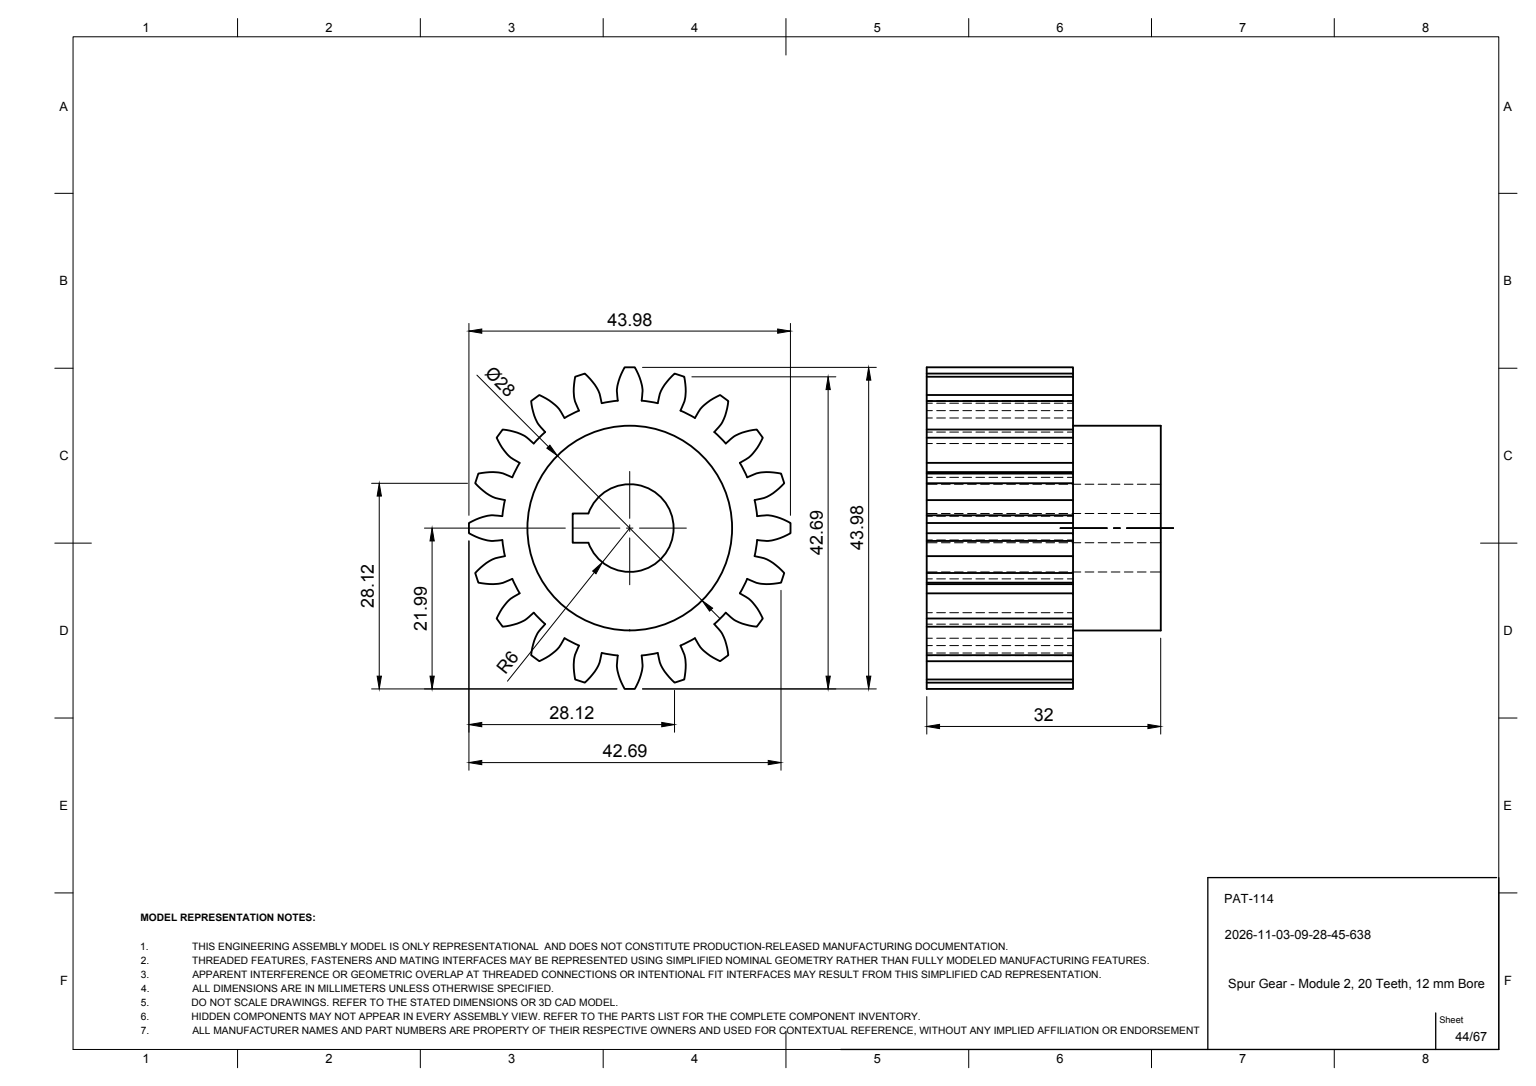
ISO-10303-21;
HEADER;
/* Generated by software containing ST-Developer
 * from STEP Tools, Inc. (www.steptools.com) 
 */

FILE_DESCRIPTION(
/* description */ ('Two-stage gear reducer in split housing'),
/* implementation_level */ '2;1');

FILE_NAME(
/* name */ 'Spur Gear - Module 2, 20 Teeth, 12 mm Bore.step',
/* time_stamp */ '2026-10-28T03:22:31-07:00',
/* author */ (''),
/* organization */ (''),
/* preprocessor_version */ 'ST-DEVELOPER v20.2',
/* originating_system */ 'Autodesk Translation Framework v15.17.0.0',
/* authorisation */ '');

FILE_SCHEMA (('AUTOMOTIVE_DESIGN { 1 0 10303 214 3 1 1 }'));
ENDSEC;

DATA;
#10=MECHANICAL_DESIGN_GEOMETRIC_PRESENTATION_REPRESENTATION('',(#1284),#73366);
#11=(
BOUNDED_SURFACE()
B_SPLINE_SURFACE(5,1,((#28644,#28645),(#28646,#28647),(#28648,#28649),(#28650,
#28651),(#28652,#28653),(#28654,#28655),(#28656,#28657),(#28658,#28659),
(#28660,#28661),(#28662,#28663),(#28664,#28665),(#28666,#28667),(#28668,
#28669),(#28670,#28671),(#28672,#28673),(#28674,#28675),(#28676,#28677),
(#28678,#28679),(#28680,#28681),(#28682,#28683),(#28684,#28685),(#28686,
#28687),(#28688,#28689),(#28690,#28691),(#28692,#28693),(#28694,#28695),
(#28696,#28697),(#28698,#28699),(#28700,#28701),(#28702,#28703),(#28704,
#28705),(#28706,#28707),(#28708,#28709),(#28710,#28711),(#28712,#28713),
(#28714,#28715),(#28716,#28717),(#28718,#28719),(#28720,#28721),(#28722,
#28723),(#28724,#28725),(#28726,#28727),(#28728,#28729),(#28730,#28731),
(#28732,#28733),(#28734,#28735),(#28736,#28737),(#28738,#28739),(#28740,
#28741),(#28742,#28743),(#28744,#28745),(#28746,#28747),(#28748,#28749),
(#28750,#28751),(#28752,#28753),(#28754,#28755),(#28756,#28757),(#28758,
#28759),(#28760,#28761),(#28762,#28763),(#28764,#28765),(#28766,#28767),
(#28768,#28769),(#28770,#28771),(#28772,#28773),(#28774,#28775),(#28776,
#28777),(#28778,#28779),(#28780,#28781),(#28782,#28783)),.UNSPECIFIED.,
 .F.,.F.,.F.)
B_SPLINE_SURFACE_WITH_KNOTS((6,1,1,1,1,1,1,1,1,1,1,1,1,1,1,1,1,1,1,1,1,
1,1,1,1,1,1,1,1,1,1,1,1,1,1,1,1,1,1,1,1,1,1,1,1,1,1,1,1,1,1,1,1,1,1,1,1,
1,1,1,1,1,1,1,1,6),(2,2),(-1.,-0.984615384615383,-0.969230769230768,-0.953846153846152,
-0.938461538461537,-0.923076923076922,-0.907692307692306,-0.892307692307691,
-0.876923076923076,-0.86153846153846,-0.846153846153845,-0.83076923076923,
-0.815384615384614,-0.799999999999999,-0.784615384615384,-0.769230769230768,
-0.753846153846153,-0.738461538461538,-0.723076923076922,-0.707692307692307,
-0.692307692307692,-0.676923076923076,-0.661538461538461,-0.646153846153846,
-0.63076923076923,-0.615384615384615,-0.6,-0.584615384615384,-0.569230769230769,
-0.553846153846154,-0.538461538461538,-0.523076923076923,-0.507692307692308,
-0.492307692307692,-0.476923076923077,-0.461538461538462,-0.446153846153846,
-0.430769230769231,-0.415384615384615,-0.4,-0.384615384615385,-0.369230769230769,
-0.353846153846154,-0.338461538461538,-0.323076923076923,-0.307692307692308,
-0.292307692307692,-0.276923076923077,-0.261538461538462,-0.246153846153846,
-0.230769230769231,-0.215384615384615,-0.2,-0.184615384615385,-0.169230769230769,
-0.153846153846154,-0.138461538461538,-0.123076923076923,-0.107692307692308,
-0.0923076923076923,-0.0769230769230769,-0.0615384615384615,-0.0461538461538462,
-0.0307692307692308,-0.0153846153846154,0.),(-1.,1.),.UNSPECIFIED.)
GEOMETRIC_REPRESENTATION_ITEM()
RATIONAL_B_SPLINE_SURFACE(((1.,1.),(1.,1.),(1.,1.),(1.,1.),(1.,1.),(1.,
1.),(1.,1.),(1.,1.),(1.,1.),(1.,1.),(1.,1.),(1.,1.),(1.,1.),(1.,1.),(1.,
1.),(1.,1.),(1.,1.),(1.,1.),(1.,1.),(1.,1.),(1.,1.),(1.,1.),(1.,1.),(1.,
1.),(1.,1.),(1.,1.),(1.,1.),(1.,1.),(1.,1.),(1.,1.),(1.,1.),(1.,1.),(1.,
1.),(1.,1.),(1.,1.),(1.,1.),(1.,1.),(1.,1.),(1.,1.),(1.,1.),(1.,1.),(1.,
1.),(1.,1.),(1.,1.),(1.,1.),(1.,1.),(1.,1.),(1.,1.),(1.,1.),(1.,1.),(1.,
1.),(1.,1.),(1.,1.),(1.,1.),(1.,1.),(1.,1.),(1.,1.),(1.,1.),(1.,1.),(1.,
1.),(1.,1.),(1.,1.),(1.,1.),(1.,1.),(1.,1.),(1.,1.),(1.,1.),(1.,1.),(1.,
1.),(1.,1.)))
REPRESENTATION_ITEM('')
SURFACE()
);
#12=(
BOUNDED_SURFACE()
B_SPLINE_SURFACE(5,1,((#28862,#28863),(#28864,#28865),(#28866,#28867),(#28868,
#28869),(#28870,#28871),(#28872,#28873),(#28874,#28875),(#28876,#28877),
(#28878,#28879),(#28880,#28881),(#28882,#28883),(#28884,#28885),(#28886,
#28887),(#28888,#28889),(#28890,#28891),(#28892,#28893),(#28894,#28895),
(#28896,#28897),(#28898,#28899),(#28900,#28901),(#28902,#28903),(#28904,
#28905),(#28906,#28907),(#28908,#28909),(#28910,#28911),(#28912,#28913),
(#28914,#28915),(#28916,#28917),(#28918,#28919),(#28920,#28921),(#28922,
#28923),(#28924,#28925),(#28926,#28927),(#28928,#28929),(#28930,#28931),
(#28932,#28933),(#28934,#28935),(#28936,#28937),(#28938,#28939),(#28940,
#28941),(#28942,#28943),(#28944,#28945),(#28946,#28947),(#28948,#28949),
(#28950,#28951),(#28952,#28953),(#28954,#28955),(#28956,#28957),(#28958,
#28959),(#28960,#28961),(#28962,#28963),(#28964,#28965),(#28966,#28967),
(#28968,#28969),(#28970,#28971),(#28972,#28973),(#28974,#28975),(#28976,
#28977),(#28978,#28979),(#28980,#28981),(#28982,#28983),(#28984,#28985),
(#28986,#28987),(#28988,#28989),(#28990,#28991),(#28992,#28993),(#28994,
#28995),(#28996,#28997),(#28998,#28999),(#29000,#29001)),.UNSPECIFIED.,
 .F.,.F.,.F.)
B_SPLINE_SURFACE_WITH_KNOTS((6,1,1,1,1,1,1,1,1,1,1,1,1,1,1,1,1,1,1,1,1,
1,1,1,1,1,1,1,1,1,1,1,1,1,1,1,1,1,1,1,1,1,1,1,1,1,1,1,1,1,1,1,1,1,1,1,1,
1,1,1,1,1,1,1,1,6),(2,2),(-1.,-0.984615384615383,-0.969230769230768,-0.953846153846152,
-0.938461538461537,-0.923076923076922,-0.907692307692306,-0.892307692307691,
-0.876923076923076,-0.86153846153846,-0.846153846153845,-0.83076923076923,
-0.815384615384614,-0.799999999999999,-0.784615384615384,-0.769230769230768,
-0.753846153846153,-0.738461538461538,-0.723076923076922,-0.707692307692307,
-0.692307692307692,-0.676923076923076,-0.661538461538461,-0.646153846153846,
-0.63076923076923,-0.615384615384615,-0.6,-0.584615384615384,-0.569230769230769,
-0.553846153846154,-0.538461538461538,-0.523076923076923,-0.507692307692308,
-0.492307692307692,-0.476923076923077,-0.461538461538462,-0.446153846153846,
-0.430769230769231,-0.415384615384615,-0.4,-0.384615384615385,-0.369230769230769,
-0.353846153846154,-0.338461538461538,-0.323076923076923,-0.307692307692308,
-0.292307692307692,-0.276923076923077,-0.261538461538462,-0.246153846153846,
-0.230769230769231,-0.215384615384615,-0.2,-0.184615384615385,-0.169230769230769,
-0.153846153846154,-0.138461538461538,-0.123076923076923,-0.107692307692308,
-0.0923076923076923,-0.0769230769230769,-0.0615384615384615,-0.0461538461538462,
-0.0307692307692308,-0.0153846153846154,0.),(-1.,1.),.UNSPECIFIED.)
GEOMETRIC_REPRESENTATION_ITEM()
RATIONAL_B_SPLINE_SURFACE(((1.,1.),(1.,1.),(1.,1.),(1.,1.),(1.,1.),(1.,
1.),(1.,1.),(1.,1.),(1.,1.),(1.,1.),(1.,1.),(1.,1.),(1.,1.),(1.,1.),(1.,
1.),(1.,1.),(1.,1.),(1.,1.),(1.,1.),(1.,1.),(1.,1.),(1.,1.),(1.,1.),(1.,
1.),(1.,1.),(1.,1.),(1.,1.),(1.,1.),(1.,1.),(1.,1.),(1.,1.),(1.,1.),(1.,
1.),(1.,1.),(1.,1.),(1.,1.),(1.,1.),(1.,1.),(1.,1.),(1.,1.),(1.,1.),(1.,
1.),(1.,1.),(1.,1.),(1.,1.),(1.,1.),(1.,1.),(1.,1.),(1.,1.),(1.,1.),(1.,
1.),(1.,1.),(1.,1.),(1.,1.),(1.,1.),(1.,1.),(1.,1.),(1.,1.),(1.,1.),(1.,
1.),(1.,1.),(1.,1.),(1.,1.),(1.,1.),(1.,1.),(1.,1.),(1.,1.),(1.,1.),(1.,
1.),(1.,1.)))
REPRESENTATION_ITEM('')
SURFACE()
);
#13=(
BOUNDED_SURFACE()
B_SPLINE_SURFACE(5,1,((#29078,#29079),(#29080,#29081),(#29082,#29083),(#29084,
#29085),(#29086,#29087),(#29088,#29089),(#29090,#29091),(#29092,#29093),
(#29094,#29095),(#29096,#29097),(#29098,#29099),(#29100,#29101),(#29102,
#29103),(#29104,#29105),(#29106,#29107),(#29108,#29109),(#29110,#29111),
(#29112,#29113),(#29114,#29115),(#29116,#29117),(#29118,#29119),(#29120,
#29121),(#29122,#29123),(#29124,#29125),(#29126,#29127),(#29128,#29129),
(#29130,#29131),(#29132,#29133),(#29134,#29135),(#29136,#29137),(#29138,
#29139),(#29140,#29141),(#29142,#29143),(#29144,#29145),(#29146,#29147),
(#29148,#29149),(#29150,#29151),(#29152,#29153),(#29154,#29155),(#29156,
#29157),(#29158,#29159),(#29160,#29161),(#29162,#29163),(#29164,#29165),
(#29166,#29167),(#29168,#29169),(#29170,#29171),(#29172,#29173),(#29174,
#29175),(#29176,#29177),(#29178,#29179),(#29180,#29181),(#29182,#29183),
(#29184,#29185),(#29186,#29187),(#29188,#29189),(#29190,#29191),(#29192,
#29193),(#29194,#29195),(#29196,#29197),(#29198,#29199),(#29200,#29201),
(#29202,#29203),(#29204,#29205),(#29206,#29207),(#29208,#29209),(#29210,
#29211),(#29212,#29213),(#29214,#29215),(#29216,#29217)),.UNSPECIFIED.,
 .F.,.F.,.F.)
B_SPLINE_SURFACE_WITH_KNOTS((6,1,1,1,1,1,1,1,1,1,1,1,1,1,1,1,1,1,1,1,1,
1,1,1,1,1,1,1,1,1,1,1,1,1,1,1,1,1,1,1,1,1,1,1,1,1,1,1,1,1,1,1,1,1,1,1,1,
1,1,1,1,1,1,1,1,6),(2,2),(-1.,-0.984615384615383,-0.969230769230768,-0.953846153846152,
-0.938461538461537,-0.923076923076922,-0.907692307692306,-0.892307692307691,
-0.876923076923076,-0.86153846153846,-0.846153846153845,-0.83076923076923,
-0.815384615384614,-0.799999999999999,-0.784615384615384,-0.769230769230768,
-0.753846153846153,-0.738461538461538,-0.723076923076922,-0.707692307692307,
-0.692307692307692,-0.676923076923076,-0.661538461538461,-0.646153846153846,
-0.63076923076923,-0.615384615384615,-0.6,-0.584615384615384,-0.569230769230769,
-0.553846153846154,-0.538461538461538,-0.523076923076923,-0.507692307692308,
-0.492307692307692,-0.476923076923077,-0.461538461538462,-0.446153846153846,
-0.430769230769231,-0.415384615384615,-0.4,-0.384615384615385,-0.369230769230769,
-0.353846153846154,-0.338461538461538,-0.323076923076923,-0.307692307692308,
-0.292307692307692,-0.276923076923077,-0.261538461538462,-0.246153846153846,
-0.230769230769231,-0.215384615384615,-0.2,-0.184615384615385,-0.169230769230769,
-0.153846153846154,-0.138461538461538,-0.123076923076923,-0.107692307692308,
-0.0923076923076923,-0.0769230769230769,-0.0615384615384615,-0.0461538461538462,
-0.0307692307692308,-0.0153846153846154,0.),(-1.,1.),.UNSPECIFIED.)
GEOMETRIC_REPRESENTATION_ITEM()
RATIONAL_B_SPLINE_SURFACE(((1.,1.),(1.,1.),(1.,1.),(1.,1.),(1.,1.),(1.,
1.),(1.,1.),(1.,1.),(1.,1.),(1.,1.),(1.,1.),(1.,1.),(1.,1.),(1.,1.),(1.,
1.),(1.,1.),(1.,1.),(1.,1.),(1.,1.),(1.,1.),(1.,1.),(1.,1.),(1.,1.),(1.,
1.),(1.,1.),(1.,1.),(1.,1.),(1.,1.),(1.,1.),(1.,1.),(1.,1.),(1.,1.),(1.,
1.),(1.,1.),(1.,1.),(1.,1.),(1.,1.),(1.,1.),(1.,1.),(1.,1.),(1.,1.),(1.,
1.),(1.,1.),(1.,1.),(1.,1.),(1.,1.),(1.,1.),(1.,1.),(1.,1.),(1.,1.),(1.,
1.),(1.,1.),(1.,1.),(1.,1.),(1.,1.),(1.,1.),(1.,1.),(1.,1.),(1.,1.),(1.,
1.),(1.,1.),(1.,1.),(1.,1.),(1.,1.),(1.,1.),(1.,1.),(1.,1.),(1.,1.),(1.,
1.),(1.,1.)))
REPRESENTATION_ITEM('')
SURFACE()
);
#14=(
BOUNDED_SURFACE()
B_SPLINE_SURFACE(5,1,((#29294,#29295),(#29296,#29297),(#29298,#29299),(#29300,
#29301),(#29302,#29303),(#29304,#29305),(#29306,#29307),(#29308,#29309),
(#29310,#29311),(#29312,#29313),(#29314,#29315),(#29316,#29317),(#29318,
#29319),(#29320,#29321),(#29322,#29323),(#29324,#29325),(#29326,#29327),
(#29328,#29329),(#29330,#29331),(#29332,#29333),(#29334,#29335),(#29336,
#29337),(#29338,#29339),(#29340,#29341),(#29342,#29343),(#29344,#29345),
(#29346,#29347),(#29348,#29349),(#29350,#29351),(#29352,#29353),(#29354,
#29355),(#29356,#29357),(#29358,#29359),(#29360,#29361),(#29362,#29363),
(#29364,#29365),(#29366,#29367),(#29368,#29369),(#29370,#29371),(#29372,
#29373),(#29374,#29375),(#29376,#29377),(#29378,#29379),(#29380,#29381),
(#29382,#29383),(#29384,#29385),(#29386,#29387),(#29388,#29389),(#29390,
#29391),(#29392,#29393),(#29394,#29395),(#29396,#29397),(#29398,#29399),
(#29400,#29401),(#29402,#29403),(#29404,#29405),(#29406,#29407),(#29408,
#29409),(#29410,#29411),(#29412,#29413),(#29414,#29415),(#29416,#29417),
(#29418,#29419),(#29420,#29421),(#29422,#29423),(#29424,#29425),(#29426,
#29427),(#29428,#29429),(#29430,#29431),(#29432,#29433)),.UNSPECIFIED.,
 .F.,.F.,.F.)
B_SPLINE_SURFACE_WITH_KNOTS((6,1,1,1,1,1,1,1,1,1,1,1,1,1,1,1,1,1,1,1,1,
1,1,1,1,1,1,1,1,1,1,1,1,1,1,1,1,1,1,1,1,1,1,1,1,1,1,1,1,1,1,1,1,1,1,1,1,
1,1,1,1,1,1,1,1,6),(2,2),(-1.,-0.984615384615383,-0.969230769230768,-0.953846153846152,
-0.938461538461537,-0.923076923076922,-0.907692307692306,-0.892307692307691,
-0.876923076923076,-0.86153846153846,-0.846153846153845,-0.83076923076923,
-0.815384615384614,-0.799999999999999,-0.784615384615384,-0.769230769230768,
-0.753846153846153,-0.738461538461538,-0.723076923076922,-0.707692307692307,
-0.692307692307692,-0.676923076923076,-0.661538461538461,-0.646153846153846,
-0.63076923076923,-0.615384615384615,-0.6,-0.584615384615384,-0.569230769230769,
-0.553846153846154,-0.538461538461538,-0.523076923076923,-0.507692307692308,
-0.492307692307692,-0.476923076923077,-0.461538461538462,-0.446153846153846,
-0.430769230769231,-0.415384615384615,-0.4,-0.384615384615385,-0.369230769230769,
-0.353846153846154,-0.338461538461538,-0.323076923076923,-0.307692307692308,
-0.292307692307692,-0.276923076923077,-0.261538461538462,-0.246153846153846,
-0.230769230769231,-0.215384615384615,-0.2,-0.184615384615385,-0.169230769230769,
-0.153846153846154,-0.138461538461538,-0.123076923076923,-0.107692307692308,
-0.0923076923076923,-0.0769230769230769,-0.0615384615384615,-0.0461538461538462,
-0.0307692307692308,-0.0153846153846154,0.),(-1.,1.),.UNSPECIFIED.)
GEOMETRIC_REPRESENTATION_ITEM()
RATIONAL_B_SPLINE_SURFACE(((1.,1.),(1.,1.),(1.,1.),(1.,1.),(1.,1.),(1.,
1.),(1.,1.),(1.,1.),(1.,1.),(1.,1.),(1.,1.),(1.,1.),(1.,1.),(1.,1.),(1.,
1.),(1.,1.),(1.,1.),(1.,1.),(1.,1.),(1.,1.),(1.,1.),(1.,1.),(1.,1.),(1.,
1.),(1.,1.),(1.,1.),(1.,1.),(1.,1.),(1.,1.),(1.,1.),(1.,1.),(1.,1.),(1.,
1.),(1.,1.),(1.,1.),(1.,1.),(1.,1.),(1.,1.),(1.,1.),(1.,1.),(1.,1.),(1.,
1.),(1.,1.),(1.,1.),(1.,1.),(1.,1.),(1.,1.),(1.,1.),(1.,1.),(1.,1.),(1.,
1.),(1.,1.),(1.,1.),(1.,1.),(1.,1.),(1.,1.),(1.,1.),(1.,1.),(1.,1.),(1.,
1.),(1.,1.),(1.,1.),(1.,1.),(1.,1.),(1.,1.),(1.,1.),(1.,1.),(1.,1.),(1.,
1.),(1.,1.)))
REPRESENTATION_ITEM('')
SURFACE()
);
#15=(
BOUNDED_SURFACE()
B_SPLINE_SURFACE(5,1,((#29510,#29511),(#29512,#29513),(#29514,#29515),(#29516,
#29517),(#29518,#29519),(#29520,#29521),(#29522,#29523),(#29524,#29525),
(#29526,#29527),(#29528,#29529),(#29530,#29531),(#29532,#29533),(#29534,
#29535),(#29536,#29537),(#29538,#29539),(#29540,#29541),(#29542,#29543),
(#29544,#29545),(#29546,#29547),(#29548,#29549),(#29550,#29551),(#29552,
#29553),(#29554,#29555),(#29556,#29557),(#29558,#29559),(#29560,#29561),
(#29562,#29563),(#29564,#29565),(#29566,#29567),(#29568,#29569),(#29570,
#29571),(#29572,#29573),(#29574,#29575),(#29576,#29577),(#29578,#29579),
(#29580,#29581),(#29582,#29583),(#29584,#29585),(#29586,#29587),(#29588,
#29589),(#29590,#29591),(#29592,#29593),(#29594,#29595),(#29596,#29597),
(#29598,#29599),(#29600,#29601),(#29602,#29603),(#29604,#29605),(#29606,
#29607),(#29608,#29609),(#29610,#29611),(#29612,#29613),(#29614,#29615),
(#29616,#29617),(#29618,#29619),(#29620,#29621),(#29622,#29623),(#29624,
#29625),(#29626,#29627),(#29628,#29629),(#29630,#29631),(#29632,#29633),
(#29634,#29635),(#29636,#29637),(#29638,#29639),(#29640,#29641),(#29642,
#29643),(#29644,#29645),(#29646,#29647),(#29648,#29649)),.UNSPECIFIED.,
 .F.,.F.,.F.)
B_SPLINE_SURFACE_WITH_KNOTS((6,1,1,1,1,1,1,1,1,1,1,1,1,1,1,1,1,1,1,1,1,
1,1,1,1,1,1,1,1,1,1,1,1,1,1,1,1,1,1,1,1,1,1,1,1,1,1,1,1,1,1,1,1,1,1,1,1,
1,1,1,1,1,1,1,1,6),(2,2),(-1.,-0.984615384615383,-0.969230769230768,-0.953846153846152,
-0.938461538461537,-0.923076923076922,-0.907692307692306,-0.892307692307691,
-0.876923076923076,-0.86153846153846,-0.846153846153845,-0.83076923076923,
-0.815384615384614,-0.799999999999999,-0.784615384615384,-0.769230769230768,
-0.753846153846153,-0.738461538461538,-0.723076923076922,-0.707692307692307,
-0.692307692307692,-0.676923076923076,-0.661538461538461,-0.646153846153846,
-0.63076923076923,-0.615384615384615,-0.6,-0.584615384615384,-0.569230769230769,
-0.553846153846154,-0.538461538461538,-0.523076923076923,-0.507692307692308,
-0.492307692307692,-0.476923076923077,-0.461538461538462,-0.446153846153846,
-0.430769230769231,-0.415384615384615,-0.4,-0.384615384615385,-0.369230769230769,
-0.353846153846154,-0.338461538461538,-0.323076923076923,-0.307692307692308,
-0.292307692307692,-0.276923076923077,-0.261538461538462,-0.246153846153846,
-0.230769230769231,-0.215384615384615,-0.2,-0.184615384615385,-0.169230769230769,
-0.153846153846154,-0.138461538461538,-0.123076923076923,-0.107692307692308,
-0.0923076923076923,-0.0769230769230769,-0.0615384615384615,-0.0461538461538462,
-0.0307692307692308,-0.0153846153846154,0.),(-1.,1.),.UNSPECIFIED.)
GEOMETRIC_REPRESENTATION_ITEM()
RATIONAL_B_SPLINE_SURFACE(((1.,1.),(1.,1.),(1.,1.),(1.,1.),(1.,1.),(1.,
1.),(1.,1.),(1.,1.),(1.,1.),(1.,1.),(1.,1.),(1.,1.),(1.,1.),(1.,1.),(1.,
1.),(1.,1.),(1.,1.),(1.,1.),(1.,1.),(1.,1.),(1.,1.),(1.,1.),(1.,1.),(1.,
1.),(1.,1.),(1.,1.),(1.,1.),(1.,1.),(1.,1.),(1.,1.),(1.,1.),(1.,1.),(1.,
1.),(1.,1.),(1.,1.),(1.,1.),(1.,1.),(1.,1.),(1.,1.),(1.,1.),(1.,1.),(1.,
1.),(1.,1.),(1.,1.),(1.,1.),(1.,1.),(1.,1.),(1.,1.),(1.,1.),(1.,1.),(1.,
1.),(1.,1.),(1.,1.),(1.,1.),(1.,1.),(1.,1.),(1.,1.),(1.,1.),(1.,1.),(1.,
1.),(1.,1.),(1.,1.),(1.,1.),(1.,1.),(1.,1.),(1.,1.),(1.,1.),(1.,1.),(1.,
1.),(1.,1.)))
REPRESENTATION_ITEM('')
SURFACE()
);
#16=(
BOUNDED_SURFACE()
B_SPLINE_SURFACE(5,1,((#29726,#29727),(#29728,#29729),(#29730,#29731),(#29732,
#29733),(#29734,#29735),(#29736,#29737),(#29738,#29739),(#29740,#29741),
(#29742,#29743),(#29744,#29745),(#29746,#29747),(#29748,#29749),(#29750,
#29751),(#29752,#29753),(#29754,#29755),(#29756,#29757),(#29758,#29759),
(#29760,#29761),(#29762,#29763),(#29764,#29765),(#29766,#29767),(#29768,
#29769),(#29770,#29771),(#29772,#29773),(#29774,#29775),(#29776,#29777),
(#29778,#29779),(#29780,#29781),(#29782,#29783),(#29784,#29785),(#29786,
#29787),(#29788,#29789),(#29790,#29791),(#29792,#29793),(#29794,#29795),
(#29796,#29797),(#29798,#29799),(#29800,#29801),(#29802,#29803),(#29804,
#29805),(#29806,#29807),(#29808,#29809),(#29810,#29811),(#29812,#29813),
(#29814,#29815),(#29816,#29817),(#29818,#29819),(#29820,#29821),(#29822,
#29823),(#29824,#29825),(#29826,#29827),(#29828,#29829),(#29830,#29831),
(#29832,#29833),(#29834,#29835),(#29836,#29837),(#29838,#29839),(#29840,
#29841),(#29842,#29843),(#29844,#29845),(#29846,#29847),(#29848,#29849),
(#29850,#29851),(#29852,#29853),(#29854,#29855),(#29856,#29857),(#29858,
#29859),(#29860,#29861),(#29862,#29863),(#29864,#29865)),.UNSPECIFIED.,
 .F.,.F.,.F.)
B_SPLINE_SURFACE_WITH_KNOTS((6,1,1,1,1,1,1,1,1,1,1,1,1,1,1,1,1,1,1,1,1,
1,1,1,1,1,1,1,1,1,1,1,1,1,1,1,1,1,1,1,1,1,1,1,1,1,1,1,1,1,1,1,1,1,1,1,1,
1,1,1,1,1,1,1,1,6),(2,2),(-1.,-0.984615384615383,-0.969230769230768,-0.953846153846152,
-0.938461538461537,-0.923076923076922,-0.907692307692306,-0.892307692307691,
-0.876923076923076,-0.86153846153846,-0.846153846153845,-0.83076923076923,
-0.815384615384614,-0.799999999999999,-0.784615384615384,-0.769230769230768,
-0.753846153846153,-0.738461538461538,-0.723076923076922,-0.707692307692307,
-0.692307692307692,-0.676923076923076,-0.661538461538461,-0.646153846153846,
-0.63076923076923,-0.615384615384615,-0.6,-0.584615384615384,-0.569230769230769,
-0.553846153846154,-0.538461538461538,-0.523076923076923,-0.507692307692308,
-0.492307692307692,-0.476923076923077,-0.461538461538462,-0.446153846153846,
-0.430769230769231,-0.415384615384615,-0.4,-0.384615384615385,-0.369230769230769,
-0.353846153846154,-0.338461538461538,-0.323076923076923,-0.307692307692308,
-0.292307692307692,-0.276923076923077,-0.261538461538462,-0.246153846153846,
-0.230769230769231,-0.215384615384615,-0.2,-0.184615384615385,-0.169230769230769,
-0.153846153846154,-0.138461538461538,-0.123076923076923,-0.107692307692308,
-0.0923076923076923,-0.0769230769230769,-0.0615384615384615,-0.0461538461538462,
-0.0307692307692308,-0.0153846153846154,0.),(-1.,1.),.UNSPECIFIED.)
GEOMETRIC_REPRESENTATION_ITEM()
RATIONAL_B_SPLINE_SURFACE(((1.,1.),(1.,1.),(1.,1.),(1.,1.),(1.,1.),(1.,
1.),(1.,1.),(1.,1.),(1.,1.),(1.,1.),(1.,1.),(1.,1.),(1.,1.),(1.,1.),(1.,
1.),(1.,1.),(1.,1.),(1.,1.),(1.,1.),(1.,1.),(1.,1.),(1.,1.),(1.,1.),(1.,
1.),(1.,1.),(1.,1.),(1.,1.),(1.,1.),(1.,1.),(1.,1.),(1.,1.),(1.,1.),(1.,
1.),(1.,1.),(1.,1.),(1.,1.),(1.,1.),(1.,1.),(1.,1.),(1.,1.),(1.,1.),(1.,
1.),(1.,1.),(1.,1.),(1.,1.),(1.,1.),(1.,1.),(1.,1.),(1.,1.),(1.,1.),(1.,
1.),(1.,1.),(1.,1.),(1.,1.),(1.,1.),(1.,1.),(1.,1.),(1.,1.),(1.,1.),(1.,
1.),(1.,1.),(1.,1.),(1.,1.),(1.,1.),(1.,1.),(1.,1.),(1.,1.),(1.,1.),(1.,
1.),(1.,1.)))
REPRESENTATION_ITEM('')
SURFACE()
);
#17=(
BOUNDED_SURFACE()
B_SPLINE_SURFACE(5,1,((#29942,#29943),(#29944,#29945),(#29946,#29947),(#29948,
#29949),(#29950,#29951),(#29952,#29953),(#29954,#29955),(#29956,#29957),
(#29958,#29959),(#29960,#29961),(#29962,#29963),(#29964,#29965),(#29966,
#29967),(#29968,#29969),(#29970,#29971),(#29972,#29973),(#29974,#29975),
(#29976,#29977),(#29978,#29979),(#29980,#29981),(#29982,#29983),(#29984,
#29985),(#29986,#29987),(#29988,#29989),(#29990,#29991),(#29992,#29993),
(#29994,#29995),(#29996,#29997),(#29998,#29999),(#30000,#30001),(#30002,
#30003),(#30004,#30005),(#30006,#30007),(#30008,#30009),(#30010,#30011),
(#30012,#30013),(#30014,#30015),(#30016,#30017),(#30018,#30019),(#30020,
#30021),(#30022,#30023),(#30024,#30025),(#30026,#30027),(#30028,#30029),
(#30030,#30031),(#30032,#30033),(#30034,#30035),(#30036,#30037),(#30038,
#30039),(#30040,#30041),(#30042,#30043),(#30044,#30045),(#30046,#30047),
(#30048,#30049),(#30050,#30051),(#30052,#30053),(#30054,#30055),(#30056,
#30057),(#30058,#30059),(#30060,#30061),(#30062,#30063),(#30064,#30065),
(#30066,#30067),(#30068,#30069),(#30070,#30071),(#30072,#30073),(#30074,
#30075),(#30076,#30077),(#30078,#30079),(#30080,#30081)),.UNSPECIFIED.,
 .F.,.F.,.F.)
B_SPLINE_SURFACE_WITH_KNOTS((6,1,1,1,1,1,1,1,1,1,1,1,1,1,1,1,1,1,1,1,1,
1,1,1,1,1,1,1,1,1,1,1,1,1,1,1,1,1,1,1,1,1,1,1,1,1,1,1,1,1,1,1,1,1,1,1,1,
1,1,1,1,1,1,1,1,6),(2,2),(-1.,-0.984615384615383,-0.969230769230768,-0.953846153846152,
-0.938461538461537,-0.923076923076922,-0.907692307692306,-0.892307692307691,
-0.876923076923076,-0.86153846153846,-0.846153846153845,-0.83076923076923,
-0.815384615384614,-0.799999999999999,-0.784615384615384,-0.769230769230768,
-0.753846153846153,-0.738461538461538,-0.723076923076922,-0.707692307692307,
-0.692307692307692,-0.676923076923076,-0.661538461538461,-0.646153846153846,
-0.63076923076923,-0.615384615384615,-0.6,-0.584615384615384,-0.569230769230769,
-0.553846153846154,-0.538461538461538,-0.523076923076923,-0.507692307692308,
-0.492307692307692,-0.476923076923077,-0.461538461538462,-0.446153846153846,
-0.430769230769231,-0.415384615384615,-0.4,-0.384615384615385,-0.369230769230769,
-0.353846153846154,-0.338461538461538,-0.323076923076923,-0.307692307692308,
-0.292307692307692,-0.276923076923077,-0.261538461538462,-0.246153846153846,
-0.230769230769231,-0.215384615384615,-0.2,-0.184615384615385,-0.169230769230769,
-0.153846153846154,-0.138461538461538,-0.123076923076923,-0.107692307692308,
-0.0923076923076923,-0.0769230769230769,-0.0615384615384615,-0.0461538461538462,
-0.0307692307692308,-0.0153846153846154,0.),(-1.,1.),.UNSPECIFIED.)
GEOMETRIC_REPRESENTATION_ITEM()
RATIONAL_B_SPLINE_SURFACE(((1.,1.),(1.,1.),(1.,1.),(1.,1.),(1.,1.),(1.,
1.),(1.,1.),(1.,1.),(1.,1.),(1.,1.),(1.,1.),(1.,1.),(1.,1.),(1.,1.),(1.,
1.),(1.,1.),(1.,1.),(1.,1.),(1.,1.),(1.,1.),(1.,1.),(1.,1.),(1.,1.),(1.,
1.),(1.,1.),(1.,1.),(1.,1.),(1.,1.),(1.,1.),(1.,1.),(1.,1.),(1.,1.),(1.,
1.),(1.,1.),(1.,1.),(1.,1.),(1.,1.),(1.,1.),(1.,1.),(1.,1.),(1.,1.),(1.,
1.),(1.,1.),(1.,1.),(1.,1.),(1.,1.),(1.,1.),(1.,1.),(1.,1.),(1.,1.),(1.,
1.),(1.,1.),(1.,1.),(1.,1.),(1.,1.),(1.,1.),(1.,1.),(1.,1.),(1.,1.),(1.,
1.),(1.,1.),(1.,1.),(1.,1.),(1.,1.),(1.,1.),(1.,1.),(1.,1.),(1.,1.),(1.,
1.),(1.,1.)))
REPRESENTATION_ITEM('')
SURFACE()
);
#18=(
BOUNDED_SURFACE()
B_SPLINE_SURFACE(5,1,((#30158,#30159),(#30160,#30161),(#30162,#30163),(#30164,
#30165),(#30166,#30167),(#30168,#30169),(#30170,#30171),(#30172,#30173),
(#30174,#30175),(#30176,#30177),(#30178,#30179),(#30180,#30181),(#30182,
#30183),(#30184,#30185),(#30186,#30187),(#30188,#30189),(#30190,#30191),
(#30192,#30193),(#30194,#30195),(#30196,#30197),(#30198,#30199),(#30200,
#30201),(#30202,#30203),(#30204,#30205),(#30206,#30207),(#30208,#30209),
(#30210,#30211),(#30212,#30213),(#30214,#30215),(#30216,#30217),(#30218,
#30219),(#30220,#30221),(#30222,#30223),(#30224,#30225),(#30226,#30227),
(#30228,#30229),(#30230,#30231),(#30232,#30233),(#30234,#30235),(#30236,
#30237),(#30238,#30239),(#30240,#30241),(#30242,#30243),(#30244,#30245),
(#30246,#30247),(#30248,#30249),(#30250,#30251),(#30252,#30253),(#30254,
#30255),(#30256,#30257),(#30258,#30259),(#30260,#30261),(#30262,#30263),
(#30264,#30265),(#30266,#30267),(#30268,#30269),(#30270,#30271),(#30272,
#30273),(#30274,#30275),(#30276,#30277),(#30278,#30279),(#30280,#30281),
(#30282,#30283),(#30284,#30285),(#30286,#30287),(#30288,#30289),(#30290,
#30291),(#30292,#30293),(#30294,#30295),(#30296,#30297)),.UNSPECIFIED.,
 .F.,.F.,.F.)
B_SPLINE_SURFACE_WITH_KNOTS((6,1,1,1,1,1,1,1,1,1,1,1,1,1,1,1,1,1,1,1,1,
1,1,1,1,1,1,1,1,1,1,1,1,1,1,1,1,1,1,1,1,1,1,1,1,1,1,1,1,1,1,1,1,1,1,1,1,
1,1,1,1,1,1,1,1,6),(2,2),(-1.,-0.984615384615383,-0.969230769230768,-0.953846153846152,
-0.938461538461537,-0.923076923076922,-0.907692307692306,-0.892307692307691,
-0.876923076923076,-0.86153846153846,-0.846153846153845,-0.83076923076923,
-0.815384615384614,-0.799999999999999,-0.784615384615384,-0.769230769230768,
-0.753846153846153,-0.738461538461538,-0.723076923076922,-0.707692307692307,
-0.692307692307692,-0.676923076923076,-0.661538461538461,-0.646153846153846,
-0.63076923076923,-0.615384615384615,-0.6,-0.584615384615384,-0.569230769230769,
-0.553846153846154,-0.538461538461538,-0.523076923076923,-0.507692307692308,
-0.492307692307692,-0.476923076923077,-0.461538461538462,-0.446153846153846,
-0.430769230769231,-0.415384615384615,-0.4,-0.384615384615385,-0.369230769230769,
-0.353846153846154,-0.338461538461538,-0.323076923076923,-0.307692307692308,
-0.292307692307692,-0.276923076923077,-0.261538461538462,-0.246153846153846,
-0.230769230769231,-0.215384615384615,-0.2,-0.184615384615385,-0.169230769230769,
-0.153846153846154,-0.138461538461538,-0.123076923076923,-0.107692307692308,
-0.0923076923076923,-0.0769230769230769,-0.0615384615384615,-0.0461538461538462,
-0.0307692307692308,-0.0153846153846154,0.),(-1.,1.),.UNSPECIFIED.)
GEOMETRIC_REPRESENTATION_ITEM()
RATIONAL_B_SPLINE_SURFACE(((1.,1.),(1.,1.),(1.,1.),(1.,1.),(1.,1.),(1.,
1.),(1.,1.),(1.,1.),(1.,1.),(1.,1.),(1.,1.),(1.,1.),(1.,1.),(1.,1.),(1.,
1.),(1.,1.),(1.,1.),(1.,1.),(1.,1.),(1.,1.),(1.,1.),(1.,1.),(1.,1.),(1.,
1.),(1.,1.),(1.,1.),(1.,1.),(1.,1.),(1.,1.),(1.,1.),(1.,1.),(1.,1.),(1.,
1.),(1.,1.),(1.,1.),(1.,1.),(1.,1.),(1.,1.),(1.,1.),(1.,1.),(1.,1.),(1.,
1.),(1.,1.),(1.,1.),(1.,1.),(1.,1.),(1.,1.),(1.,1.),(1.,1.),(1.,1.),(1.,
1.),(1.,1.),(1.,1.),(1.,1.),(1.,1.),(1.,1.),(1.,1.),(1.,1.),(1.,1.),(1.,
1.),(1.,1.),(1.,1.),(1.,1.),(1.,1.),(1.,1.),(1.,1.),(1.,1.),(1.,1.),(1.,
1.),(1.,1.)))
REPRESENTATION_ITEM('')
SURFACE()
);
#19=(
BOUNDED_SURFACE()
B_SPLINE_SURFACE(5,1,((#30374,#30375),(#30376,#30377),(#30378,#30379),(#30380,
#30381),(#30382,#30383),(#30384,#30385),(#30386,#30387),(#30388,#30389),
(#30390,#30391),(#30392,#30393),(#30394,#30395),(#30396,#30397),(#30398,
#30399),(#30400,#30401),(#30402,#30403),(#30404,#30405),(#30406,#30407),
(#30408,#30409),(#30410,#30411),(#30412,#30413),(#30414,#30415),(#30416,
#30417),(#30418,#30419),(#30420,#30421),(#30422,#30423),(#30424,#30425),
(#30426,#30427),(#30428,#30429),(#30430,#30431),(#30432,#30433),(#30434,
#30435),(#30436,#30437),(#30438,#30439),(#30440,#30441),(#30442,#30443),
(#30444,#30445),(#30446,#30447),(#30448,#30449),(#30450,#30451),(#30452,
#30453),(#30454,#30455),(#30456,#30457),(#30458,#30459),(#30460,#30461),
(#30462,#30463),(#30464,#30465),(#30466,#30467),(#30468,#30469),(#30470,
#30471),(#30472,#30473),(#30474,#30475),(#30476,#30477),(#30478,#30479),
(#30480,#30481),(#30482,#30483),(#30484,#30485),(#30486,#30487),(#30488,
#30489),(#30490,#30491),(#30492,#30493),(#30494,#30495),(#30496,#30497),
(#30498,#30499),(#30500,#30501),(#30502,#30503),(#30504,#30505),(#30506,
#30507),(#30508,#30509),(#30510,#30511),(#30512,#30513)),.UNSPECIFIED.,
 .F.,.F.,.F.)
B_SPLINE_SURFACE_WITH_KNOTS((6,1,1,1,1,1,1,1,1,1,1,1,1,1,1,1,1,1,1,1,1,
1,1,1,1,1,1,1,1,1,1,1,1,1,1,1,1,1,1,1,1,1,1,1,1,1,1,1,1,1,1,1,1,1,1,1,1,
1,1,1,1,1,1,1,1,6),(2,2),(-1.,-0.984615384615383,-0.969230769230768,-0.953846153846152,
-0.938461538461537,-0.923076923076922,-0.907692307692306,-0.892307692307691,
-0.876923076923076,-0.86153846153846,-0.846153846153845,-0.83076923076923,
-0.815384615384614,-0.799999999999999,-0.784615384615384,-0.769230769230768,
-0.753846153846153,-0.738461538461538,-0.723076923076922,-0.707692307692307,
-0.692307692307692,-0.676923076923076,-0.661538461538461,-0.646153846153846,
-0.63076923076923,-0.615384615384615,-0.6,-0.584615384615384,-0.569230769230769,
-0.553846153846154,-0.538461538461538,-0.523076923076923,-0.507692307692308,
-0.492307692307692,-0.476923076923077,-0.461538461538462,-0.446153846153846,
-0.430769230769231,-0.415384615384615,-0.4,-0.384615384615385,-0.369230769230769,
-0.353846153846154,-0.338461538461538,-0.323076923076923,-0.307692307692308,
-0.292307692307692,-0.276923076923077,-0.261538461538462,-0.246153846153846,
-0.230769230769231,-0.215384615384615,-0.2,-0.184615384615385,-0.169230769230769,
-0.153846153846154,-0.138461538461538,-0.123076923076923,-0.107692307692308,
-0.0923076923076923,-0.0769230769230769,-0.0615384615384615,-0.0461538461538462,
-0.0307692307692308,-0.0153846153846154,0.),(-1.,1.),.UNSPECIFIED.)
GEOMETRIC_REPRESENTATION_ITEM()
RATIONAL_B_SPLINE_SURFACE(((1.,1.),(1.,1.),(1.,1.),(1.,1.),(1.,1.),(1.,
1.),(1.,1.),(1.,1.),(1.,1.),(1.,1.),(1.,1.),(1.,1.),(1.,1.),(1.,1.),(1.,
1.),(1.,1.),(1.,1.),(1.,1.),(1.,1.),(1.,1.),(1.,1.),(1.,1.),(1.,1.),(1.,
1.),(1.,1.),(1.,1.),(1.,1.),(1.,1.),(1.,1.),(1.,1.),(1.,1.),(1.,1.),(1.,
1.),(1.,1.),(1.,1.),(1.,1.),(1.,1.),(1.,1.),(1.,1.),(1.,1.),(1.,1.),(1.,
1.),(1.,1.),(1.,1.),(1.,1.),(1.,1.),(1.,1.),(1.,1.),(1.,1.),(1.,1.),(1.,
1.),(1.,1.),(1.,1.),(1.,1.),(1.,1.),(1.,1.),(1.,1.),(1.,1.),(1.,1.),(1.,
1.),(1.,1.),(1.,1.),(1.,1.),(1.,1.),(1.,1.),(1.,1.),(1.,1.),(1.,1.),(1.,
1.),(1.,1.)))
REPRESENTATION_ITEM('')
SURFACE()
);
#20=(
BOUNDED_SURFACE()
B_SPLINE_SURFACE(5,1,((#30590,#30591),(#30592,#30593),(#30594,#30595),(#30596,
#30597),(#30598,#30599),(#30600,#30601),(#30602,#30603),(#30604,#30605),
(#30606,#30607),(#30608,#30609),(#30610,#30611),(#30612,#30613),(#30614,
#30615),(#30616,#30617),(#30618,#30619),(#30620,#30621),(#30622,#30623),
(#30624,#30625),(#30626,#30627),(#30628,#30629),(#30630,#30631),(#30632,
#30633),(#30634,#30635),(#30636,#30637),(#30638,#30639),(#30640,#30641),
(#30642,#30643),(#30644,#30645),(#30646,#30647),(#30648,#30649),(#30650,
#30651),(#30652,#30653),(#30654,#30655),(#30656,#30657),(#30658,#30659),
(#30660,#30661),(#30662,#30663),(#30664,#30665),(#30666,#30667),(#30668,
#30669),(#30670,#30671),(#30672,#30673),(#30674,#30675),(#30676,#30677),
(#30678,#30679),(#30680,#30681),(#30682,#30683),(#30684,#30685),(#30686,
#30687),(#30688,#30689),(#30690,#30691),(#30692,#30693),(#30694,#30695),
(#30696,#30697),(#30698,#30699),(#30700,#30701),(#30702,#30703),(#30704,
#30705),(#30706,#30707),(#30708,#30709),(#30710,#30711),(#30712,#30713),
(#30714,#30715),(#30716,#30717),(#30718,#30719),(#30720,#30721),(#30722,
#30723),(#30724,#30725),(#30726,#30727),(#30728,#30729)),.UNSPECIFIED.,
 .F.,.F.,.F.)
B_SPLINE_SURFACE_WITH_KNOTS((6,1,1,1,1,1,1,1,1,1,1,1,1,1,1,1,1,1,1,1,1,
1,1,1,1,1,1,1,1,1,1,1,1,1,1,1,1,1,1,1,1,1,1,1,1,1,1,1,1,1,1,1,1,1,1,1,1,
1,1,1,1,1,1,1,1,6),(2,2),(-1.,-0.984615384615383,-0.969230769230768,-0.953846153846152,
-0.938461538461537,-0.923076923076922,-0.907692307692306,-0.892307692307691,
-0.876923076923076,-0.86153846153846,-0.846153846153845,-0.83076923076923,
-0.815384615384614,-0.799999999999999,-0.784615384615384,-0.769230769230768,
-0.753846153846153,-0.738461538461538,-0.723076923076922,-0.707692307692307,
-0.692307692307692,-0.676923076923076,-0.661538461538461,-0.646153846153846,
-0.63076923076923,-0.615384615384615,-0.6,-0.584615384615384,-0.569230769230769,
-0.553846153846154,-0.538461538461538,-0.523076923076923,-0.507692307692308,
-0.492307692307692,-0.476923076923077,-0.461538461538462,-0.446153846153846,
-0.430769230769231,-0.415384615384615,-0.4,-0.384615384615385,-0.369230769230769,
-0.353846153846154,-0.338461538461538,-0.323076923076923,-0.307692307692308,
-0.292307692307692,-0.276923076923077,-0.261538461538462,-0.246153846153846,
-0.230769230769231,-0.215384615384615,-0.2,-0.184615384615385,-0.169230769230769,
-0.153846153846154,-0.138461538461538,-0.123076923076923,-0.107692307692308,
-0.0923076923076923,-0.0769230769230769,-0.0615384615384615,-0.0461538461538462,
-0.0307692307692308,-0.0153846153846154,0.),(-1.,1.),.UNSPECIFIED.)
GEOMETRIC_REPRESENTATION_ITEM()
RATIONAL_B_SPLINE_SURFACE(((1.,1.),(1.,1.),(1.,1.),(1.,1.),(1.,1.),(1.,
1.),(1.,1.),(1.,1.),(1.,1.),(1.,1.),(1.,1.),(1.,1.),(1.,1.),(1.,1.),(1.,
1.),(1.,1.),(1.,1.),(1.,1.),(1.,1.),(1.,1.),(1.,1.),(1.,1.),(1.,1.),(1.,
1.),(1.,1.),(1.,1.),(1.,1.),(1.,1.),(1.,1.),(1.,1.),(1.,1.),(1.,1.),(1.,
1.),(1.,1.),(1.,1.),(1.,1.),(1.,1.),(1.,1.),(1.,1.),(1.,1.),(1.,1.),(1.,
1.),(1.,1.),(1.,1.),(1.,1.),(1.,1.),(1.,1.),(1.,1.),(1.,1.),(1.,1.),(1.,
1.),(1.,1.),(1.,1.),(1.,1.),(1.,1.),(1.,1.),(1.,1.),(1.,1.),(1.,1.),(1.,
1.),(1.,1.),(1.,1.),(1.,1.),(1.,1.),(1.,1.),(1.,1.),(1.,1.),(1.,1.),(1.,
1.),(1.,1.)))
REPRESENTATION_ITEM('')
SURFACE()
);
#21=(
BOUNDED_SURFACE()
B_SPLINE_SURFACE(5,1,((#30806,#30807),(#30808,#30809),(#30810,#30811),(#30812,
#30813),(#30814,#30815),(#30816,#30817),(#30818,#30819),(#30820,#30821),
(#30822,#30823),(#30824,#30825),(#30826,#30827),(#30828,#30829),(#30830,
#30831),(#30832,#30833),(#30834,#30835),(#30836,#30837),(#30838,#30839),
(#30840,#30841),(#30842,#30843),(#30844,#30845),(#30846,#30847),(#30848,
#30849),(#30850,#30851),(#30852,#30853),(#30854,#30855),(#30856,#30857),
(#30858,#30859),(#30860,#30861),(#30862,#30863),(#30864,#30865),(#30866,
#30867),(#30868,#30869),(#30870,#30871),(#30872,#30873),(#30874,#30875),
(#30876,#30877),(#30878,#30879),(#30880,#30881),(#30882,#30883),(#30884,
#30885),(#30886,#30887),(#30888,#30889),(#30890,#30891),(#30892,#30893),
(#30894,#30895),(#30896,#30897),(#30898,#30899),(#30900,#30901),(#30902,
#30903),(#30904,#30905),(#30906,#30907),(#30908,#30909),(#30910,#30911),
(#30912,#30913),(#30914,#30915),(#30916,#30917),(#30918,#30919),(#30920,
#30921),(#30922,#30923),(#30924,#30925),(#30926,#30927),(#30928,#30929),
(#30930,#30931),(#30932,#30933),(#30934,#30935),(#30936,#30937),(#30938,
#30939),(#30940,#30941),(#30942,#30943),(#30944,#30945)),.UNSPECIFIED.,
 .F.,.F.,.F.)
B_SPLINE_SURFACE_WITH_KNOTS((6,1,1,1,1,1,1,1,1,1,1,1,1,1,1,1,1,1,1,1,1,
1,1,1,1,1,1,1,1,1,1,1,1,1,1,1,1,1,1,1,1,1,1,1,1,1,1,1,1,1,1,1,1,1,1,1,1,
1,1,1,1,1,1,1,1,6),(2,2),(-1.,-0.984615384615383,-0.969230769230768,-0.953846153846152,
-0.938461538461537,-0.923076923076922,-0.907692307692306,-0.892307692307691,
-0.876923076923076,-0.86153846153846,-0.846153846153845,-0.83076923076923,
-0.815384615384614,-0.799999999999999,-0.784615384615384,-0.769230769230768,
-0.753846153846153,-0.738461538461538,-0.723076923076922,-0.707692307692307,
-0.692307692307692,-0.676923076923076,-0.661538461538461,-0.646153846153846,
-0.63076923076923,-0.615384615384615,-0.6,-0.584615384615384,-0.569230769230769,
-0.553846153846154,-0.538461538461538,-0.523076923076923,-0.507692307692308,
-0.492307692307692,-0.476923076923077,-0.461538461538462,-0.446153846153846,
-0.430769230769231,-0.415384615384615,-0.4,-0.384615384615385,-0.369230769230769,
-0.353846153846154,-0.338461538461538,-0.323076923076923,-0.307692307692308,
-0.292307692307692,-0.276923076923077,-0.261538461538462,-0.246153846153846,
-0.230769230769231,-0.215384615384615,-0.2,-0.184615384615385,-0.169230769230769,
-0.153846153846154,-0.138461538461538,-0.123076923076923,-0.107692307692308,
-0.0923076923076923,-0.0769230769230769,-0.0615384615384615,-0.0461538461538462,
-0.0307692307692308,-0.0153846153846154,0.),(-1.,1.),.UNSPECIFIED.)
GEOMETRIC_REPRESENTATION_ITEM()
RATIONAL_B_SPLINE_SURFACE(((1.,1.),(1.,1.),(1.,1.),(1.,1.),(1.,1.),(1.,
1.),(1.,1.),(1.,1.),(1.,1.),(1.,1.),(1.,1.),(1.,1.),(1.,1.),(1.,1.),(1.,
1.),(1.,1.),(1.,1.),(1.,1.),(1.,1.),(1.,1.),(1.,1.),(1.,1.),(1.,1.),(1.,
1.),(1.,1.),(1.,1.),(1.,1.),(1.,1.),(1.,1.),(1.,1.),(1.,1.),(1.,1.),(1.,
1.),(1.,1.),(1.,1.),(1.,1.),(1.,1.),(1.,1.),(1.,1.),(1.,1.),(1.,1.),(1.,
1.),(1.,1.),(1.,1.),(1.,1.),(1.,1.),(1.,1.),(1.,1.),(1.,1.),(1.,1.),(1.,
1.),(1.,1.),(1.,1.),(1.,1.),(1.,1.),(1.,1.),(1.,1.),(1.,1.),(1.,1.),(1.,
1.),(1.,1.),(1.,1.),(1.,1.),(1.,1.),(1.,1.),(1.,1.),(1.,1.),(1.,1.),(1.,
1.),(1.,1.)))
REPRESENTATION_ITEM('')
SURFACE()
);
#22=(
BOUNDED_SURFACE()
B_SPLINE_SURFACE(5,1,((#31022,#31023),(#31024,#31025),(#31026,#31027),(#31028,
#31029),(#31030,#31031),(#31032,#31033),(#31034,#31035),(#31036,#31037),
(#31038,#31039),(#31040,#31041),(#31042,#31043),(#31044,#31045),(#31046,
#31047),(#31048,#31049),(#31050,#31051),(#31052,#31053),(#31054,#31055),
(#31056,#31057),(#31058,#31059),(#31060,#31061),(#31062,#31063),(#31064,
#31065),(#31066,#31067),(#31068,#31069),(#31070,#31071),(#31072,#31073),
(#31074,#31075),(#31076,#31077),(#31078,#31079),(#31080,#31081),(#31082,
#31083),(#31084,#31085),(#31086,#31087),(#31088,#31089),(#31090,#31091),
(#31092,#31093),(#31094,#31095),(#31096,#31097),(#31098,#31099),(#31100,
#31101),(#31102,#31103),(#31104,#31105),(#31106,#31107),(#31108,#31109),
(#31110,#31111),(#31112,#31113),(#31114,#31115),(#31116,#31117),(#31118,
#31119),(#31120,#31121),(#31122,#31123),(#31124,#31125),(#31126,#31127),
(#31128,#31129),(#31130,#31131),(#31132,#31133),(#31134,#31135),(#31136,
#31137),(#31138,#31139),(#31140,#31141),(#31142,#31143),(#31144,#31145),
(#31146,#31147),(#31148,#31149),(#31150,#31151),(#31152,#31153),(#31154,
#31155),(#31156,#31157),(#31158,#31159),(#31160,#31161)),.UNSPECIFIED.,
 .F.,.F.,.F.)
B_SPLINE_SURFACE_WITH_KNOTS((6,1,1,1,1,1,1,1,1,1,1,1,1,1,1,1,1,1,1,1,1,
1,1,1,1,1,1,1,1,1,1,1,1,1,1,1,1,1,1,1,1,1,1,1,1,1,1,1,1,1,1,1,1,1,1,1,1,
1,1,1,1,1,1,1,1,6),(2,2),(-1.,-0.984615384615383,-0.969230769230768,-0.953846153846152,
-0.938461538461537,-0.923076923076922,-0.907692307692306,-0.892307692307691,
-0.876923076923076,-0.86153846153846,-0.846153846153845,-0.83076923076923,
-0.815384615384614,-0.799999999999999,-0.784615384615384,-0.769230769230768,
-0.753846153846153,-0.738461538461538,-0.723076923076922,-0.707692307692307,
-0.692307692307692,-0.676923076923076,-0.661538461538461,-0.646153846153846,
-0.63076923076923,-0.615384615384615,-0.6,-0.584615384615384,-0.569230769230769,
-0.553846153846154,-0.538461538461538,-0.523076923076923,-0.507692307692308,
-0.492307692307692,-0.476923076923077,-0.461538461538462,-0.446153846153846,
-0.430769230769231,-0.415384615384615,-0.4,-0.384615384615385,-0.369230769230769,
-0.353846153846154,-0.338461538461538,-0.323076923076923,-0.307692307692308,
-0.292307692307692,-0.276923076923077,-0.261538461538462,-0.246153846153846,
-0.230769230769231,-0.215384615384615,-0.2,-0.184615384615385,-0.169230769230769,
-0.153846153846154,-0.138461538461538,-0.123076923076923,-0.107692307692308,
-0.0923076923076923,-0.0769230769230769,-0.0615384615384615,-0.0461538461538462,
-0.0307692307692308,-0.0153846153846154,0.),(-1.,1.),.UNSPECIFIED.)
GEOMETRIC_REPRESENTATION_ITEM()
RATIONAL_B_SPLINE_SURFACE(((1.,1.),(1.,1.),(1.,1.),(1.,1.),(1.,1.),(1.,
1.),(1.,1.),(1.,1.),(1.,1.),(1.,1.),(1.,1.),(1.,1.),(1.,1.),(1.,1.),(1.,
1.),(1.,1.),(1.,1.),(1.,1.),(1.,1.),(1.,1.),(1.,1.),(1.,1.),(1.,1.),(1.,
1.),(1.,1.),(1.,1.),(1.,1.),(1.,1.),(1.,1.),(1.,1.),(1.,1.),(1.,1.),(1.,
1.),(1.,1.),(1.,1.),(1.,1.),(1.,1.),(1.,1.),(1.,1.),(1.,1.),(1.,1.),(1.,
1.),(1.,1.),(1.,1.),(1.,1.),(1.,1.),(1.,1.),(1.,1.),(1.,1.),(1.,1.),(1.,
1.),(1.,1.),(1.,1.),(1.,1.),(1.,1.),(1.,1.),(1.,1.),(1.,1.),(1.,1.),(1.,
1.),(1.,1.),(1.,1.),(1.,1.),(1.,1.),(1.,1.),(1.,1.),(1.,1.),(1.,1.),(1.,
1.),(1.,1.)))
REPRESENTATION_ITEM('')
SURFACE()
);
#23=(
BOUNDED_SURFACE()
B_SPLINE_SURFACE(5,1,((#31238,#31239),(#31240,#31241),(#31242,#31243),(#31244,
#31245),(#31246,#31247),(#31248,#31249),(#31250,#31251),(#31252,#31253),
(#31254,#31255),(#31256,#31257),(#31258,#31259),(#31260,#31261),(#31262,
#31263),(#31264,#31265),(#31266,#31267),(#31268,#31269),(#31270,#31271),
(#31272,#31273),(#31274,#31275),(#31276,#31277),(#31278,#31279),(#31280,
#31281),(#31282,#31283),(#31284,#31285),(#31286,#31287),(#31288,#31289),
(#31290,#31291),(#31292,#31293),(#31294,#31295),(#31296,#31297),(#31298,
#31299),(#31300,#31301),(#31302,#31303),(#31304,#31305),(#31306,#31307),
(#31308,#31309),(#31310,#31311),(#31312,#31313),(#31314,#31315),(#31316,
#31317),(#31318,#31319),(#31320,#31321),(#31322,#31323),(#31324,#31325),
(#31326,#31327),(#31328,#31329),(#31330,#31331),(#31332,#31333),(#31334,
#31335),(#31336,#31337),(#31338,#31339),(#31340,#31341),(#31342,#31343),
(#31344,#31345),(#31346,#31347),(#31348,#31349),(#31350,#31351),(#31352,
#31353),(#31354,#31355),(#31356,#31357),(#31358,#31359),(#31360,#31361),
(#31362,#31363),(#31364,#31365),(#31366,#31367),(#31368,#31369),(#31370,
#31371),(#31372,#31373),(#31374,#31375),(#31376,#31377)),.UNSPECIFIED.,
 .F.,.F.,.F.)
B_SPLINE_SURFACE_WITH_KNOTS((6,1,1,1,1,1,1,1,1,1,1,1,1,1,1,1,1,1,1,1,1,
1,1,1,1,1,1,1,1,1,1,1,1,1,1,1,1,1,1,1,1,1,1,1,1,1,1,1,1,1,1,1,1,1,1,1,1,
1,1,1,1,1,1,1,1,6),(2,2),(-1.,-0.984615384615383,-0.969230769230768,-0.953846153846152,
-0.938461538461537,-0.923076923076922,-0.907692307692306,-0.892307692307691,
-0.876923076923076,-0.86153846153846,-0.846153846153845,-0.83076923076923,
-0.815384615384614,-0.799999999999999,-0.784615384615384,-0.769230769230768,
-0.753846153846153,-0.738461538461538,-0.723076923076922,-0.707692307692307,
-0.692307692307692,-0.676923076923076,-0.661538461538461,-0.646153846153846,
-0.63076923076923,-0.615384615384615,-0.6,-0.584615384615384,-0.569230769230769,
-0.553846153846154,-0.538461538461538,-0.523076923076923,-0.507692307692308,
-0.492307692307692,-0.476923076923077,-0.461538461538462,-0.446153846153846,
-0.430769230769231,-0.415384615384615,-0.4,-0.384615384615385,-0.369230769230769,
-0.353846153846154,-0.338461538461538,-0.323076923076923,-0.307692307692308,
-0.292307692307692,-0.276923076923077,-0.261538461538462,-0.246153846153846,
-0.230769230769231,-0.215384615384615,-0.2,-0.184615384615385,-0.169230769230769,
-0.153846153846154,-0.138461538461538,-0.123076923076923,-0.107692307692308,
-0.0923076923076923,-0.0769230769230769,-0.0615384615384615,-0.0461538461538462,
-0.0307692307692308,-0.0153846153846154,0.),(-1.,1.),.UNSPECIFIED.)
GEOMETRIC_REPRESENTATION_ITEM()
RATIONAL_B_SPLINE_SURFACE(((1.,1.),(1.,1.),(1.,1.),(1.,1.),(1.,1.),(1.,
1.),(1.,1.),(1.,1.),(1.,1.),(1.,1.),(1.,1.),(1.,1.),(1.,1.),(1.,1.),(1.,
1.),(1.,1.),(1.,1.),(1.,1.),(1.,1.),(1.,1.),(1.,1.),(1.,1.),(1.,1.),(1.,
1.),(1.,1.),(1.,1.),(1.,1.),(1.,1.),(1.,1.),(1.,1.),(1.,1.),(1.,1.),(1.,
1.),(1.,1.),(1.,1.),(1.,1.),(1.,1.),(1.,1.),(1.,1.),(1.,1.),(1.,1.),(1.,
1.),(1.,1.),(1.,1.),(1.,1.),(1.,1.),(1.,1.),(1.,1.),(1.,1.),(1.,1.),(1.,
1.),(1.,1.),(1.,1.),(1.,1.),(1.,1.),(1.,1.),(1.,1.),(1.,1.),(1.,1.),(1.,
1.),(1.,1.),(1.,1.),(1.,1.),(1.,1.),(1.,1.),(1.,1.),(1.,1.),(1.,1.),(1.,
1.),(1.,1.)))
REPRESENTATION_ITEM('')
SURFACE()
);
#24=(
BOUNDED_SURFACE()
B_SPLINE_SURFACE(5,1,((#31454,#31455),(#31456,#31457),(#31458,#31459),(#31460,
#31461),(#31462,#31463),(#31464,#31465),(#31466,#31467),(#31468,#31469),
(#31470,#31471),(#31472,#31473),(#31474,#31475),(#31476,#31477),(#31478,
#31479),(#31480,#31481),(#31482,#31483),(#31484,#31485),(#31486,#31487),
(#31488,#31489),(#31490,#31491),(#31492,#31493),(#31494,#31495),(#31496,
#31497),(#31498,#31499),(#31500,#31501),(#31502,#31503),(#31504,#31505),
(#31506,#31507),(#31508,#31509),(#31510,#31511),(#31512,#31513),(#31514,
#31515),(#31516,#31517),(#31518,#31519),(#31520,#31521),(#31522,#31523),
(#31524,#31525),(#31526,#31527),(#31528,#31529),(#31530,#31531),(#31532,
#31533),(#31534,#31535),(#31536,#31537),(#31538,#31539),(#31540,#31541),
(#31542,#31543),(#31544,#31545),(#31546,#31547),(#31548,#31549),(#31550,
#31551),(#31552,#31553),(#31554,#31555),(#31556,#31557),(#31558,#31559),
(#31560,#31561),(#31562,#31563),(#31564,#31565),(#31566,#31567),(#31568,
#31569),(#31570,#31571),(#31572,#31573),(#31574,#31575),(#31576,#31577),
(#31578,#31579),(#31580,#31581),(#31582,#31583),(#31584,#31585),(#31586,
#31587),(#31588,#31589),(#31590,#31591),(#31592,#31593)),.UNSPECIFIED.,
 .F.,.F.,.F.)
B_SPLINE_SURFACE_WITH_KNOTS((6,1,1,1,1,1,1,1,1,1,1,1,1,1,1,1,1,1,1,1,1,
1,1,1,1,1,1,1,1,1,1,1,1,1,1,1,1,1,1,1,1,1,1,1,1,1,1,1,1,1,1,1,1,1,1,1,1,
1,1,1,1,1,1,1,1,6),(2,2),(-1.,-0.984615384615383,-0.969230769230768,-0.953846153846152,
-0.938461538461537,-0.923076923076922,-0.907692307692306,-0.892307692307691,
-0.876923076923076,-0.86153846153846,-0.846153846153845,-0.83076923076923,
-0.815384615384614,-0.799999999999999,-0.784615384615384,-0.769230769230768,
-0.753846153846153,-0.738461538461538,-0.723076923076922,-0.707692307692307,
-0.692307692307692,-0.676923076923076,-0.661538461538461,-0.646153846153846,
-0.63076923076923,-0.615384615384615,-0.6,-0.584615384615384,-0.569230769230769,
-0.553846153846154,-0.538461538461538,-0.523076923076923,-0.507692307692308,
-0.492307692307692,-0.476923076923077,-0.461538461538462,-0.446153846153846,
-0.430769230769231,-0.415384615384615,-0.4,-0.384615384615385,-0.369230769230769,
-0.353846153846154,-0.338461538461538,-0.323076923076923,-0.307692307692308,
-0.292307692307692,-0.276923076923077,-0.261538461538462,-0.246153846153846,
-0.230769230769231,-0.215384615384615,-0.2,-0.184615384615385,-0.169230769230769,
-0.153846153846154,-0.138461538461538,-0.123076923076923,-0.107692307692308,
-0.0923076923076923,-0.0769230769230769,-0.0615384615384615,-0.0461538461538462,
-0.0307692307692308,-0.0153846153846154,0.),(-1.,1.),.UNSPECIFIED.)
GEOMETRIC_REPRESENTATION_ITEM()
RATIONAL_B_SPLINE_SURFACE(((1.,1.),(1.,1.),(1.,1.),(1.,1.),(1.,1.),(1.,
1.),(1.,1.),(1.,1.),(1.,1.),(1.,1.),(1.,1.),(1.,1.),(1.,1.),(1.,1.),(1.,
1.),(1.,1.),(1.,1.),(1.,1.),(1.,1.),(1.,1.),(1.,1.),(1.,1.),(1.,1.),(1.,
1.),(1.,1.),(1.,1.),(1.,1.),(1.,1.),(1.,1.),(1.,1.),(1.,1.),(1.,1.),(1.,
1.),(1.,1.),(1.,1.),(1.,1.),(1.,1.),(1.,1.),(1.,1.),(1.,1.),(1.,1.),(1.,
1.),(1.,1.),(1.,1.),(1.,1.),(1.,1.),(1.,1.),(1.,1.),(1.,1.),(1.,1.),(1.,
1.),(1.,1.),(1.,1.),(1.,1.),(1.,1.),(1.,1.),(1.,1.),(1.,1.),(1.,1.),(1.,
1.),(1.,1.),(1.,1.),(1.,1.),(1.,1.),(1.,1.),(1.,1.),(1.,1.),(1.,1.),(1.,
1.),(1.,1.)))
REPRESENTATION_ITEM('')
SURFACE()
);
#25=(
BOUNDED_SURFACE()
B_SPLINE_SURFACE(5,1,((#31670,#31671),(#31672,#31673),(#31674,#31675),(#31676,
#31677),(#31678,#31679),(#31680,#31681),(#31682,#31683),(#31684,#31685),
(#31686,#31687),(#31688,#31689),(#31690,#31691),(#31692,#31693),(#31694,
#31695),(#31696,#31697),(#31698,#31699),(#31700,#31701),(#31702,#31703),
(#31704,#31705),(#31706,#31707),(#31708,#31709),(#31710,#31711),(#31712,
#31713),(#31714,#31715),(#31716,#31717),(#31718,#31719),(#31720,#31721),
(#31722,#31723),(#31724,#31725),(#31726,#31727),(#31728,#31729),(#31730,
#31731),(#31732,#31733),(#31734,#31735),(#31736,#31737),(#31738,#31739),
(#31740,#31741),(#31742,#31743),(#31744,#31745),(#31746,#31747),(#31748,
#31749),(#31750,#31751),(#31752,#31753),(#31754,#31755),(#31756,#31757),
(#31758,#31759),(#31760,#31761),(#31762,#31763),(#31764,#31765),(#31766,
#31767),(#31768,#31769),(#31770,#31771),(#31772,#31773),(#31774,#31775),
(#31776,#31777),(#31778,#31779),(#31780,#31781),(#31782,#31783),(#31784,
#31785),(#31786,#31787),(#31788,#31789),(#31790,#31791),(#31792,#31793),
(#31794,#31795),(#31796,#31797),(#31798,#31799),(#31800,#31801),(#31802,
#31803),(#31804,#31805),(#31806,#31807),(#31808,#31809)),.UNSPECIFIED.,
 .F.,.F.,.F.)
B_SPLINE_SURFACE_WITH_KNOTS((6,1,1,1,1,1,1,1,1,1,1,1,1,1,1,1,1,1,1,1,1,
1,1,1,1,1,1,1,1,1,1,1,1,1,1,1,1,1,1,1,1,1,1,1,1,1,1,1,1,1,1,1,1,1,1,1,1,
1,1,1,1,1,1,1,1,6),(2,2),(-1.,-0.984615384615383,-0.969230769230768,-0.953846153846152,
-0.938461538461537,-0.923076923076922,-0.907692307692306,-0.892307692307691,
-0.876923076923076,-0.86153846153846,-0.846153846153845,-0.83076923076923,
-0.815384615384614,-0.799999999999999,-0.784615384615384,-0.769230769230768,
-0.753846153846153,-0.738461538461538,-0.723076923076922,-0.707692307692307,
-0.692307692307692,-0.676923076923076,-0.661538461538461,-0.646153846153846,
-0.63076923076923,-0.615384615384615,-0.6,-0.584615384615384,-0.569230769230769,
-0.553846153846154,-0.538461538461538,-0.523076923076923,-0.507692307692308,
-0.492307692307692,-0.476923076923077,-0.461538461538462,-0.446153846153846,
-0.430769230769231,-0.415384615384615,-0.4,-0.384615384615385,-0.369230769230769,
-0.353846153846154,-0.338461538461538,-0.323076923076923,-0.307692307692308,
-0.292307692307692,-0.276923076923077,-0.261538461538462,-0.246153846153846,
-0.230769230769231,-0.215384615384615,-0.2,-0.184615384615385,-0.169230769230769,
-0.153846153846154,-0.138461538461538,-0.123076923076923,-0.107692307692308,
-0.0923076923076923,-0.0769230769230769,-0.0615384615384615,-0.0461538461538462,
-0.0307692307692308,-0.0153846153846154,0.),(-1.,1.),.UNSPECIFIED.)
GEOMETRIC_REPRESENTATION_ITEM()
RATIONAL_B_SPLINE_SURFACE(((1.,1.),(1.,1.),(1.,1.),(1.,1.),(1.,1.),(1.,
1.),(1.,1.),(1.,1.),(1.,1.),(1.,1.),(1.,1.),(1.,1.),(1.,1.),(1.,1.),(1.,
1.),(1.,1.),(1.,1.),(1.,1.),(1.,1.),(1.,1.),(1.,1.),(1.,1.),(1.,1.),(1.,
1.),(1.,1.),(1.,1.),(1.,1.),(1.,1.),(1.,1.),(1.,1.),(1.,1.),(1.,1.),(1.,
1.),(1.,1.),(1.,1.),(1.,1.),(1.,1.),(1.,1.),(1.,1.),(1.,1.),(1.,1.),(1.,
1.),(1.,1.),(1.,1.),(1.,1.),(1.,1.),(1.,1.),(1.,1.),(1.,1.),(1.,1.),(1.,
1.),(1.,1.),(1.,1.),(1.,1.),(1.,1.),(1.,1.),(1.,1.),(1.,1.),(1.,1.),(1.,
1.),(1.,1.),(1.,1.),(1.,1.),(1.,1.),(1.,1.),(1.,1.),(1.,1.),(1.,1.),(1.,
1.),(1.,1.)))
REPRESENTATION_ITEM('')
SURFACE()
);
#26=(
BOUNDED_SURFACE()
B_SPLINE_SURFACE(5,1,((#31886,#31887),(#31888,#31889),(#31890,#31891),(#31892,
#31893),(#31894,#31895),(#31896,#31897),(#31898,#31899),(#31900,#31901),
(#31902,#31903),(#31904,#31905),(#31906,#31907),(#31908,#31909),(#31910,
#31911),(#31912,#31913),(#31914,#31915),(#31916,#31917),(#31918,#31919),
(#31920,#31921),(#31922,#31923),(#31924,#31925),(#31926,#31927),(#31928,
#31929),(#31930,#31931),(#31932,#31933),(#31934,#31935),(#31936,#31937),
(#31938,#31939),(#31940,#31941),(#31942,#31943),(#31944,#31945),(#31946,
#31947),(#31948,#31949),(#31950,#31951),(#31952,#31953),(#31954,#31955),
(#31956,#31957),(#31958,#31959),(#31960,#31961),(#31962,#31963),(#31964,
#31965),(#31966,#31967),(#31968,#31969),(#31970,#31971),(#31972,#31973),
(#31974,#31975),(#31976,#31977),(#31978,#31979),(#31980,#31981),(#31982,
#31983),(#31984,#31985),(#31986,#31987),(#31988,#31989),(#31990,#31991),
(#31992,#31993),(#31994,#31995),(#31996,#31997),(#31998,#31999),(#32000,
#32001),(#32002,#32003),(#32004,#32005),(#32006,#32007),(#32008,#32009),
(#32010,#32011),(#32012,#32013),(#32014,#32015),(#32016,#32017),(#32018,
#32019),(#32020,#32021),(#32022,#32023),(#32024,#32025)),.UNSPECIFIED.,
 .F.,.F.,.F.)
B_SPLINE_SURFACE_WITH_KNOTS((6,1,1,1,1,1,1,1,1,1,1,1,1,1,1,1,1,1,1,1,1,
1,1,1,1,1,1,1,1,1,1,1,1,1,1,1,1,1,1,1,1,1,1,1,1,1,1,1,1,1,1,1,1,1,1,1,1,
1,1,1,1,1,1,1,1,6),(2,2),(-1.,-0.984615384615383,-0.969230769230768,-0.953846153846152,
-0.938461538461537,-0.923076923076922,-0.907692307692306,-0.892307692307691,
-0.876923076923076,-0.86153846153846,-0.846153846153845,-0.83076923076923,
-0.815384615384614,-0.799999999999999,-0.784615384615384,-0.769230769230768,
-0.753846153846153,-0.738461538461538,-0.723076923076922,-0.707692307692307,
-0.692307692307692,-0.676923076923076,-0.661538461538461,-0.646153846153846,
-0.63076923076923,-0.615384615384615,-0.6,-0.584615384615384,-0.569230769230769,
-0.553846153846154,-0.538461538461538,-0.523076923076923,-0.507692307692308,
-0.492307692307692,-0.476923076923077,-0.461538461538462,-0.446153846153846,
-0.430769230769231,-0.415384615384615,-0.4,-0.384615384615385,-0.369230769230769,
-0.353846153846154,-0.338461538461538,-0.323076923076923,-0.307692307692308,
-0.292307692307692,-0.276923076923077,-0.261538461538462,-0.246153846153846,
-0.230769230769231,-0.215384615384615,-0.2,-0.184615384615385,-0.169230769230769,
-0.153846153846154,-0.138461538461538,-0.123076923076923,-0.107692307692308,
-0.0923076923076923,-0.0769230769230769,-0.0615384615384615,-0.0461538461538462,
-0.0307692307692308,-0.0153846153846154,0.),(-1.,1.),.UNSPECIFIED.)
GEOMETRIC_REPRESENTATION_ITEM()
RATIONAL_B_SPLINE_SURFACE(((1.,1.),(1.,1.),(1.,1.),(1.,1.),(1.,1.),(1.,
1.),(1.,1.),(1.,1.),(1.,1.),(1.,1.),(1.,1.),(1.,1.),(1.,1.),(1.,1.),(1.,
1.),(1.,1.),(1.,1.),(1.,1.),(1.,1.),(1.,1.),(1.,1.),(1.,1.),(1.,1.),(1.,
1.),(1.,1.),(1.,1.),(1.,1.),(1.,1.),(1.,1.),(1.,1.),(1.,1.),(1.,1.),(1.,
1.),(1.,1.),(1.,1.),(1.,1.),(1.,1.),(1.,1.),(1.,1.),(1.,1.),(1.,1.),(1.,
1.),(1.,1.),(1.,1.),(1.,1.),(1.,1.),(1.,1.),(1.,1.),(1.,1.),(1.,1.),(1.,
1.),(1.,1.),(1.,1.),(1.,1.),(1.,1.),(1.,1.),(1.,1.),(1.,1.),(1.,1.),(1.,
1.),(1.,1.),(1.,1.),(1.,1.),(1.,1.),(1.,1.),(1.,1.),(1.,1.),(1.,1.),(1.,
1.),(1.,1.)))
REPRESENTATION_ITEM('')
SURFACE()
);
#27=(
BOUNDED_SURFACE()
B_SPLINE_SURFACE(5,1,((#32102,#32103),(#32104,#32105),(#32106,#32107),(#32108,
#32109),(#32110,#32111),(#32112,#32113),(#32114,#32115),(#32116,#32117),
(#32118,#32119),(#32120,#32121),(#32122,#32123),(#32124,#32125),(#32126,
#32127),(#32128,#32129),(#32130,#32131),(#32132,#32133),(#32134,#32135),
(#32136,#32137),(#32138,#32139),(#32140,#32141),(#32142,#32143),(#32144,
#32145),(#32146,#32147),(#32148,#32149),(#32150,#32151),(#32152,#32153),
(#32154,#32155),(#32156,#32157),(#32158,#32159),(#32160,#32161),(#32162,
#32163),(#32164,#32165),(#32166,#32167),(#32168,#32169),(#32170,#32171),
(#32172,#32173),(#32174,#32175),(#32176,#32177),(#32178,#32179),(#32180,
#32181),(#32182,#32183),(#32184,#32185),(#32186,#32187),(#32188,#32189),
(#32190,#32191),(#32192,#32193),(#32194,#32195),(#32196,#32197),(#32198,
#32199),(#32200,#32201),(#32202,#32203),(#32204,#32205),(#32206,#32207),
(#32208,#32209),(#32210,#32211),(#32212,#32213),(#32214,#32215),(#32216,
#32217),(#32218,#32219),(#32220,#32221),(#32222,#32223),(#32224,#32225),
(#32226,#32227),(#32228,#32229),(#32230,#32231),(#32232,#32233),(#32234,
#32235),(#32236,#32237),(#32238,#32239),(#32240,#32241)),.UNSPECIFIED.,
 .F.,.F.,.F.)
B_SPLINE_SURFACE_WITH_KNOTS((6,1,1,1,1,1,1,1,1,1,1,1,1,1,1,1,1,1,1,1,1,
1,1,1,1,1,1,1,1,1,1,1,1,1,1,1,1,1,1,1,1,1,1,1,1,1,1,1,1,1,1,1,1,1,1,1,1,
1,1,1,1,1,1,1,1,6),(2,2),(-1.,-0.984615384615383,-0.969230769230768,-0.953846153846152,
-0.938461538461537,-0.923076923076922,-0.907692307692306,-0.892307692307691,
-0.876923076923076,-0.86153846153846,-0.846153846153845,-0.83076923076923,
-0.815384615384614,-0.799999999999999,-0.784615384615384,-0.769230769230768,
-0.753846153846153,-0.738461538461538,-0.723076923076922,-0.707692307692307,
-0.692307692307692,-0.676923076923076,-0.661538461538461,-0.646153846153846,
-0.63076923076923,-0.615384615384615,-0.6,-0.584615384615384,-0.569230769230769,
-0.553846153846154,-0.538461538461538,-0.523076923076923,-0.507692307692308,
-0.492307692307692,-0.476923076923077,-0.461538461538462,-0.446153846153846,
-0.430769230769231,-0.415384615384615,-0.4,-0.384615384615385,-0.369230769230769,
-0.353846153846154,-0.338461538461538,-0.323076923076923,-0.307692307692308,
-0.292307692307692,-0.276923076923077,-0.261538461538462,-0.246153846153846,
-0.230769230769231,-0.215384615384615,-0.2,-0.184615384615385,-0.169230769230769,
-0.153846153846154,-0.138461538461538,-0.123076923076923,-0.107692307692308,
-0.0923076923076923,-0.0769230769230769,-0.0615384615384615,-0.0461538461538462,
-0.0307692307692308,-0.0153846153846154,0.),(-1.,1.),.UNSPECIFIED.)
GEOMETRIC_REPRESENTATION_ITEM()
RATIONAL_B_SPLINE_SURFACE(((1.,1.),(1.,1.),(1.,1.),(1.,1.),(1.,1.),(1.,
1.),(1.,1.),(1.,1.),(1.,1.),(1.,1.),(1.,1.),(1.,1.),(1.,1.),(1.,1.),(1.,
1.),(1.,1.),(1.,1.),(1.,1.),(1.,1.),(1.,1.),(1.,1.),(1.,1.),(1.,1.),(1.,
1.),(1.,1.),(1.,1.),(1.,1.),(1.,1.),(1.,1.),(1.,1.),(1.,1.),(1.,1.),(1.,
1.),(1.,1.),(1.,1.),(1.,1.),(1.,1.),(1.,1.),(1.,1.),(1.,1.),(1.,1.),(1.,
1.),(1.,1.),(1.,1.),(1.,1.),(1.,1.),(1.,1.),(1.,1.),(1.,1.),(1.,1.),(1.,
1.),(1.,1.),(1.,1.),(1.,1.),(1.,1.),(1.,1.),(1.,1.),(1.,1.),(1.,1.),(1.,
1.),(1.,1.),(1.,1.),(1.,1.),(1.,1.),(1.,1.),(1.,1.),(1.,1.),(1.,1.),(1.,
1.),(1.,1.)))
REPRESENTATION_ITEM('')
SURFACE()
);
#28=(
BOUNDED_SURFACE()
B_SPLINE_SURFACE(5,1,((#32318,#32319),(#32320,#32321),(#32322,#32323),(#32324,
#32325),(#32326,#32327),(#32328,#32329),(#32330,#32331),(#32332,#32333),
(#32334,#32335),(#32336,#32337),(#32338,#32339),(#32340,#32341),(#32342,
#32343),(#32344,#32345),(#32346,#32347),(#32348,#32349),(#32350,#32351),
(#32352,#32353),(#32354,#32355),(#32356,#32357),(#32358,#32359),(#32360,
#32361),(#32362,#32363),(#32364,#32365),(#32366,#32367),(#32368,#32369),
(#32370,#32371),(#32372,#32373),(#32374,#32375),(#32376,#32377),(#32378,
#32379),(#32380,#32381),(#32382,#32383),(#32384,#32385),(#32386,#32387),
(#32388,#32389),(#32390,#32391),(#32392,#32393),(#32394,#32395),(#32396,
#32397),(#32398,#32399),(#32400,#32401),(#32402,#32403),(#32404,#32405),
(#32406,#32407),(#32408,#32409),(#32410,#32411),(#32412,#32413),(#32414,
#32415),(#32416,#32417),(#32418,#32419),(#32420,#32421),(#32422,#32423),
(#32424,#32425),(#32426,#32427),(#32428,#32429),(#32430,#32431),(#32432,
#32433),(#32434,#32435),(#32436,#32437),(#32438,#32439),(#32440,#32441),
(#32442,#32443),(#32444,#32445),(#32446,#32447),(#32448,#32449),(#32450,
#32451),(#32452,#32453),(#32454,#32455),(#32456,#32457)),.UNSPECIFIED.,
 .F.,.F.,.F.)
B_SPLINE_SURFACE_WITH_KNOTS((6,1,1,1,1,1,1,1,1,1,1,1,1,1,1,1,1,1,1,1,1,
1,1,1,1,1,1,1,1,1,1,1,1,1,1,1,1,1,1,1,1,1,1,1,1,1,1,1,1,1,1,1,1,1,1,1,1,
1,1,1,1,1,1,1,1,6),(2,2),(-1.,-0.984615384615383,-0.969230769230768,-0.953846153846152,
-0.938461538461537,-0.923076923076922,-0.907692307692306,-0.892307692307691,
-0.876923076923076,-0.86153846153846,-0.846153846153845,-0.83076923076923,
-0.815384615384614,-0.799999999999999,-0.784615384615384,-0.769230769230768,
-0.753846153846153,-0.738461538461538,-0.723076923076922,-0.707692307692307,
-0.692307692307692,-0.676923076923076,-0.661538461538461,-0.646153846153846,
-0.63076923076923,-0.615384615384615,-0.6,-0.584615384615384,-0.569230769230769,
-0.553846153846154,-0.538461538461538,-0.523076923076923,-0.507692307692308,
-0.492307692307692,-0.476923076923077,-0.461538461538462,-0.446153846153846,
-0.430769230769231,-0.415384615384615,-0.4,-0.384615384615385,-0.369230769230769,
-0.353846153846154,-0.338461538461538,-0.323076923076923,-0.307692307692308,
-0.292307692307692,-0.276923076923077,-0.261538461538462,-0.246153846153846,
-0.230769230769231,-0.215384615384615,-0.2,-0.184615384615385,-0.169230769230769,
-0.153846153846154,-0.138461538461538,-0.123076923076923,-0.107692307692308,
-0.0923076923076923,-0.0769230769230769,-0.0615384615384615,-0.0461538461538462,
-0.0307692307692308,-0.0153846153846154,0.),(-1.,1.),.UNSPECIFIED.)
GEOMETRIC_REPRESENTATION_ITEM()
RATIONAL_B_SPLINE_SURFACE(((1.,1.),(1.,1.),(1.,1.),(1.,1.),(1.,1.),(1.,
1.),(1.,1.),(1.,1.),(1.,1.),(1.,1.),(1.,1.),(1.,1.),(1.,1.),(1.,1.),(1.,
1.),(1.,1.),(1.,1.),(1.,1.),(1.,1.),(1.,1.),(1.,1.),(1.,1.),(1.,1.),(1.,
1.),(1.,1.),(1.,1.),(1.,1.),(1.,1.),(1.,1.),(1.,1.),(1.,1.),(1.,1.),(1.,
1.),(1.,1.),(1.,1.),(1.,1.),(1.,1.),(1.,1.),(1.,1.),(1.,1.),(1.,1.),(1.,
1.),(1.,1.),(1.,1.),(1.,1.),(1.,1.),(1.,1.),(1.,1.),(1.,1.),(1.,1.),(1.,
1.),(1.,1.),(1.,1.),(1.,1.),(1.,1.),(1.,1.),(1.,1.),(1.,1.),(1.,1.),(1.,
1.),(1.,1.),(1.,1.),(1.,1.),(1.,1.),(1.,1.),(1.,1.),(1.,1.),(1.,1.),(1.,
1.),(1.,1.)))
REPRESENTATION_ITEM('')
SURFACE()
);
#29=(
BOUNDED_SURFACE()
B_SPLINE_SURFACE(5,1,((#32534,#32535),(#32536,#32537),(#32538,#32539),(#32540,
#32541),(#32542,#32543),(#32544,#32545),(#32546,#32547),(#32548,#32549),
(#32550,#32551),(#32552,#32553),(#32554,#32555),(#32556,#32557),(#32558,
#32559),(#32560,#32561),(#32562,#32563),(#32564,#32565),(#32566,#32567),
(#32568,#32569),(#32570,#32571),(#32572,#32573),(#32574,#32575),(#32576,
#32577),(#32578,#32579),(#32580,#32581),(#32582,#32583),(#32584,#32585),
(#32586,#32587),(#32588,#32589),(#32590,#32591),(#32592,#32593),(#32594,
#32595),(#32596,#32597),(#32598,#32599),(#32600,#32601),(#32602,#32603),
(#32604,#32605),(#32606,#32607),(#32608,#32609),(#32610,#32611),(#32612,
#32613),(#32614,#32615),(#32616,#32617),(#32618,#32619),(#32620,#32621),
(#32622,#32623),(#32624,#32625),(#32626,#32627),(#32628,#32629),(#32630,
#32631),(#32632,#32633),(#32634,#32635),(#32636,#32637),(#32638,#32639),
(#32640,#32641),(#32642,#32643),(#32644,#32645),(#32646,#32647),(#32648,
#32649),(#32650,#32651),(#32652,#32653),(#32654,#32655),(#32656,#32657),
(#32658,#32659),(#32660,#32661),(#32662,#32663),(#32664,#32665),(#32666,
#32667),(#32668,#32669),(#32670,#32671),(#32672,#32673)),.UNSPECIFIED.,
 .F.,.F.,.F.)
B_SPLINE_SURFACE_WITH_KNOTS((6,1,1,1,1,1,1,1,1,1,1,1,1,1,1,1,1,1,1,1,1,
1,1,1,1,1,1,1,1,1,1,1,1,1,1,1,1,1,1,1,1,1,1,1,1,1,1,1,1,1,1,1,1,1,1,1,1,
1,1,1,1,1,1,1,1,6),(2,2),(-1.,-0.984615384615383,-0.969230769230768,-0.953846153846152,
-0.938461538461537,-0.923076923076922,-0.907692307692306,-0.892307692307691,
-0.876923076923076,-0.86153846153846,-0.846153846153845,-0.83076923076923,
-0.815384615384614,-0.799999999999999,-0.784615384615384,-0.769230769230768,
-0.753846153846153,-0.738461538461538,-0.723076923076922,-0.707692307692307,
-0.692307692307692,-0.676923076923076,-0.661538461538461,-0.646153846153846,
-0.63076923076923,-0.615384615384615,-0.6,-0.584615384615384,-0.569230769230769,
-0.553846153846154,-0.538461538461538,-0.523076923076923,-0.507692307692308,
-0.492307692307692,-0.476923076923077,-0.461538461538462,-0.446153846153846,
-0.430769230769231,-0.415384615384615,-0.4,-0.384615384615385,-0.369230769230769,
-0.353846153846154,-0.338461538461538,-0.323076923076923,-0.307692307692308,
-0.292307692307692,-0.276923076923077,-0.261538461538462,-0.246153846153846,
-0.230769230769231,-0.215384615384615,-0.2,-0.184615384615385,-0.169230769230769,
-0.153846153846154,-0.138461538461538,-0.123076923076923,-0.107692307692308,
-0.0923076923076923,-0.0769230769230769,-0.0615384615384615,-0.0461538461538462,
-0.0307692307692308,-0.0153846153846154,0.),(-1.,1.),.UNSPECIFIED.)
GEOMETRIC_REPRESENTATION_ITEM()
RATIONAL_B_SPLINE_SURFACE(((1.,1.),(1.,1.),(1.,1.),(1.,1.),(1.,1.),(1.,
1.),(1.,1.),(1.,1.),(1.,1.),(1.,1.),(1.,1.),(1.,1.),(1.,1.),(1.,1.),(1.,
1.),(1.,1.),(1.,1.),(1.,1.),(1.,1.),(1.,1.),(1.,1.),(1.,1.),(1.,1.),(1.,
1.),(1.,1.),(1.,1.),(1.,1.),(1.,1.),(1.,1.),(1.,1.),(1.,1.),(1.,1.),(1.,
1.),(1.,1.),(1.,1.),(1.,1.),(1.,1.),(1.,1.),(1.,1.),(1.,1.),(1.,1.),(1.,
1.),(1.,1.),(1.,1.),(1.,1.),(1.,1.),(1.,1.),(1.,1.),(1.,1.),(1.,1.),(1.,
1.),(1.,1.),(1.,1.),(1.,1.),(1.,1.),(1.,1.),(1.,1.),(1.,1.),(1.,1.),(1.,
1.),(1.,1.),(1.,1.),(1.,1.),(1.,1.),(1.,1.),(1.,1.),(1.,1.),(1.,1.),(1.,
1.),(1.,1.)))
REPRESENTATION_ITEM('')
SURFACE()
);
#30=(
BOUNDED_SURFACE()
B_SPLINE_SURFACE(5,1,((#32750,#32751),(#32752,#32753),(#32754,#32755),(#32756,
#32757),(#32758,#32759),(#32760,#32761),(#32762,#32763),(#32764,#32765),
(#32766,#32767),(#32768,#32769),(#32770,#32771),(#32772,#32773),(#32774,
#32775),(#32776,#32777),(#32778,#32779),(#32780,#32781),(#32782,#32783),
(#32784,#32785),(#32786,#32787),(#32788,#32789),(#32790,#32791),(#32792,
#32793),(#32794,#32795),(#32796,#32797),(#32798,#32799),(#32800,#32801),
(#32802,#32803),(#32804,#32805),(#32806,#32807),(#32808,#32809),(#32810,
#32811),(#32812,#32813),(#32814,#32815),(#32816,#32817),(#32818,#32819),
(#32820,#32821),(#32822,#32823),(#32824,#32825),(#32826,#32827),(#32828,
#32829),(#32830,#32831),(#32832,#32833),(#32834,#32835),(#32836,#32837),
(#32838,#32839),(#32840,#32841),(#32842,#32843),(#32844,#32845),(#32846,
#32847),(#32848,#32849),(#32850,#32851),(#32852,#32853),(#32854,#32855),
(#32856,#32857),(#32858,#32859),(#32860,#32861),(#32862,#32863),(#32864,
#32865),(#32866,#32867),(#32868,#32869),(#32870,#32871),(#32872,#32873),
(#32874,#32875),(#32876,#32877),(#32878,#32879),(#32880,#32881),(#32882,
#32883),(#32884,#32885),(#32886,#32887),(#32888,#32889)),.UNSPECIFIED.,
 .F.,.F.,.F.)
B_SPLINE_SURFACE_WITH_KNOTS((6,1,1,1,1,1,1,1,1,1,1,1,1,1,1,1,1,1,1,1,1,
1,1,1,1,1,1,1,1,1,1,1,1,1,1,1,1,1,1,1,1,1,1,1,1,1,1,1,1,1,1,1,1,1,1,1,1,
1,1,1,1,1,1,1,1,6),(2,2),(-1.,-0.984615384615383,-0.969230769230768,-0.953846153846152,
-0.938461538461537,-0.923076923076922,-0.907692307692306,-0.892307692307691,
-0.876923076923076,-0.86153846153846,-0.846153846153845,-0.83076923076923,
-0.815384615384614,-0.799999999999999,-0.784615384615384,-0.769230769230768,
-0.753846153846153,-0.738461538461538,-0.723076923076922,-0.707692307692307,
-0.692307692307692,-0.676923076923076,-0.661538461538461,-0.646153846153846,
-0.63076923076923,-0.615384615384615,-0.6,-0.584615384615384,-0.569230769230769,
-0.553846153846154,-0.538461538461538,-0.523076923076923,-0.507692307692308,
-0.492307692307692,-0.476923076923077,-0.461538461538462,-0.446153846153846,
-0.430769230769231,-0.415384615384615,-0.4,-0.384615384615385,-0.369230769230769,
-0.353846153846154,-0.338461538461538,-0.323076923076923,-0.307692307692308,
-0.292307692307692,-0.276923076923077,-0.261538461538462,-0.246153846153846,
-0.230769230769231,-0.215384615384615,-0.2,-0.184615384615385,-0.169230769230769,
-0.153846153846154,-0.138461538461538,-0.123076923076923,-0.107692307692308,
-0.0923076923076923,-0.0769230769230769,-0.0615384615384615,-0.0461538461538462,
-0.0307692307692308,-0.0153846153846154,0.),(-1.,1.),.UNSPECIFIED.)
GEOMETRIC_REPRESENTATION_ITEM()
RATIONAL_B_SPLINE_SURFACE(((1.,1.),(1.,1.),(1.,1.),(1.,1.),(1.,1.),(1.,
1.),(1.,1.),(1.,1.),(1.,1.),(1.,1.),(1.,1.),(1.,1.),(1.,1.),(1.,1.),(1.,
1.),(1.,1.),(1.,1.),(1.,1.),(1.,1.),(1.,1.),(1.,1.),(1.,1.),(1.,1.),(1.,
1.),(1.,1.),(1.,1.),(1.,1.),(1.,1.),(1.,1.),(1.,1.),(1.,1.),(1.,1.),(1.,
1.),(1.,1.),(1.,1.),(1.,1.),(1.,1.),(1.,1.),(1.,1.),(1.,1.),(1.,1.),(1.,
1.),(1.,1.),(1.,1.),(1.,1.),(1.,1.),(1.,1.),(1.,1.),(1.,1.),(1.,1.),(1.,
1.),(1.,1.),(1.,1.),(1.,1.),(1.,1.),(1.,1.),(1.,1.),(1.,1.),(1.,1.),(1.,
1.),(1.,1.),(1.,1.),(1.,1.),(1.,1.),(1.,1.),(1.,1.),(1.,1.),(1.,1.),(1.,
1.),(1.,1.)))
REPRESENTATION_ITEM('')
SURFACE()
);
#31=(
BOUNDED_SURFACE()
B_SPLINE_SURFACE(5,1,((#32966,#32967),(#32968,#32969),(#32970,#32971),(#32972,
#32973),(#32974,#32975),(#32976,#32977),(#32978,#32979),(#32980,#32981),
(#32982,#32983),(#32984,#32985),(#32986,#32987),(#32988,#32989),(#32990,
#32991),(#32992,#32993),(#32994,#32995),(#32996,#32997),(#32998,#32999),
(#33000,#33001),(#33002,#33003),(#33004,#33005),(#33006,#33007),(#33008,
#33009),(#33010,#33011),(#33012,#33013),(#33014,#33015),(#33016,#33017),
(#33018,#33019),(#33020,#33021),(#33022,#33023),(#33024,#33025),(#33026,
#33027),(#33028,#33029),(#33030,#33031),(#33032,#33033),(#33034,#33035),
(#33036,#33037),(#33038,#33039),(#33040,#33041),(#33042,#33043),(#33044,
#33045),(#33046,#33047),(#33048,#33049),(#33050,#33051),(#33052,#33053),
(#33054,#33055),(#33056,#33057),(#33058,#33059),(#33060,#33061),(#33062,
#33063),(#33064,#33065),(#33066,#33067),(#33068,#33069),(#33070,#33071),
(#33072,#33073),(#33074,#33075),(#33076,#33077),(#33078,#33079),(#33080,
#33081),(#33082,#33083),(#33084,#33085),(#33086,#33087),(#33088,#33089),
(#33090,#33091),(#33092,#33093),(#33094,#33095),(#33096,#33097),(#33098,
#33099),(#33100,#33101),(#33102,#33103),(#33104,#33105)),.UNSPECIFIED.,
 .F.,.F.,.F.)
B_SPLINE_SURFACE_WITH_KNOTS((6,1,1,1,1,1,1,1,1,1,1,1,1,1,1,1,1,1,1,1,1,
1,1,1,1,1,1,1,1,1,1,1,1,1,1,1,1,1,1,1,1,1,1,1,1,1,1,1,1,1,1,1,1,1,1,1,1,
1,1,1,1,1,1,1,1,6),(2,2),(-1.,-0.984615384615383,-0.969230769230768,-0.953846153846152,
-0.938461538461537,-0.923076923076922,-0.907692307692306,-0.892307692307691,
-0.876923076923076,-0.86153846153846,-0.846153846153845,-0.83076923076923,
-0.815384615384614,-0.799999999999999,-0.784615384615384,-0.769230769230768,
-0.753846153846153,-0.738461538461538,-0.723076923076922,-0.707692307692307,
-0.692307692307692,-0.676923076923076,-0.661538461538461,-0.646153846153846,
-0.63076923076923,-0.615384615384615,-0.6,-0.584615384615384,-0.569230769230769,
-0.553846153846154,-0.538461538461538,-0.523076923076923,-0.507692307692308,
-0.492307692307692,-0.476923076923077,-0.461538461538462,-0.446153846153846,
-0.430769230769231,-0.415384615384615,-0.4,-0.384615384615385,-0.369230769230769,
-0.353846153846154,-0.338461538461538,-0.323076923076923,-0.307692307692308,
-0.292307692307692,-0.276923076923077,-0.261538461538462,-0.246153846153846,
-0.230769230769231,-0.215384615384615,-0.2,-0.184615384615385,-0.169230769230769,
-0.153846153846154,-0.138461538461538,-0.123076923076923,-0.107692307692308,
-0.0923076923076923,-0.0769230769230769,-0.0615384615384615,-0.0461538461538462,
-0.0307692307692308,-0.0153846153846154,0.),(-1.,1.),.UNSPECIFIED.)
GEOMETRIC_REPRESENTATION_ITEM()
RATIONAL_B_SPLINE_SURFACE(((1.,1.),(1.,1.),(1.,1.),(1.,1.),(1.,1.),(1.,
1.),(1.,1.),(1.,1.),(1.,1.),(1.,1.),(1.,1.),(1.,1.),(1.,1.),(1.,1.),(1.,
1.),(1.,1.),(1.,1.),(1.,1.),(1.,1.),(1.,1.),(1.,1.),(1.,1.),(1.,1.),(1.,
1.),(1.,1.),(1.,1.),(1.,1.),(1.,1.),(1.,1.),(1.,1.),(1.,1.),(1.,1.),(1.,
1.),(1.,1.),(1.,1.),(1.,1.),(1.,1.),(1.,1.),(1.,1.),(1.,1.),(1.,1.),(1.,
1.),(1.,1.),(1.,1.),(1.,1.),(1.,1.),(1.,1.),(1.,1.),(1.,1.),(1.,1.),(1.,
1.),(1.,1.),(1.,1.),(1.,1.),(1.,1.),(1.,1.),(1.,1.),(1.,1.),(1.,1.),(1.,
1.),(1.,1.),(1.,1.),(1.,1.),(1.,1.),(1.,1.),(1.,1.),(1.,1.),(1.,1.),(1.,
1.),(1.,1.)))
REPRESENTATION_ITEM('')
SURFACE()
);
#32=(
BOUNDED_SURFACE()
B_SPLINE_SURFACE(5,1,((#33182,#33183),(#33184,#33185),(#33186,#33187),(#33188,
#33189),(#33190,#33191),(#33192,#33193),(#33194,#33195),(#33196,#33197),
(#33198,#33199),(#33200,#33201),(#33202,#33203),(#33204,#33205),(#33206,
#33207),(#33208,#33209),(#33210,#33211),(#33212,#33213),(#33214,#33215),
(#33216,#33217),(#33218,#33219),(#33220,#33221),(#33222,#33223),(#33224,
#33225),(#33226,#33227),(#33228,#33229),(#33230,#33231),(#33232,#33233),
(#33234,#33235),(#33236,#33237),(#33238,#33239),(#33240,#33241),(#33242,
#33243),(#33244,#33245),(#33246,#33247),(#33248,#33249),(#33250,#33251),
(#33252,#33253),(#33254,#33255),(#33256,#33257),(#33258,#33259),(#33260,
#33261),(#33262,#33263),(#33264,#33265),(#33266,#33267),(#33268,#33269),
(#33270,#33271),(#33272,#33273),(#33274,#33275),(#33276,#33277),(#33278,
#33279),(#33280,#33281),(#33282,#33283),(#33284,#33285),(#33286,#33287),
(#33288,#33289),(#33290,#33291),(#33292,#33293),(#33294,#33295),(#33296,
#33297),(#33298,#33299),(#33300,#33301),(#33302,#33303),(#33304,#33305),
(#33306,#33307),(#33308,#33309),(#33310,#33311),(#33312,#33313),(#33314,
#33315),(#33316,#33317),(#33318,#33319),(#33320,#33321)),.UNSPECIFIED.,
 .F.,.F.,.F.)
B_SPLINE_SURFACE_WITH_KNOTS((6,1,1,1,1,1,1,1,1,1,1,1,1,1,1,1,1,1,1,1,1,
1,1,1,1,1,1,1,1,1,1,1,1,1,1,1,1,1,1,1,1,1,1,1,1,1,1,1,1,1,1,1,1,1,1,1,1,
1,1,1,1,1,1,1,1,6),(2,2),(-1.,-0.984615384615383,-0.969230769230768,-0.953846153846152,
-0.938461538461537,-0.923076923076922,-0.907692307692306,-0.892307692307691,
-0.876923076923076,-0.86153846153846,-0.846153846153845,-0.83076923076923,
-0.815384615384614,-0.799999999999999,-0.784615384615384,-0.769230769230768,
-0.753846153846153,-0.738461538461538,-0.723076923076922,-0.707692307692307,
-0.692307692307692,-0.676923076923076,-0.661538461538461,-0.646153846153846,
-0.63076923076923,-0.615384615384615,-0.6,-0.584615384615384,-0.569230769230769,
-0.553846153846154,-0.538461538461538,-0.523076923076923,-0.507692307692308,
-0.492307692307692,-0.476923076923077,-0.461538461538462,-0.446153846153846,
-0.430769230769231,-0.415384615384615,-0.4,-0.384615384615385,-0.369230769230769,
-0.353846153846154,-0.338461538461538,-0.323076923076923,-0.307692307692308,
-0.292307692307692,-0.276923076923077,-0.261538461538462,-0.246153846153846,
-0.230769230769231,-0.215384615384615,-0.2,-0.184615384615385,-0.169230769230769,
-0.153846153846154,-0.138461538461538,-0.123076923076923,-0.107692307692308,
-0.0923076923076923,-0.0769230769230769,-0.0615384615384615,-0.0461538461538462,
-0.0307692307692308,-0.0153846153846154,0.),(-1.,1.),.UNSPECIFIED.)
GEOMETRIC_REPRESENTATION_ITEM()
RATIONAL_B_SPLINE_SURFACE(((1.,1.),(1.,1.),(1.,1.),(1.,1.),(1.,1.),(1.,
1.),(1.,1.),(1.,1.),(1.,1.),(1.,1.),(1.,1.),(1.,1.),(1.,1.),(1.,1.),(1.,
1.),(1.,1.),(1.,1.),(1.,1.),(1.,1.),(1.,1.),(1.,1.),(1.,1.),(1.,1.),(1.,
1.),(1.,1.),(1.,1.),(1.,1.),(1.,1.),(1.,1.),(1.,1.),(1.,1.),(1.,1.),(1.,
1.),(1.,1.),(1.,1.),(1.,1.),(1.,1.),(1.,1.),(1.,1.),(1.,1.),(1.,1.),(1.,
1.),(1.,1.),(1.,1.),(1.,1.),(1.,1.),(1.,1.),(1.,1.),(1.,1.),(1.,1.),(1.,
1.),(1.,1.),(1.,1.),(1.,1.),(1.,1.),(1.,1.),(1.,1.),(1.,1.),(1.,1.),(1.,
1.),(1.,1.),(1.,1.),(1.,1.),(1.,1.),(1.,1.),(1.,1.),(1.,1.),(1.,1.),(1.,
1.),(1.,1.)))
REPRESENTATION_ITEM('')
SURFACE()
);
#33=(
BOUNDED_SURFACE()
B_SPLINE_SURFACE(5,1,((#33398,#33399),(#33400,#33401),(#33402,#33403),(#33404,
#33405),(#33406,#33407),(#33408,#33409),(#33410,#33411),(#33412,#33413),
(#33414,#33415),(#33416,#33417),(#33418,#33419),(#33420,#33421),(#33422,
#33423),(#33424,#33425),(#33426,#33427),(#33428,#33429),(#33430,#33431),
(#33432,#33433),(#33434,#33435),(#33436,#33437),(#33438,#33439),(#33440,
#33441),(#33442,#33443),(#33444,#33445),(#33446,#33447),(#33448,#33449),
(#33450,#33451),(#33452,#33453),(#33454,#33455),(#33456,#33457),(#33458,
#33459),(#33460,#33461),(#33462,#33463),(#33464,#33465),(#33466,#33467),
(#33468,#33469),(#33470,#33471),(#33472,#33473),(#33474,#33475),(#33476,
#33477),(#33478,#33479),(#33480,#33481),(#33482,#33483),(#33484,#33485),
(#33486,#33487),(#33488,#33489),(#33490,#33491),(#33492,#33493),(#33494,
#33495),(#33496,#33497),(#33498,#33499),(#33500,#33501),(#33502,#33503),
(#33504,#33505),(#33506,#33507),(#33508,#33509),(#33510,#33511),(#33512,
#33513),(#33514,#33515),(#33516,#33517),(#33518,#33519),(#33520,#33521),
(#33522,#33523),(#33524,#33525),(#33526,#33527),(#33528,#33529),(#33530,
#33531),(#33532,#33533),(#33534,#33535),(#33536,#33537)),.UNSPECIFIED.,
 .F.,.F.,.F.)
B_SPLINE_SURFACE_WITH_KNOTS((6,1,1,1,1,1,1,1,1,1,1,1,1,1,1,1,1,1,1,1,1,
1,1,1,1,1,1,1,1,1,1,1,1,1,1,1,1,1,1,1,1,1,1,1,1,1,1,1,1,1,1,1,1,1,1,1,1,
1,1,1,1,1,1,1,1,6),(2,2),(-1.,-0.984615384615383,-0.969230769230768,-0.953846153846152,
-0.938461538461537,-0.923076923076922,-0.907692307692306,-0.892307692307691,
-0.876923076923076,-0.86153846153846,-0.846153846153845,-0.83076923076923,
-0.815384615384614,-0.799999999999999,-0.784615384615384,-0.769230769230768,
-0.753846153846153,-0.738461538461538,-0.723076923076922,-0.707692307692307,
-0.692307692307692,-0.676923076923076,-0.661538461538461,-0.646153846153846,
-0.63076923076923,-0.615384615384615,-0.6,-0.584615384615384,-0.569230769230769,
-0.553846153846154,-0.538461538461538,-0.523076923076923,-0.507692307692308,
-0.492307692307692,-0.476923076923077,-0.461538461538462,-0.446153846153846,
-0.430769230769231,-0.415384615384615,-0.4,-0.384615384615385,-0.369230769230769,
-0.353846153846154,-0.338461538461538,-0.323076923076923,-0.307692307692308,
-0.292307692307692,-0.276923076923077,-0.261538461538462,-0.246153846153846,
-0.230769230769231,-0.215384615384615,-0.2,-0.184615384615385,-0.169230769230769,
-0.153846153846154,-0.138461538461538,-0.123076923076923,-0.107692307692308,
-0.0923076923076923,-0.0769230769230769,-0.0615384615384615,-0.0461538461538462,
-0.0307692307692308,-0.0153846153846154,0.),(-1.,1.),.UNSPECIFIED.)
GEOMETRIC_REPRESENTATION_ITEM()
RATIONAL_B_SPLINE_SURFACE(((1.,1.),(1.,1.),(1.,1.),(1.,1.),(1.,1.),(1.,
1.),(1.,1.),(1.,1.),(1.,1.),(1.,1.),(1.,1.),(1.,1.),(1.,1.),(1.,1.),(1.,
1.),(1.,1.),(1.,1.),(1.,1.),(1.,1.),(1.,1.),(1.,1.),(1.,1.),(1.,1.),(1.,
1.),(1.,1.),(1.,1.),(1.,1.),(1.,1.),(1.,1.),(1.,1.),(1.,1.),(1.,1.),(1.,
1.),(1.,1.),(1.,1.),(1.,1.),(1.,1.),(1.,1.),(1.,1.),(1.,1.),(1.,1.),(1.,
1.),(1.,1.),(1.,1.),(1.,1.),(1.,1.),(1.,1.),(1.,1.),(1.,1.),(1.,1.),(1.,
1.),(1.,1.),(1.,1.),(1.,1.),(1.,1.),(1.,1.),(1.,1.),(1.,1.),(1.,1.),(1.,
1.),(1.,1.),(1.,1.),(1.,1.),(1.,1.),(1.,1.),(1.,1.),(1.,1.),(1.,1.),(1.,
1.),(1.,1.)))
REPRESENTATION_ITEM('')
SURFACE()
);
#34=(
BOUNDED_SURFACE()
B_SPLINE_SURFACE(5,1,((#33614,#33615),(#33616,#33617),(#33618,#33619),(#33620,
#33621),(#33622,#33623),(#33624,#33625),(#33626,#33627),(#33628,#33629),
(#33630,#33631),(#33632,#33633),(#33634,#33635),(#33636,#33637),(#33638,
#33639),(#33640,#33641),(#33642,#33643),(#33644,#33645),(#33646,#33647),
(#33648,#33649),(#33650,#33651),(#33652,#33653),(#33654,#33655),(#33656,
#33657),(#33658,#33659),(#33660,#33661),(#33662,#33663),(#33664,#33665),
(#33666,#33667),(#33668,#33669),(#33670,#33671),(#33672,#33673),(#33674,
#33675),(#33676,#33677),(#33678,#33679),(#33680,#33681),(#33682,#33683),
(#33684,#33685),(#33686,#33687),(#33688,#33689),(#33690,#33691),(#33692,
#33693),(#33694,#33695),(#33696,#33697),(#33698,#33699),(#33700,#33701),
(#33702,#33703),(#33704,#33705),(#33706,#33707),(#33708,#33709),(#33710,
#33711),(#33712,#33713),(#33714,#33715),(#33716,#33717),(#33718,#33719),
(#33720,#33721),(#33722,#33723),(#33724,#33725),(#33726,#33727),(#33728,
#33729),(#33730,#33731),(#33732,#33733),(#33734,#33735),(#33736,#33737),
(#33738,#33739),(#33740,#33741),(#33742,#33743),(#33744,#33745),(#33746,
#33747),(#33748,#33749),(#33750,#33751),(#33752,#33753)),.UNSPECIFIED.,
 .F.,.F.,.F.)
B_SPLINE_SURFACE_WITH_KNOTS((6,1,1,1,1,1,1,1,1,1,1,1,1,1,1,1,1,1,1,1,1,
1,1,1,1,1,1,1,1,1,1,1,1,1,1,1,1,1,1,1,1,1,1,1,1,1,1,1,1,1,1,1,1,1,1,1,1,
1,1,1,1,1,1,1,1,6),(2,2),(-1.,-0.984615384615383,-0.969230769230768,-0.953846153846152,
-0.938461538461537,-0.923076923076922,-0.907692307692306,-0.892307692307691,
-0.876923076923076,-0.86153846153846,-0.846153846153845,-0.83076923076923,
-0.815384615384614,-0.799999999999999,-0.784615384615384,-0.769230769230768,
-0.753846153846153,-0.738461538461538,-0.723076923076922,-0.707692307692307,
-0.692307692307692,-0.676923076923076,-0.661538461538461,-0.646153846153846,
-0.63076923076923,-0.615384615384615,-0.6,-0.584615384615384,-0.569230769230769,
-0.553846153846154,-0.538461538461538,-0.523076923076923,-0.507692307692308,
-0.492307692307692,-0.476923076923077,-0.461538461538462,-0.446153846153846,
-0.430769230769231,-0.415384615384615,-0.4,-0.384615384615385,-0.369230769230769,
-0.353846153846154,-0.338461538461538,-0.323076923076923,-0.307692307692308,
-0.292307692307692,-0.276923076923077,-0.261538461538462,-0.246153846153846,
-0.230769230769231,-0.215384615384615,-0.2,-0.184615384615385,-0.169230769230769,
-0.153846153846154,-0.138461538461538,-0.123076923076923,-0.107692307692308,
-0.0923076923076923,-0.0769230769230769,-0.0615384615384615,-0.0461538461538462,
-0.0307692307692308,-0.0153846153846154,0.),(-1.,1.),.UNSPECIFIED.)
GEOMETRIC_REPRESENTATION_ITEM()
RATIONAL_B_SPLINE_SURFACE(((1.,1.),(1.,1.),(1.,1.),(1.,1.),(1.,1.),(1.,
1.),(1.,1.),(1.,1.),(1.,1.),(1.,1.),(1.,1.),(1.,1.),(1.,1.),(1.,1.),(1.,
1.),(1.,1.),(1.,1.),(1.,1.),(1.,1.),(1.,1.),(1.,1.),(1.,1.),(1.,1.),(1.,
1.),(1.,1.),(1.,1.),(1.,1.),(1.,1.),(1.,1.),(1.,1.),(1.,1.),(1.,1.),(1.,
1.),(1.,1.),(1.,1.),(1.,1.),(1.,1.),(1.,1.),(1.,1.),(1.,1.),(1.,1.),(1.,
1.),(1.,1.),(1.,1.),(1.,1.),(1.,1.),(1.,1.),(1.,1.),(1.,1.),(1.,1.),(1.,
1.),(1.,1.),(1.,1.),(1.,1.),(1.,1.),(1.,1.),(1.,1.),(1.,1.),(1.,1.),(1.,
1.),(1.,1.),(1.,1.),(1.,1.),(1.,1.),(1.,1.),(1.,1.),(1.,1.),(1.,1.),(1.,
1.),(1.,1.)))
REPRESENTATION_ITEM('')
SURFACE()
);
#35=(
BOUNDED_SURFACE()
B_SPLINE_SURFACE(5,1,((#33830,#33831),(#33832,#33833),(#33834,#33835),(#33836,
#33837),(#33838,#33839),(#33840,#33841),(#33842,#33843),(#33844,#33845),
(#33846,#33847),(#33848,#33849),(#33850,#33851),(#33852,#33853),(#33854,
#33855),(#33856,#33857),(#33858,#33859),(#33860,#33861),(#33862,#33863),
(#33864,#33865),(#33866,#33867),(#33868,#33869),(#33870,#33871),(#33872,
#33873),(#33874,#33875),(#33876,#33877),(#33878,#33879),(#33880,#33881),
(#33882,#33883),(#33884,#33885),(#33886,#33887),(#33888,#33889),(#33890,
#33891),(#33892,#33893),(#33894,#33895),(#33896,#33897),(#33898,#33899),
(#33900,#33901),(#33902,#33903),(#33904,#33905),(#33906,#33907),(#33908,
#33909),(#33910,#33911),(#33912,#33913),(#33914,#33915),(#33916,#33917),
(#33918,#33919),(#33920,#33921),(#33922,#33923),(#33924,#33925),(#33926,
#33927),(#33928,#33929),(#33930,#33931),(#33932,#33933),(#33934,#33935),
(#33936,#33937),(#33938,#33939),(#33940,#33941),(#33942,#33943),(#33944,
#33945),(#33946,#33947),(#33948,#33949),(#33950,#33951),(#33952,#33953),
(#33954,#33955),(#33956,#33957),(#33958,#33959),(#33960,#33961),(#33962,
#33963),(#33964,#33965),(#33966,#33967),(#33968,#33969)),.UNSPECIFIED.,
 .F.,.F.,.F.)
B_SPLINE_SURFACE_WITH_KNOTS((6,1,1,1,1,1,1,1,1,1,1,1,1,1,1,1,1,1,1,1,1,
1,1,1,1,1,1,1,1,1,1,1,1,1,1,1,1,1,1,1,1,1,1,1,1,1,1,1,1,1,1,1,1,1,1,1,1,
1,1,1,1,1,1,1,1,6),(2,2),(-1.,-0.984615384615383,-0.969230769230768,-0.953846153846152,
-0.938461538461537,-0.923076923076922,-0.907692307692306,-0.892307692307691,
-0.876923076923076,-0.86153846153846,-0.846153846153845,-0.83076923076923,
-0.815384615384614,-0.799999999999999,-0.784615384615384,-0.769230769230768,
-0.753846153846153,-0.738461538461538,-0.723076923076922,-0.707692307692307,
-0.692307692307692,-0.676923076923076,-0.661538461538461,-0.646153846153846,
-0.63076923076923,-0.615384615384615,-0.6,-0.584615384615384,-0.569230769230769,
-0.553846153846154,-0.538461538461538,-0.523076923076923,-0.507692307692308,
-0.492307692307692,-0.476923076923077,-0.461538461538462,-0.446153846153846,
-0.430769230769231,-0.415384615384615,-0.4,-0.384615384615385,-0.369230769230769,
-0.353846153846154,-0.338461538461538,-0.323076923076923,-0.307692307692308,
-0.292307692307692,-0.276923076923077,-0.261538461538462,-0.246153846153846,
-0.230769230769231,-0.215384615384615,-0.2,-0.184615384615385,-0.169230769230769,
-0.153846153846154,-0.138461538461538,-0.123076923076923,-0.107692307692308,
-0.0923076923076923,-0.0769230769230769,-0.0615384615384615,-0.0461538461538462,
-0.0307692307692308,-0.0153846153846154,0.),(-1.,1.),.UNSPECIFIED.)
GEOMETRIC_REPRESENTATION_ITEM()
RATIONAL_B_SPLINE_SURFACE(((1.,1.),(1.,1.),(1.,1.),(1.,1.),(1.,1.),(1.,
1.),(1.,1.),(1.,1.),(1.,1.),(1.,1.),(1.,1.),(1.,1.),(1.,1.),(1.,1.),(1.,
1.),(1.,1.),(1.,1.),(1.,1.),(1.,1.),(1.,1.),(1.,1.),(1.,1.),(1.,1.),(1.,
1.),(1.,1.),(1.,1.),(1.,1.),(1.,1.),(1.,1.),(1.,1.),(1.,1.),(1.,1.),(1.,
1.),(1.,1.),(1.,1.),(1.,1.),(1.,1.),(1.,1.),(1.,1.),(1.,1.),(1.,1.),(1.,
1.),(1.,1.),(1.,1.),(1.,1.),(1.,1.),(1.,1.),(1.,1.),(1.,1.),(1.,1.),(1.,
1.),(1.,1.),(1.,1.),(1.,1.),(1.,1.),(1.,1.),(1.,1.),(1.,1.),(1.,1.),(1.,
1.),(1.,1.),(1.,1.),(1.,1.),(1.,1.),(1.,1.),(1.,1.),(1.,1.),(1.,1.),(1.,
1.),(1.,1.)))
REPRESENTATION_ITEM('')
SURFACE()
);
#36=(
BOUNDED_SURFACE()
B_SPLINE_SURFACE(5,1,((#34046,#34047),(#34048,#34049),(#34050,#34051),(#34052,
#34053),(#34054,#34055),(#34056,#34057),(#34058,#34059),(#34060,#34061),
(#34062,#34063),(#34064,#34065),(#34066,#34067),(#34068,#34069),(#34070,
#34071),(#34072,#34073),(#34074,#34075),(#34076,#34077),(#34078,#34079),
(#34080,#34081),(#34082,#34083),(#34084,#34085),(#34086,#34087),(#34088,
#34089),(#34090,#34091),(#34092,#34093),(#34094,#34095),(#34096,#34097),
(#34098,#34099),(#34100,#34101),(#34102,#34103),(#34104,#34105),(#34106,
#34107),(#34108,#34109),(#34110,#34111),(#34112,#34113),(#34114,#34115),
(#34116,#34117),(#34118,#34119),(#34120,#34121),(#34122,#34123),(#34124,
#34125),(#34126,#34127),(#34128,#34129),(#34130,#34131),(#34132,#34133),
(#34134,#34135),(#34136,#34137),(#34138,#34139),(#34140,#34141),(#34142,
#34143),(#34144,#34145),(#34146,#34147),(#34148,#34149),(#34150,#34151),
(#34152,#34153),(#34154,#34155),(#34156,#34157),(#34158,#34159),(#34160,
#34161),(#34162,#34163),(#34164,#34165),(#34166,#34167),(#34168,#34169),
(#34170,#34171),(#34172,#34173),(#34174,#34175),(#34176,#34177),(#34178,
#34179),(#34180,#34181),(#34182,#34183),(#34184,#34185)),.UNSPECIFIED.,
 .F.,.F.,.F.)
B_SPLINE_SURFACE_WITH_KNOTS((6,1,1,1,1,1,1,1,1,1,1,1,1,1,1,1,1,1,1,1,1,
1,1,1,1,1,1,1,1,1,1,1,1,1,1,1,1,1,1,1,1,1,1,1,1,1,1,1,1,1,1,1,1,1,1,1,1,
1,1,1,1,1,1,1,1,6),(2,2),(-1.,-0.984615384615383,-0.969230769230768,-0.953846153846152,
-0.938461538461537,-0.923076923076922,-0.907692307692306,-0.892307692307691,
-0.876923076923076,-0.86153846153846,-0.846153846153845,-0.83076923076923,
-0.815384615384614,-0.799999999999999,-0.784615384615384,-0.769230769230768,
-0.753846153846153,-0.738461538461538,-0.723076923076922,-0.707692307692307,
-0.692307692307692,-0.676923076923076,-0.661538461538461,-0.646153846153846,
-0.63076923076923,-0.615384615384615,-0.6,-0.584615384615384,-0.569230769230769,
-0.553846153846154,-0.538461538461538,-0.523076923076923,-0.507692307692308,
-0.492307692307692,-0.476923076923077,-0.461538461538462,-0.446153846153846,
-0.430769230769231,-0.415384615384615,-0.4,-0.384615384615385,-0.369230769230769,
-0.353846153846154,-0.338461538461538,-0.323076923076923,-0.307692307692308,
-0.292307692307692,-0.276923076923077,-0.261538461538462,-0.246153846153846,
-0.230769230769231,-0.215384615384615,-0.2,-0.184615384615385,-0.169230769230769,
-0.153846153846154,-0.138461538461538,-0.123076923076923,-0.107692307692308,
-0.0923076923076923,-0.0769230769230769,-0.0615384615384615,-0.0461538461538462,
-0.0307692307692308,-0.0153846153846154,0.),(-1.,1.),.UNSPECIFIED.)
GEOMETRIC_REPRESENTATION_ITEM()
RATIONAL_B_SPLINE_SURFACE(((1.,1.),(1.,1.),(1.,1.),(1.,1.),(1.,1.),(1.,
1.),(1.,1.),(1.,1.),(1.,1.),(1.,1.),(1.,1.),(1.,1.),(1.,1.),(1.,1.),(1.,
1.),(1.,1.),(1.,1.),(1.,1.),(1.,1.),(1.,1.),(1.,1.),(1.,1.),(1.,1.),(1.,
1.),(1.,1.),(1.,1.),(1.,1.),(1.,1.),(1.,1.),(1.,1.),(1.,1.),(1.,1.),(1.,
1.),(1.,1.),(1.,1.),(1.,1.),(1.,1.),(1.,1.),(1.,1.),(1.,1.),(1.,1.),(1.,
1.),(1.,1.),(1.,1.),(1.,1.),(1.,1.),(1.,1.),(1.,1.),(1.,1.),(1.,1.),(1.,
1.),(1.,1.),(1.,1.),(1.,1.),(1.,1.),(1.,1.),(1.,1.),(1.,1.),(1.,1.),(1.,
1.),(1.,1.),(1.,1.),(1.,1.),(1.,1.),(1.,1.),(1.,1.),(1.,1.),(1.,1.),(1.,
1.),(1.,1.)))
REPRESENTATION_ITEM('')
SURFACE()
);
#37=(
BOUNDED_SURFACE()
B_SPLINE_SURFACE(5,1,((#34262,#34263),(#34264,#34265),(#34266,#34267),(#34268,
#34269),(#34270,#34271),(#34272,#34273),(#34274,#34275),(#34276,#34277),
(#34278,#34279),(#34280,#34281),(#34282,#34283),(#34284,#34285),(#34286,
#34287),(#34288,#34289),(#34290,#34291),(#34292,#34293),(#34294,#34295),
(#34296,#34297),(#34298,#34299),(#34300,#34301),(#34302,#34303),(#34304,
#34305),(#34306,#34307),(#34308,#34309),(#34310,#34311),(#34312,#34313),
(#34314,#34315),(#34316,#34317),(#34318,#34319),(#34320,#34321),(#34322,
#34323),(#34324,#34325),(#34326,#34327),(#34328,#34329),(#34330,#34331),
(#34332,#34333),(#34334,#34335),(#34336,#34337),(#34338,#34339),(#34340,
#34341),(#34342,#34343),(#34344,#34345),(#34346,#34347),(#34348,#34349),
(#34350,#34351),(#34352,#34353),(#34354,#34355),(#34356,#34357),(#34358,
#34359),(#34360,#34361),(#34362,#34363),(#34364,#34365),(#34366,#34367),
(#34368,#34369),(#34370,#34371),(#34372,#34373),(#34374,#34375),(#34376,
#34377),(#34378,#34379),(#34380,#34381),(#34382,#34383),(#34384,#34385),
(#34386,#34387),(#34388,#34389),(#34390,#34391),(#34392,#34393),(#34394,
#34395),(#34396,#34397),(#34398,#34399),(#34400,#34401)),.UNSPECIFIED.,
 .F.,.F.,.F.)
B_SPLINE_SURFACE_WITH_KNOTS((6,1,1,1,1,1,1,1,1,1,1,1,1,1,1,1,1,1,1,1,1,
1,1,1,1,1,1,1,1,1,1,1,1,1,1,1,1,1,1,1,1,1,1,1,1,1,1,1,1,1,1,1,1,1,1,1,1,
1,1,1,1,1,1,1,1,6),(2,2),(-1.,-0.984615384615383,-0.969230769230768,-0.953846153846152,
-0.938461538461537,-0.923076923076922,-0.907692307692306,-0.892307692307691,
-0.876923076923076,-0.86153846153846,-0.846153846153845,-0.83076923076923,
-0.815384615384614,-0.799999999999999,-0.784615384615384,-0.769230769230768,
-0.753846153846153,-0.738461538461538,-0.723076923076922,-0.707692307692307,
-0.692307692307692,-0.676923076923076,-0.661538461538461,-0.646153846153846,
-0.63076923076923,-0.615384615384615,-0.6,-0.584615384615384,-0.569230769230769,
-0.553846153846154,-0.538461538461538,-0.523076923076923,-0.507692307692308,
-0.492307692307692,-0.476923076923077,-0.461538461538462,-0.446153846153846,
-0.430769230769231,-0.415384615384615,-0.4,-0.384615384615385,-0.369230769230769,
-0.353846153846154,-0.338461538461538,-0.323076923076923,-0.307692307692308,
-0.292307692307692,-0.276923076923077,-0.261538461538462,-0.246153846153846,
-0.230769230769231,-0.215384615384615,-0.2,-0.184615384615385,-0.169230769230769,
-0.153846153846154,-0.138461538461538,-0.123076923076923,-0.107692307692308,
-0.0923076923076923,-0.0769230769230769,-0.0615384615384615,-0.0461538461538462,
-0.0307692307692308,-0.0153846153846154,0.),(-1.,1.),.UNSPECIFIED.)
GEOMETRIC_REPRESENTATION_ITEM()
RATIONAL_B_SPLINE_SURFACE(((1.,1.),(1.,1.),(1.,1.),(1.,1.),(1.,1.),(1.,
1.),(1.,1.),(1.,1.),(1.,1.),(1.,1.),(1.,1.),(1.,1.),(1.,1.),(1.,1.),(1.,
1.),(1.,1.),(1.,1.),(1.,1.),(1.,1.),(1.,1.),(1.,1.),(1.,1.),(1.,1.),(1.,
1.),(1.,1.),(1.,1.),(1.,1.),(1.,1.),(1.,1.),(1.,1.),(1.,1.),(1.,1.),(1.,
1.),(1.,1.),(1.,1.),(1.,1.),(1.,1.),(1.,1.),(1.,1.),(1.,1.),(1.,1.),(1.,
1.),(1.,1.),(1.,1.),(1.,1.),(1.,1.),(1.,1.),(1.,1.),(1.,1.),(1.,1.),(1.,
1.),(1.,1.),(1.,1.),(1.,1.),(1.,1.),(1.,1.),(1.,1.),(1.,1.),(1.,1.),(1.,
1.),(1.,1.),(1.,1.),(1.,1.),(1.,1.),(1.,1.),(1.,1.),(1.,1.),(1.,1.),(1.,
1.),(1.,1.)))
REPRESENTATION_ITEM('')
SURFACE()
);
#38=(
BOUNDED_SURFACE()
B_SPLINE_SURFACE(5,1,((#34478,#34479),(#34480,#34481),(#34482,#34483),(#34484,
#34485),(#34486,#34487),(#34488,#34489),(#34490,#34491),(#34492,#34493),
(#34494,#34495),(#34496,#34497),(#34498,#34499),(#34500,#34501),(#34502,
#34503),(#34504,#34505),(#34506,#34507),(#34508,#34509),(#34510,#34511),
(#34512,#34513),(#34514,#34515),(#34516,#34517),(#34518,#34519),(#34520,
#34521),(#34522,#34523),(#34524,#34525),(#34526,#34527),(#34528,#34529),
(#34530,#34531),(#34532,#34533),(#34534,#34535),(#34536,#34537),(#34538,
#34539),(#34540,#34541),(#34542,#34543),(#34544,#34545),(#34546,#34547),
(#34548,#34549),(#34550,#34551),(#34552,#34553),(#34554,#34555),(#34556,
#34557),(#34558,#34559),(#34560,#34561),(#34562,#34563),(#34564,#34565),
(#34566,#34567),(#34568,#34569),(#34570,#34571),(#34572,#34573),(#34574,
#34575),(#34576,#34577),(#34578,#34579),(#34580,#34581),(#34582,#34583),
(#34584,#34585),(#34586,#34587),(#34588,#34589),(#34590,#34591),(#34592,
#34593),(#34594,#34595),(#34596,#34597),(#34598,#34599),(#34600,#34601),
(#34602,#34603),(#34604,#34605),(#34606,#34607),(#34608,#34609),(#34610,
#34611),(#34612,#34613),(#34614,#34615),(#34616,#34617)),.UNSPECIFIED.,
 .F.,.F.,.F.)
B_SPLINE_SURFACE_WITH_KNOTS((6,1,1,1,1,1,1,1,1,1,1,1,1,1,1,1,1,1,1,1,1,
1,1,1,1,1,1,1,1,1,1,1,1,1,1,1,1,1,1,1,1,1,1,1,1,1,1,1,1,1,1,1,1,1,1,1,1,
1,1,1,1,1,1,1,1,6),(2,2),(-1.,-0.984615384615383,-0.969230769230768,-0.953846153846152,
-0.938461538461537,-0.923076923076922,-0.907692307692306,-0.892307692307691,
-0.876923076923076,-0.86153846153846,-0.846153846153845,-0.83076923076923,
-0.815384615384614,-0.799999999999999,-0.784615384615384,-0.769230769230768,
-0.753846153846153,-0.738461538461538,-0.723076923076922,-0.707692307692307,
-0.692307692307692,-0.676923076923076,-0.661538461538461,-0.646153846153846,
-0.63076923076923,-0.615384615384615,-0.6,-0.584615384615384,-0.569230769230769,
-0.553846153846154,-0.538461538461538,-0.523076923076923,-0.507692307692308,
-0.492307692307692,-0.476923076923077,-0.461538461538462,-0.446153846153846,
-0.430769230769231,-0.415384615384615,-0.4,-0.384615384615385,-0.369230769230769,
-0.353846153846154,-0.338461538461538,-0.323076923076923,-0.307692307692308,
-0.292307692307692,-0.276923076923077,-0.261538461538462,-0.246153846153846,
-0.230769230769231,-0.215384615384615,-0.2,-0.184615384615385,-0.169230769230769,
-0.153846153846154,-0.138461538461538,-0.123076923076923,-0.107692307692308,
-0.0923076923076923,-0.0769230769230769,-0.0615384615384615,-0.0461538461538462,
-0.0307692307692308,-0.0153846153846154,0.),(-1.,1.),.UNSPECIFIED.)
GEOMETRIC_REPRESENTATION_ITEM()
RATIONAL_B_SPLINE_SURFACE(((1.,1.),(1.,1.),(1.,1.),(1.,1.),(1.,1.),(1.,
1.),(1.,1.),(1.,1.),(1.,1.),(1.,1.),(1.,1.),(1.,1.),(1.,1.),(1.,1.),(1.,
1.),(1.,1.),(1.,1.),(1.,1.),(1.,1.),(1.,1.),(1.,1.),(1.,1.),(1.,1.),(1.,
1.),(1.,1.),(1.,1.),(1.,1.),(1.,1.),(1.,1.),(1.,1.),(1.,1.),(1.,1.),(1.,
1.),(1.,1.),(1.,1.),(1.,1.),(1.,1.),(1.,1.),(1.,1.),(1.,1.),(1.,1.),(1.,
1.),(1.,1.),(1.,1.),(1.,1.),(1.,1.),(1.,1.),(1.,1.),(1.,1.),(1.,1.),(1.,
1.),(1.,1.),(1.,1.),(1.,1.),(1.,1.),(1.,1.),(1.,1.),(1.,1.),(1.,1.),(1.,
1.),(1.,1.),(1.,1.),(1.,1.),(1.,1.),(1.,1.),(1.,1.),(1.,1.),(1.,1.),(1.,
1.),(1.,1.)))
REPRESENTATION_ITEM('')
SURFACE()
);
#39=(
BOUNDED_SURFACE()
B_SPLINE_SURFACE(5,1,((#34694,#34695),(#34696,#34697),(#34698,#34699),(#34700,
#34701),(#34702,#34703),(#34704,#34705),(#34706,#34707),(#34708,#34709),
(#34710,#34711),(#34712,#34713),(#34714,#34715),(#34716,#34717),(#34718,
#34719),(#34720,#34721),(#34722,#34723),(#34724,#34725),(#34726,#34727),
(#34728,#34729),(#34730,#34731),(#34732,#34733),(#34734,#34735),(#34736,
#34737),(#34738,#34739),(#34740,#34741),(#34742,#34743),(#34744,#34745),
(#34746,#34747),(#34748,#34749),(#34750,#34751),(#34752,#34753),(#34754,
#34755),(#34756,#34757),(#34758,#34759),(#34760,#34761),(#34762,#34763),
(#34764,#34765),(#34766,#34767),(#34768,#34769),(#34770,#34771),(#34772,
#34773),(#34774,#34775),(#34776,#34777),(#34778,#34779),(#34780,#34781),
(#34782,#34783),(#34784,#34785),(#34786,#34787),(#34788,#34789),(#34790,
#34791),(#34792,#34793),(#34794,#34795),(#34796,#34797),(#34798,#34799),
(#34800,#34801),(#34802,#34803),(#34804,#34805),(#34806,#34807),(#34808,
#34809),(#34810,#34811),(#34812,#34813),(#34814,#34815),(#34816,#34817),
(#34818,#34819),(#34820,#34821),(#34822,#34823),(#34824,#34825),(#34826,
#34827),(#34828,#34829),(#34830,#34831),(#34832,#34833)),.UNSPECIFIED.,
 .F.,.F.,.F.)
B_SPLINE_SURFACE_WITH_KNOTS((6,1,1,1,1,1,1,1,1,1,1,1,1,1,1,1,1,1,1,1,1,
1,1,1,1,1,1,1,1,1,1,1,1,1,1,1,1,1,1,1,1,1,1,1,1,1,1,1,1,1,1,1,1,1,1,1,1,
1,1,1,1,1,1,1,1,6),(2,2),(-1.,-0.984615384615383,-0.969230769230768,-0.953846153846152,
-0.938461538461537,-0.923076923076922,-0.907692307692306,-0.892307692307691,
-0.876923076923076,-0.86153846153846,-0.846153846153845,-0.83076923076923,
-0.815384615384614,-0.799999999999999,-0.784615384615384,-0.769230769230768,
-0.753846153846153,-0.738461538461538,-0.723076923076922,-0.707692307692307,
-0.692307692307692,-0.676923076923076,-0.661538461538461,-0.646153846153846,
-0.63076923076923,-0.615384615384615,-0.6,-0.584615384615384,-0.569230769230769,
-0.553846153846154,-0.538461538461538,-0.523076923076923,-0.507692307692308,
-0.492307692307692,-0.476923076923077,-0.461538461538462,-0.446153846153846,
-0.430769230769231,-0.415384615384615,-0.4,-0.384615384615385,-0.369230769230769,
-0.353846153846154,-0.338461538461538,-0.323076923076923,-0.307692307692308,
-0.292307692307692,-0.276923076923077,-0.261538461538462,-0.246153846153846,
-0.230769230769231,-0.215384615384615,-0.2,-0.184615384615385,-0.169230769230769,
-0.153846153846154,-0.138461538461538,-0.123076923076923,-0.107692307692308,
-0.0923076923076923,-0.0769230769230769,-0.0615384615384615,-0.0461538461538462,
-0.0307692307692308,-0.0153846153846154,0.),(-1.,1.),.UNSPECIFIED.)
GEOMETRIC_REPRESENTATION_ITEM()
RATIONAL_B_SPLINE_SURFACE(((1.,1.),(1.,1.),(1.,1.),(1.,1.),(1.,1.),(1.,
1.),(1.,1.),(1.,1.),(1.,1.),(1.,1.),(1.,1.),(1.,1.),(1.,1.),(1.,1.),(1.,
1.),(1.,1.),(1.,1.),(1.,1.),(1.,1.),(1.,1.),(1.,1.),(1.,1.),(1.,1.),(1.,
1.),(1.,1.),(1.,1.),(1.,1.),(1.,1.),(1.,1.),(1.,1.),(1.,1.),(1.,1.),(1.,
1.),(1.,1.),(1.,1.),(1.,1.),(1.,1.),(1.,1.),(1.,1.),(1.,1.),(1.,1.),(1.,
1.),(1.,1.),(1.,1.),(1.,1.),(1.,1.),(1.,1.),(1.,1.),(1.,1.),(1.,1.),(1.,
1.),(1.,1.),(1.,1.),(1.,1.),(1.,1.),(1.,1.),(1.,1.),(1.,1.),(1.,1.),(1.,
1.),(1.,1.),(1.,1.),(1.,1.),(1.,1.),(1.,1.),(1.,1.),(1.,1.),(1.,1.),(1.,
1.),(1.,1.)))
REPRESENTATION_ITEM('')
SURFACE()
);
#40=(
BOUNDED_SURFACE()
B_SPLINE_SURFACE(5,1,((#34910,#34911),(#34912,#34913),(#34914,#34915),(#34916,
#34917),(#34918,#34919),(#34920,#34921),(#34922,#34923),(#34924,#34925),
(#34926,#34927),(#34928,#34929),(#34930,#34931),(#34932,#34933),(#34934,
#34935),(#34936,#34937),(#34938,#34939),(#34940,#34941),(#34942,#34943),
(#34944,#34945),(#34946,#34947),(#34948,#34949),(#34950,#34951),(#34952,
#34953),(#34954,#34955),(#34956,#34957),(#34958,#34959),(#34960,#34961),
(#34962,#34963),(#34964,#34965),(#34966,#34967),(#34968,#34969),(#34970,
#34971),(#34972,#34973),(#34974,#34975),(#34976,#34977),(#34978,#34979),
(#34980,#34981),(#34982,#34983),(#34984,#34985),(#34986,#34987),(#34988,
#34989),(#34990,#34991),(#34992,#34993),(#34994,#34995),(#34996,#34997),
(#34998,#34999),(#35000,#35001),(#35002,#35003),(#35004,#35005),(#35006,
#35007),(#35008,#35009),(#35010,#35011),(#35012,#35013),(#35014,#35015),
(#35016,#35017),(#35018,#35019),(#35020,#35021),(#35022,#35023),(#35024,
#35025),(#35026,#35027),(#35028,#35029),(#35030,#35031),(#35032,#35033),
(#35034,#35035),(#35036,#35037),(#35038,#35039),(#35040,#35041),(#35042,
#35043),(#35044,#35045),(#35046,#35047),(#35048,#35049)),.UNSPECIFIED.,
 .F.,.F.,.F.)
B_SPLINE_SURFACE_WITH_KNOTS((6,1,1,1,1,1,1,1,1,1,1,1,1,1,1,1,1,1,1,1,1,
1,1,1,1,1,1,1,1,1,1,1,1,1,1,1,1,1,1,1,1,1,1,1,1,1,1,1,1,1,1,1,1,1,1,1,1,
1,1,1,1,1,1,1,1,6),(2,2),(-1.,-0.984615384615383,-0.969230769230768,-0.953846153846152,
-0.938461538461537,-0.923076923076922,-0.907692307692306,-0.892307692307691,
-0.876923076923076,-0.86153846153846,-0.846153846153845,-0.83076923076923,
-0.815384615384614,-0.799999999999999,-0.784615384615384,-0.769230769230768,
-0.753846153846153,-0.738461538461538,-0.723076923076922,-0.707692307692307,
-0.692307692307692,-0.676923076923076,-0.661538461538461,-0.646153846153846,
-0.63076923076923,-0.615384615384615,-0.6,-0.584615384615384,-0.569230769230769,
-0.553846153846154,-0.538461538461538,-0.523076923076923,-0.507692307692308,
-0.492307692307692,-0.476923076923077,-0.461538461538462,-0.446153846153846,
-0.430769230769231,-0.415384615384615,-0.4,-0.384615384615385,-0.369230769230769,
-0.353846153846154,-0.338461538461538,-0.323076923076923,-0.307692307692308,
-0.292307692307692,-0.276923076923077,-0.261538461538462,-0.246153846153846,
-0.230769230769231,-0.215384615384615,-0.2,-0.184615384615385,-0.169230769230769,
-0.153846153846154,-0.138461538461538,-0.123076923076923,-0.107692307692308,
-0.0923076923076923,-0.0769230769230769,-0.0615384615384615,-0.0461538461538462,
-0.0307692307692308,-0.0153846153846154,0.),(-1.,1.),.UNSPECIFIED.)
GEOMETRIC_REPRESENTATION_ITEM()
RATIONAL_B_SPLINE_SURFACE(((1.,1.),(1.,1.),(1.,1.),(1.,1.),(1.,1.),(1.,
1.),(1.,1.),(1.,1.),(1.,1.),(1.,1.),(1.,1.),(1.,1.),(1.,1.),(1.,1.),(1.,
1.),(1.,1.),(1.,1.),(1.,1.),(1.,1.),(1.,1.),(1.,1.),(1.,1.),(1.,1.),(1.,
1.),(1.,1.),(1.,1.),(1.,1.),(1.,1.),(1.,1.),(1.,1.),(1.,1.),(1.,1.),(1.,
1.),(1.,1.),(1.,1.),(1.,1.),(1.,1.),(1.,1.),(1.,1.),(1.,1.),(1.,1.),(1.,
1.),(1.,1.),(1.,1.),(1.,1.),(1.,1.),(1.,1.),(1.,1.),(1.,1.),(1.,1.),(1.,
1.),(1.,1.),(1.,1.),(1.,1.),(1.,1.),(1.,1.),(1.,1.),(1.,1.),(1.,1.),(1.,
1.),(1.,1.),(1.,1.),(1.,1.),(1.,1.),(1.,1.),(1.,1.),(1.,1.),(1.,1.),(1.,
1.),(1.,1.)))
REPRESENTATION_ITEM('')
SURFACE()
);
#41=(
BOUNDED_SURFACE()
B_SPLINE_SURFACE(5,1,((#35126,#35127),(#35128,#35129),(#35130,#35131),(#35132,
#35133),(#35134,#35135),(#35136,#35137),(#35138,#35139),(#35140,#35141),
(#35142,#35143),(#35144,#35145),(#35146,#35147),(#35148,#35149),(#35150,
#35151),(#35152,#35153),(#35154,#35155),(#35156,#35157),(#35158,#35159),
(#35160,#35161),(#35162,#35163),(#35164,#35165),(#35166,#35167),(#35168,
#35169),(#35170,#35171),(#35172,#35173),(#35174,#35175),(#35176,#35177),
(#35178,#35179),(#35180,#35181),(#35182,#35183),(#35184,#35185),(#35186,
#35187),(#35188,#35189),(#35190,#35191),(#35192,#35193),(#35194,#35195),
(#35196,#35197),(#35198,#35199),(#35200,#35201),(#35202,#35203),(#35204,
#35205),(#35206,#35207),(#35208,#35209),(#35210,#35211),(#35212,#35213),
(#35214,#35215),(#35216,#35217),(#35218,#35219),(#35220,#35221),(#35222,
#35223),(#35224,#35225),(#35226,#35227),(#35228,#35229),(#35230,#35231),
(#35232,#35233),(#35234,#35235),(#35236,#35237),(#35238,#35239),(#35240,
#35241),(#35242,#35243),(#35244,#35245),(#35246,#35247),(#35248,#35249),
(#35250,#35251),(#35252,#35253),(#35254,#35255),(#35256,#35257),(#35258,
#35259),(#35260,#35261),(#35262,#35263),(#35264,#35265)),.UNSPECIFIED.,
 .F.,.F.,.F.)
B_SPLINE_SURFACE_WITH_KNOTS((6,1,1,1,1,1,1,1,1,1,1,1,1,1,1,1,1,1,1,1,1,
1,1,1,1,1,1,1,1,1,1,1,1,1,1,1,1,1,1,1,1,1,1,1,1,1,1,1,1,1,1,1,1,1,1,1,1,
1,1,1,1,1,1,1,1,6),(2,2),(-1.,-0.984615384615383,-0.969230769230768,-0.953846153846152,
-0.938461538461537,-0.923076923076922,-0.907692307692306,-0.892307692307691,
-0.876923076923076,-0.86153846153846,-0.846153846153845,-0.83076923076923,
-0.815384615384614,-0.799999999999999,-0.784615384615384,-0.769230769230768,
-0.753846153846153,-0.738461538461538,-0.723076923076922,-0.707692307692307,
-0.692307692307692,-0.676923076923076,-0.661538461538461,-0.646153846153846,
-0.63076923076923,-0.615384615384615,-0.6,-0.584615384615384,-0.569230769230769,
-0.553846153846154,-0.538461538461538,-0.523076923076923,-0.507692307692308,
-0.492307692307692,-0.476923076923077,-0.461538461538462,-0.446153846153846,
-0.430769230769231,-0.415384615384615,-0.4,-0.384615384615385,-0.369230769230769,
-0.353846153846154,-0.338461538461538,-0.323076923076923,-0.307692307692308,
-0.292307692307692,-0.276923076923077,-0.261538461538462,-0.246153846153846,
-0.230769230769231,-0.215384615384615,-0.2,-0.184615384615385,-0.169230769230769,
-0.153846153846154,-0.138461538461538,-0.123076923076923,-0.107692307692308,
-0.0923076923076923,-0.0769230769230769,-0.0615384615384615,-0.0461538461538462,
-0.0307692307692308,-0.0153846153846154,0.),(-1.,1.),.UNSPECIFIED.)
GEOMETRIC_REPRESENTATION_ITEM()
RATIONAL_B_SPLINE_SURFACE(((1.,1.),(1.,1.),(1.,1.),(1.,1.),(1.,1.),(1.,
1.),(1.,1.),(1.,1.),(1.,1.),(1.,1.),(1.,1.),(1.,1.),(1.,1.),(1.,1.),(1.,
1.),(1.,1.),(1.,1.),(1.,1.),(1.,1.),(1.,1.),(1.,1.),(1.,1.),(1.,1.),(1.,
1.),(1.,1.),(1.,1.),(1.,1.),(1.,1.),(1.,1.),(1.,1.),(1.,1.),(1.,1.),(1.,
1.),(1.,1.),(1.,1.),(1.,1.),(1.,1.),(1.,1.),(1.,1.),(1.,1.),(1.,1.),(1.,
1.),(1.,1.),(1.,1.),(1.,1.),(1.,1.),(1.,1.),(1.,1.),(1.,1.),(1.,1.),(1.,
1.),(1.,1.),(1.,1.),(1.,1.),(1.,1.),(1.,1.),(1.,1.),(1.,1.),(1.,1.),(1.,
1.),(1.,1.),(1.,1.),(1.,1.),(1.,1.),(1.,1.),(1.,1.),(1.,1.),(1.,1.),(1.,
1.),(1.,1.)))
REPRESENTATION_ITEM('')
SURFACE()
);
#42=(
BOUNDED_SURFACE()
B_SPLINE_SURFACE(5,1,((#35342,#35343),(#35344,#35345),(#35346,#35347),(#35348,
#35349),(#35350,#35351),(#35352,#35353),(#35354,#35355),(#35356,#35357),
(#35358,#35359),(#35360,#35361),(#35362,#35363),(#35364,#35365),(#35366,
#35367),(#35368,#35369),(#35370,#35371),(#35372,#35373),(#35374,#35375),
(#35376,#35377),(#35378,#35379),(#35380,#35381),(#35382,#35383),(#35384,
#35385),(#35386,#35387),(#35388,#35389),(#35390,#35391),(#35392,#35393),
(#35394,#35395),(#35396,#35397),(#35398,#35399),(#35400,#35401),(#35402,
#35403),(#35404,#35405),(#35406,#35407),(#35408,#35409),(#35410,#35411),
(#35412,#35413),(#35414,#35415),(#35416,#35417),(#35418,#35419),(#35420,
#35421),(#35422,#35423),(#35424,#35425),(#35426,#35427),(#35428,#35429),
(#35430,#35431),(#35432,#35433),(#35434,#35435),(#35436,#35437),(#35438,
#35439),(#35440,#35441),(#35442,#35443),(#35444,#35445),(#35446,#35447),
(#35448,#35449),(#35450,#35451),(#35452,#35453),(#35454,#35455),(#35456,
#35457),(#35458,#35459),(#35460,#35461),(#35462,#35463),(#35464,#35465),
(#35466,#35467),(#35468,#35469),(#35470,#35471),(#35472,#35473),(#35474,
#35475),(#35476,#35477),(#35478,#35479),(#35480,#35481)),.UNSPECIFIED.,
 .F.,.F.,.F.)
B_SPLINE_SURFACE_WITH_KNOTS((6,1,1,1,1,1,1,1,1,1,1,1,1,1,1,1,1,1,1,1,1,
1,1,1,1,1,1,1,1,1,1,1,1,1,1,1,1,1,1,1,1,1,1,1,1,1,1,1,1,1,1,1,1,1,1,1,1,
1,1,1,1,1,1,1,1,6),(2,2),(-1.,-0.984615384615383,-0.969230769230768,-0.953846153846152,
-0.938461538461537,-0.923076923076922,-0.907692307692306,-0.892307692307691,
-0.876923076923076,-0.86153846153846,-0.846153846153845,-0.83076923076923,
-0.815384615384614,-0.799999999999999,-0.784615384615384,-0.769230769230768,
-0.753846153846153,-0.738461538461538,-0.723076923076922,-0.707692307692307,
-0.692307692307692,-0.676923076923076,-0.661538461538461,-0.646153846153846,
-0.63076923076923,-0.615384615384615,-0.6,-0.584615384615384,-0.569230769230769,
-0.553846153846154,-0.538461538461538,-0.523076923076923,-0.507692307692308,
-0.492307692307692,-0.476923076923077,-0.461538461538462,-0.446153846153846,
-0.430769230769231,-0.415384615384615,-0.4,-0.384615384615385,-0.369230769230769,
-0.353846153846154,-0.338461538461538,-0.323076923076923,-0.307692307692308,
-0.292307692307692,-0.276923076923077,-0.261538461538462,-0.246153846153846,
-0.230769230769231,-0.215384615384615,-0.2,-0.184615384615385,-0.169230769230769,
-0.153846153846154,-0.138461538461538,-0.123076923076923,-0.107692307692308,
-0.0923076923076923,-0.0769230769230769,-0.0615384615384615,-0.0461538461538462,
-0.0307692307692308,-0.0153846153846154,0.),(-1.,1.),.UNSPECIFIED.)
GEOMETRIC_REPRESENTATION_ITEM()
RATIONAL_B_SPLINE_SURFACE(((1.,1.),(1.,1.),(1.,1.),(1.,1.),(1.,1.),(1.,
1.),(1.,1.),(1.,1.),(1.,1.),(1.,1.),(1.,1.),(1.,1.),(1.,1.),(1.,1.),(1.,
1.),(1.,1.),(1.,1.),(1.,1.),(1.,1.),(1.,1.),(1.,1.),(1.,1.),(1.,1.),(1.,
1.),(1.,1.),(1.,1.),(1.,1.),(1.,1.),(1.,1.),(1.,1.),(1.,1.),(1.,1.),(1.,
1.),(1.,1.),(1.,1.),(1.,1.),(1.,1.),(1.,1.),(1.,1.),(1.,1.),(1.,1.),(1.,
1.),(1.,1.),(1.,1.),(1.,1.),(1.,1.),(1.,1.),(1.,1.),(1.,1.),(1.,1.),(1.,
1.),(1.,1.),(1.,1.),(1.,1.),(1.,1.),(1.,1.),(1.,1.),(1.,1.),(1.,1.),(1.,
1.),(1.,1.),(1.,1.),(1.,1.),(1.,1.),(1.,1.),(1.,1.),(1.,1.),(1.,1.),(1.,
1.),(1.,1.)))
REPRESENTATION_ITEM('')
SURFACE()
);
#43=(
BOUNDED_SURFACE()
B_SPLINE_SURFACE(5,1,((#35558,#35559),(#35560,#35561),(#35562,#35563),(#35564,
#35565),(#35566,#35567),(#35568,#35569),(#35570,#35571),(#35572,#35573),
(#35574,#35575),(#35576,#35577),(#35578,#35579),(#35580,#35581),(#35582,
#35583),(#35584,#35585),(#35586,#35587),(#35588,#35589),(#35590,#35591),
(#35592,#35593),(#35594,#35595),(#35596,#35597),(#35598,#35599),(#35600,
#35601),(#35602,#35603),(#35604,#35605),(#35606,#35607),(#35608,#35609),
(#35610,#35611),(#35612,#35613),(#35614,#35615),(#35616,#35617),(#35618,
#35619),(#35620,#35621),(#35622,#35623),(#35624,#35625),(#35626,#35627),
(#35628,#35629),(#35630,#35631),(#35632,#35633),(#35634,#35635),(#35636,
#35637),(#35638,#35639),(#35640,#35641),(#35642,#35643),(#35644,#35645),
(#35646,#35647),(#35648,#35649),(#35650,#35651),(#35652,#35653),(#35654,
#35655),(#35656,#35657),(#35658,#35659),(#35660,#35661),(#35662,#35663),
(#35664,#35665),(#35666,#35667),(#35668,#35669),(#35670,#35671),(#35672,
#35673),(#35674,#35675),(#35676,#35677),(#35678,#35679),(#35680,#35681),
(#35682,#35683),(#35684,#35685),(#35686,#35687),(#35688,#35689),(#35690,
#35691),(#35692,#35693),(#35694,#35695),(#35696,#35697)),.UNSPECIFIED.,
 .F.,.F.,.F.)
B_SPLINE_SURFACE_WITH_KNOTS((6,1,1,1,1,1,1,1,1,1,1,1,1,1,1,1,1,1,1,1,1,
1,1,1,1,1,1,1,1,1,1,1,1,1,1,1,1,1,1,1,1,1,1,1,1,1,1,1,1,1,1,1,1,1,1,1,1,
1,1,1,1,1,1,1,1,6),(2,2),(-1.,-0.984615384615383,-0.969230769230768,-0.953846153846152,
-0.938461538461537,-0.923076923076922,-0.907692307692306,-0.892307692307691,
-0.876923076923076,-0.86153846153846,-0.846153846153845,-0.83076923076923,
-0.815384615384614,-0.799999999999999,-0.784615384615384,-0.769230769230768,
-0.753846153846153,-0.738461538461538,-0.723076923076922,-0.707692307692307,
-0.692307692307692,-0.676923076923076,-0.661538461538461,-0.646153846153846,
-0.63076923076923,-0.615384615384615,-0.6,-0.584615384615384,-0.569230769230769,
-0.553846153846154,-0.538461538461538,-0.523076923076923,-0.507692307692308,
-0.492307692307692,-0.476923076923077,-0.461538461538462,-0.446153846153846,
-0.430769230769231,-0.415384615384615,-0.4,-0.384615384615385,-0.369230769230769,
-0.353846153846154,-0.338461538461538,-0.323076923076923,-0.307692307692308,
-0.292307692307692,-0.276923076923077,-0.261538461538462,-0.246153846153846,
-0.230769230769231,-0.215384615384615,-0.2,-0.184615384615385,-0.169230769230769,
-0.153846153846154,-0.138461538461538,-0.123076923076923,-0.107692307692308,
-0.0923076923076923,-0.0769230769230769,-0.0615384615384615,-0.0461538461538462,
-0.0307692307692308,-0.0153846153846154,0.),(-1.,1.),.UNSPECIFIED.)
GEOMETRIC_REPRESENTATION_ITEM()
RATIONAL_B_SPLINE_SURFACE(((1.,1.),(1.,1.),(1.,1.),(1.,1.),(1.,1.),(1.,
1.),(1.,1.),(1.,1.),(1.,1.),(1.,1.),(1.,1.),(1.,1.),(1.,1.),(1.,1.),(1.,
1.),(1.,1.),(1.,1.),(1.,1.),(1.,1.),(1.,1.),(1.,1.),(1.,1.),(1.,1.),(1.,
1.),(1.,1.),(1.,1.),(1.,1.),(1.,1.),(1.,1.),(1.,1.),(1.,1.),(1.,1.),(1.,
1.),(1.,1.),(1.,1.),(1.,1.),(1.,1.),(1.,1.),(1.,1.),(1.,1.),(1.,1.),(1.,
1.),(1.,1.),(1.,1.),(1.,1.),(1.,1.),(1.,1.),(1.,1.),(1.,1.),(1.,1.),(1.,
1.),(1.,1.),(1.,1.),(1.,1.),(1.,1.),(1.,1.),(1.,1.),(1.,1.),(1.,1.),(1.,
1.),(1.,1.),(1.,1.),(1.,1.),(1.,1.),(1.,1.),(1.,1.),(1.,1.),(1.,1.),(1.,
1.),(1.,1.)))
REPRESENTATION_ITEM('')
SURFACE()
);
#44=(
BOUNDED_SURFACE()
B_SPLINE_SURFACE(5,1,((#35774,#35775),(#35776,#35777),(#35778,#35779),(#35780,
#35781),(#35782,#35783),(#35784,#35785),(#35786,#35787),(#35788,#35789),
(#35790,#35791),(#35792,#35793),(#35794,#35795),(#35796,#35797),(#35798,
#35799),(#35800,#35801),(#35802,#35803),(#35804,#35805),(#35806,#35807),
(#35808,#35809),(#35810,#35811),(#35812,#35813),(#35814,#35815),(#35816,
#35817),(#35818,#35819),(#35820,#35821),(#35822,#35823),(#35824,#35825),
(#35826,#35827),(#35828,#35829),(#35830,#35831),(#35832,#35833),(#35834,
#35835),(#35836,#35837),(#35838,#35839),(#35840,#35841),(#35842,#35843),
(#35844,#35845),(#35846,#35847),(#35848,#35849),(#35850,#35851),(#35852,
#35853),(#35854,#35855),(#35856,#35857),(#35858,#35859),(#35860,#35861),
(#35862,#35863),(#35864,#35865),(#35866,#35867),(#35868,#35869),(#35870,
#35871),(#35872,#35873),(#35874,#35875),(#35876,#35877),(#35878,#35879),
(#35880,#35881),(#35882,#35883),(#35884,#35885),(#35886,#35887),(#35888,
#35889),(#35890,#35891),(#35892,#35893),(#35894,#35895),(#35896,#35897),
(#35898,#35899),(#35900,#35901),(#35902,#35903),(#35904,#35905),(#35906,
#35907),(#35908,#35909),(#35910,#35911),(#35912,#35913)),.UNSPECIFIED.,
 .F.,.F.,.F.)
B_SPLINE_SURFACE_WITH_KNOTS((6,1,1,1,1,1,1,1,1,1,1,1,1,1,1,1,1,1,1,1,1,
1,1,1,1,1,1,1,1,1,1,1,1,1,1,1,1,1,1,1,1,1,1,1,1,1,1,1,1,1,1,1,1,1,1,1,1,
1,1,1,1,1,1,1,1,6),(2,2),(-1.,-0.984615384615383,-0.969230769230768,-0.953846153846152,
-0.938461538461537,-0.923076923076922,-0.907692307692306,-0.892307692307691,
-0.876923076923076,-0.86153846153846,-0.846153846153845,-0.83076923076923,
-0.815384615384614,-0.799999999999999,-0.784615384615384,-0.769230769230768,
-0.753846153846153,-0.738461538461538,-0.723076923076922,-0.707692307692307,
-0.692307692307692,-0.676923076923076,-0.661538461538461,-0.646153846153846,
-0.63076923076923,-0.615384615384615,-0.6,-0.584615384615384,-0.569230769230769,
-0.553846153846154,-0.538461538461538,-0.523076923076923,-0.507692307692308,
-0.492307692307692,-0.476923076923077,-0.461538461538462,-0.446153846153846,
-0.430769230769231,-0.415384615384615,-0.4,-0.384615384615385,-0.369230769230769,
-0.353846153846154,-0.338461538461538,-0.323076923076923,-0.307692307692308,
-0.292307692307692,-0.276923076923077,-0.261538461538462,-0.246153846153846,
-0.230769230769231,-0.215384615384615,-0.2,-0.184615384615385,-0.169230769230769,
-0.153846153846154,-0.138461538461538,-0.123076923076923,-0.107692307692308,
-0.0923076923076923,-0.0769230769230769,-0.0615384615384615,-0.0461538461538462,
-0.0307692307692308,-0.0153846153846154,0.),(-1.,1.),.UNSPECIFIED.)
GEOMETRIC_REPRESENTATION_ITEM()
RATIONAL_B_SPLINE_SURFACE(((1.,1.),(1.,1.),(1.,1.),(1.,1.),(1.,1.),(1.,
1.),(1.,1.),(1.,1.),(1.,1.),(1.,1.),(1.,1.),(1.,1.),(1.,1.),(1.,1.),(1.,
1.),(1.,1.),(1.,1.),(1.,1.),(1.,1.),(1.,1.),(1.,1.),(1.,1.),(1.,1.),(1.,
1.),(1.,1.),(1.,1.),(1.,1.),(1.,1.),(1.,1.),(1.,1.),(1.,1.),(1.,1.),(1.,
1.),(1.,1.),(1.,1.),(1.,1.),(1.,1.),(1.,1.),(1.,1.),(1.,1.),(1.,1.),(1.,
1.),(1.,1.),(1.,1.),(1.,1.),(1.,1.),(1.,1.),(1.,1.),(1.,1.),(1.,1.),(1.,
1.),(1.,1.),(1.,1.),(1.,1.),(1.,1.),(1.,1.),(1.,1.),(1.,1.),(1.,1.),(1.,
1.),(1.,1.),(1.,1.),(1.,1.),(1.,1.),(1.,1.),(1.,1.),(1.,1.),(1.,1.),(1.,
1.),(1.,1.)))
REPRESENTATION_ITEM('')
SURFACE()
);
#45=(
BOUNDED_SURFACE()
B_SPLINE_SURFACE(5,1,((#35990,#35991),(#35992,#35993),(#35994,#35995),(#35996,
#35997),(#35998,#35999),(#36000,#36001),(#36002,#36003),(#36004,#36005),
(#36006,#36007),(#36008,#36009),(#36010,#36011),(#36012,#36013),(#36014,
#36015),(#36016,#36017),(#36018,#36019),(#36020,#36021),(#36022,#36023),
(#36024,#36025),(#36026,#36027),(#36028,#36029),(#36030,#36031),(#36032,
#36033),(#36034,#36035),(#36036,#36037),(#36038,#36039),(#36040,#36041),
(#36042,#36043),(#36044,#36045),(#36046,#36047),(#36048,#36049),(#36050,
#36051),(#36052,#36053),(#36054,#36055),(#36056,#36057),(#36058,#36059),
(#36060,#36061),(#36062,#36063),(#36064,#36065),(#36066,#36067),(#36068,
#36069),(#36070,#36071),(#36072,#36073),(#36074,#36075),(#36076,#36077),
(#36078,#36079),(#36080,#36081),(#36082,#36083),(#36084,#36085),(#36086,
#36087),(#36088,#36089),(#36090,#36091),(#36092,#36093),(#36094,#36095),
(#36096,#36097),(#36098,#36099),(#36100,#36101),(#36102,#36103),(#36104,
#36105),(#36106,#36107),(#36108,#36109),(#36110,#36111),(#36112,#36113),
(#36114,#36115),(#36116,#36117),(#36118,#36119),(#36120,#36121),(#36122,
#36123),(#36124,#36125),(#36126,#36127),(#36128,#36129)),.UNSPECIFIED.,
 .F.,.F.,.F.)
B_SPLINE_SURFACE_WITH_KNOTS((6,1,1,1,1,1,1,1,1,1,1,1,1,1,1,1,1,1,1,1,1,
1,1,1,1,1,1,1,1,1,1,1,1,1,1,1,1,1,1,1,1,1,1,1,1,1,1,1,1,1,1,1,1,1,1,1,1,
1,1,1,1,1,1,1,1,6),(2,2),(-1.,-0.984615384615383,-0.969230769230768,-0.953846153846152,
-0.938461538461537,-0.923076923076922,-0.907692307692306,-0.892307692307691,
-0.876923076923076,-0.86153846153846,-0.846153846153845,-0.83076923076923,
-0.815384615384614,-0.799999999999999,-0.784615384615384,-0.769230769230768,
-0.753846153846153,-0.738461538461538,-0.723076923076922,-0.707692307692307,
-0.692307692307692,-0.676923076923076,-0.661538461538461,-0.646153846153846,
-0.63076923076923,-0.615384615384615,-0.6,-0.584615384615384,-0.569230769230769,
-0.553846153846154,-0.538461538461538,-0.523076923076923,-0.507692307692308,
-0.492307692307692,-0.476923076923077,-0.461538461538462,-0.446153846153846,
-0.430769230769231,-0.415384615384615,-0.4,-0.384615384615385,-0.369230769230769,
-0.353846153846154,-0.338461538461538,-0.323076923076923,-0.307692307692308,
-0.292307692307692,-0.276923076923077,-0.261538461538462,-0.246153846153846,
-0.230769230769231,-0.215384615384615,-0.2,-0.184615384615385,-0.169230769230769,
-0.153846153846154,-0.138461538461538,-0.123076923076923,-0.107692307692308,
-0.0923076923076923,-0.0769230769230769,-0.0615384615384615,-0.0461538461538462,
-0.0307692307692308,-0.0153846153846154,0.),(-1.,1.),.UNSPECIFIED.)
GEOMETRIC_REPRESENTATION_ITEM()
RATIONAL_B_SPLINE_SURFACE(((1.,1.),(1.,1.),(1.,1.),(1.,1.),(1.,1.),(1.,
1.),(1.,1.),(1.,1.),(1.,1.),(1.,1.),(1.,1.),(1.,1.),(1.,1.),(1.,1.),(1.,
1.),(1.,1.),(1.,1.),(1.,1.),(1.,1.),(1.,1.),(1.,1.),(1.,1.),(1.,1.),(1.,
1.),(1.,1.),(1.,1.),(1.,1.),(1.,1.),(1.,1.),(1.,1.),(1.,1.),(1.,1.),(1.,
1.),(1.,1.),(1.,1.),(1.,1.),(1.,1.),(1.,1.),(1.,1.),(1.,1.),(1.,1.),(1.,
1.),(1.,1.),(1.,1.),(1.,1.),(1.,1.),(1.,1.),(1.,1.),(1.,1.),(1.,1.),(1.,
1.),(1.,1.),(1.,1.),(1.,1.),(1.,1.),(1.,1.),(1.,1.),(1.,1.),(1.,1.),(1.,
1.),(1.,1.),(1.,1.),(1.,1.),(1.,1.),(1.,1.),(1.,1.),(1.,1.),(1.,1.),(1.,
1.),(1.,1.)))
REPRESENTATION_ITEM('')
SURFACE()
);
#46=(
BOUNDED_SURFACE()
B_SPLINE_SURFACE(5,1,((#36206,#36207),(#36208,#36209),(#36210,#36211),(#36212,
#36213),(#36214,#36215),(#36216,#36217),(#36218,#36219),(#36220,#36221),
(#36222,#36223),(#36224,#36225),(#36226,#36227),(#36228,#36229),(#36230,
#36231),(#36232,#36233),(#36234,#36235),(#36236,#36237),(#36238,#36239),
(#36240,#36241),(#36242,#36243),(#36244,#36245),(#36246,#36247),(#36248,
#36249),(#36250,#36251),(#36252,#36253),(#36254,#36255),(#36256,#36257),
(#36258,#36259),(#36260,#36261),(#36262,#36263),(#36264,#36265),(#36266,
#36267),(#36268,#36269),(#36270,#36271),(#36272,#36273),(#36274,#36275),
(#36276,#36277),(#36278,#36279),(#36280,#36281),(#36282,#36283),(#36284,
#36285),(#36286,#36287),(#36288,#36289),(#36290,#36291),(#36292,#36293),
(#36294,#36295),(#36296,#36297),(#36298,#36299),(#36300,#36301),(#36302,
#36303),(#36304,#36305),(#36306,#36307),(#36308,#36309),(#36310,#36311),
(#36312,#36313),(#36314,#36315),(#36316,#36317),(#36318,#36319),(#36320,
#36321),(#36322,#36323),(#36324,#36325),(#36326,#36327),(#36328,#36329),
(#36330,#36331),(#36332,#36333),(#36334,#36335),(#36336,#36337),(#36338,
#36339),(#36340,#36341),(#36342,#36343),(#36344,#36345)),.UNSPECIFIED.,
 .F.,.F.,.F.)
B_SPLINE_SURFACE_WITH_KNOTS((6,1,1,1,1,1,1,1,1,1,1,1,1,1,1,1,1,1,1,1,1,
1,1,1,1,1,1,1,1,1,1,1,1,1,1,1,1,1,1,1,1,1,1,1,1,1,1,1,1,1,1,1,1,1,1,1,1,
1,1,1,1,1,1,1,1,6),(2,2),(-1.,-0.984615384615383,-0.969230769230768,-0.953846153846152,
-0.938461538461537,-0.923076923076922,-0.907692307692306,-0.892307692307691,
-0.876923076923076,-0.86153846153846,-0.846153846153845,-0.83076923076923,
-0.815384615384614,-0.799999999999999,-0.784615384615384,-0.769230769230768,
-0.753846153846153,-0.738461538461538,-0.723076923076922,-0.707692307692307,
-0.692307692307692,-0.676923076923076,-0.661538461538461,-0.646153846153846,
-0.63076923076923,-0.615384615384615,-0.6,-0.584615384615384,-0.569230769230769,
-0.553846153846154,-0.538461538461538,-0.523076923076923,-0.507692307692308,
-0.492307692307692,-0.476923076923077,-0.461538461538462,-0.446153846153846,
-0.430769230769231,-0.415384615384615,-0.4,-0.384615384615385,-0.369230769230769,
-0.353846153846154,-0.338461538461538,-0.323076923076923,-0.307692307692308,
-0.292307692307692,-0.276923076923077,-0.261538461538462,-0.246153846153846,
-0.230769230769231,-0.215384615384615,-0.2,-0.184615384615385,-0.169230769230769,
-0.153846153846154,-0.138461538461538,-0.123076923076923,-0.107692307692308,
-0.0923076923076923,-0.0769230769230769,-0.0615384615384615,-0.0461538461538462,
-0.0307692307692308,-0.0153846153846154,0.),(-1.,1.),.UNSPECIFIED.)
GEOMETRIC_REPRESENTATION_ITEM()
RATIONAL_B_SPLINE_SURFACE(((1.,1.),(1.,1.),(1.,1.),(1.,1.),(1.,1.),(1.,
1.),(1.,1.),(1.,1.),(1.,1.),(1.,1.),(1.,1.),(1.,1.),(1.,1.),(1.,1.),(1.,
1.),(1.,1.),(1.,1.),(1.,1.),(1.,1.),(1.,1.),(1.,1.),(1.,1.),(1.,1.),(1.,
1.),(1.,1.),(1.,1.),(1.,1.),(1.,1.),(1.,1.),(1.,1.),(1.,1.),(1.,1.),(1.,
1.),(1.,1.),(1.,1.),(1.,1.),(1.,1.),(1.,1.),(1.,1.),(1.,1.),(1.,1.),(1.,
1.),(1.,1.),(1.,1.),(1.,1.),(1.,1.),(1.,1.),(1.,1.),(1.,1.),(1.,1.),(1.,
1.),(1.,1.),(1.,1.),(1.,1.),(1.,1.),(1.,1.),(1.,1.),(1.,1.),(1.,1.),(1.,
1.),(1.,1.),(1.,1.),(1.,1.),(1.,1.),(1.,1.),(1.,1.),(1.,1.),(1.,1.),(1.,
1.),(1.,1.)))
REPRESENTATION_ITEM('')
SURFACE()
);
#47=(
BOUNDED_SURFACE()
B_SPLINE_SURFACE(5,1,((#36422,#36423),(#36424,#36425),(#36426,#36427),(#36428,
#36429),(#36430,#36431),(#36432,#36433),(#36434,#36435),(#36436,#36437),
(#36438,#36439),(#36440,#36441),(#36442,#36443),(#36444,#36445),(#36446,
#36447),(#36448,#36449),(#36450,#36451),(#36452,#36453),(#36454,#36455),
(#36456,#36457),(#36458,#36459),(#36460,#36461),(#36462,#36463),(#36464,
#36465),(#36466,#36467),(#36468,#36469),(#36470,#36471),(#36472,#36473),
(#36474,#36475),(#36476,#36477),(#36478,#36479),(#36480,#36481),(#36482,
#36483),(#36484,#36485),(#36486,#36487),(#36488,#36489),(#36490,#36491),
(#36492,#36493),(#36494,#36495),(#36496,#36497),(#36498,#36499),(#36500,
#36501),(#36502,#36503),(#36504,#36505),(#36506,#36507),(#36508,#36509),
(#36510,#36511),(#36512,#36513),(#36514,#36515),(#36516,#36517),(#36518,
#36519),(#36520,#36521),(#36522,#36523),(#36524,#36525),(#36526,#36527),
(#36528,#36529),(#36530,#36531),(#36532,#36533),(#36534,#36535),(#36536,
#36537),(#36538,#36539),(#36540,#36541),(#36542,#36543),(#36544,#36545),
(#36546,#36547),(#36548,#36549),(#36550,#36551),(#36552,#36553),(#36554,
#36555),(#36556,#36557),(#36558,#36559),(#36560,#36561)),.UNSPECIFIED.,
 .F.,.F.,.F.)
B_SPLINE_SURFACE_WITH_KNOTS((6,1,1,1,1,1,1,1,1,1,1,1,1,1,1,1,1,1,1,1,1,
1,1,1,1,1,1,1,1,1,1,1,1,1,1,1,1,1,1,1,1,1,1,1,1,1,1,1,1,1,1,1,1,1,1,1,1,
1,1,1,1,1,1,1,1,6),(2,2),(-1.,-0.984615384615383,-0.969230769230768,-0.953846153846152,
-0.938461538461537,-0.923076923076922,-0.907692307692306,-0.892307692307691,
-0.876923076923076,-0.86153846153846,-0.846153846153845,-0.83076923076923,
-0.815384615384614,-0.799999999999999,-0.784615384615384,-0.769230769230768,
-0.753846153846153,-0.738461538461538,-0.723076923076922,-0.707692307692307,
-0.692307692307692,-0.676923076923076,-0.661538461538461,-0.646153846153846,
-0.63076923076923,-0.615384615384615,-0.6,-0.584615384615384,-0.569230769230769,
-0.553846153846154,-0.538461538461538,-0.523076923076923,-0.507692307692308,
-0.492307692307692,-0.476923076923077,-0.461538461538462,-0.446153846153846,
-0.430769230769231,-0.415384615384615,-0.4,-0.384615384615385,-0.369230769230769,
-0.353846153846154,-0.338461538461538,-0.323076923076923,-0.307692307692308,
-0.292307692307692,-0.276923076923077,-0.261538461538462,-0.246153846153846,
-0.230769230769231,-0.215384615384615,-0.2,-0.184615384615385,-0.169230769230769,
-0.153846153846154,-0.138461538461538,-0.123076923076923,-0.107692307692308,
-0.0923076923076923,-0.0769230769230769,-0.0615384615384615,-0.0461538461538462,
-0.0307692307692308,-0.0153846153846154,0.),(-1.,1.),.UNSPECIFIED.)
GEOMETRIC_REPRESENTATION_ITEM()
RATIONAL_B_SPLINE_SURFACE(((1.,1.),(1.,1.),(1.,1.),(1.,1.),(1.,1.),(1.,
1.),(1.,1.),(1.,1.),(1.,1.),(1.,1.),(1.,1.),(1.,1.),(1.,1.),(1.,1.),(1.,
1.),(1.,1.),(1.,1.),(1.,1.),(1.,1.),(1.,1.),(1.,1.),(1.,1.),(1.,1.),(1.,
1.),(1.,1.),(1.,1.),(1.,1.),(1.,1.),(1.,1.),(1.,1.),(1.,1.),(1.,1.),(1.,
1.),(1.,1.),(1.,1.),(1.,1.),(1.,1.),(1.,1.),(1.,1.),(1.,1.),(1.,1.),(1.,
1.),(1.,1.),(1.,1.),(1.,1.),(1.,1.),(1.,1.),(1.,1.),(1.,1.),(1.,1.),(1.,
1.),(1.,1.),(1.,1.),(1.,1.),(1.,1.),(1.,1.),(1.,1.),(1.,1.),(1.,1.),(1.,
1.),(1.,1.),(1.,1.),(1.,1.),(1.,1.),(1.,1.),(1.,1.),(1.,1.),(1.,1.),(1.,
1.),(1.,1.)))
REPRESENTATION_ITEM('')
SURFACE()
);
#48=(
BOUNDED_SURFACE()
B_SPLINE_SURFACE(5,1,((#36638,#36639),(#36640,#36641),(#36642,#36643),(#36644,
#36645),(#36646,#36647),(#36648,#36649),(#36650,#36651),(#36652,#36653),
(#36654,#36655),(#36656,#36657),(#36658,#36659),(#36660,#36661),(#36662,
#36663),(#36664,#36665),(#36666,#36667),(#36668,#36669),(#36670,#36671),
(#36672,#36673),(#36674,#36675),(#36676,#36677),(#36678,#36679),(#36680,
#36681),(#36682,#36683),(#36684,#36685),(#36686,#36687),(#36688,#36689),
(#36690,#36691),(#36692,#36693),(#36694,#36695),(#36696,#36697),(#36698,
#36699),(#36700,#36701),(#36702,#36703),(#36704,#36705),(#36706,#36707),
(#36708,#36709),(#36710,#36711),(#36712,#36713),(#36714,#36715),(#36716,
#36717),(#36718,#36719),(#36720,#36721),(#36722,#36723),(#36724,#36725),
(#36726,#36727),(#36728,#36729),(#36730,#36731),(#36732,#36733),(#36734,
#36735),(#36736,#36737),(#36738,#36739),(#36740,#36741),(#36742,#36743),
(#36744,#36745),(#36746,#36747),(#36748,#36749),(#36750,#36751),(#36752,
#36753),(#36754,#36755),(#36756,#36757),(#36758,#36759),(#36760,#36761),
(#36762,#36763),(#36764,#36765),(#36766,#36767),(#36768,#36769),(#36770,
#36771),(#36772,#36773),(#36774,#36775),(#36776,#36777)),.UNSPECIFIED.,
 .F.,.F.,.F.)
B_SPLINE_SURFACE_WITH_KNOTS((6,1,1,1,1,1,1,1,1,1,1,1,1,1,1,1,1,1,1,1,1,
1,1,1,1,1,1,1,1,1,1,1,1,1,1,1,1,1,1,1,1,1,1,1,1,1,1,1,1,1,1,1,1,1,1,1,1,
1,1,1,1,1,1,1,1,6),(2,2),(-1.,-0.984615384615383,-0.969230769230768,-0.953846153846152,
-0.938461538461537,-0.923076923076922,-0.907692307692306,-0.892307692307691,
-0.876923076923076,-0.86153846153846,-0.846153846153845,-0.83076923076923,
-0.815384615384614,-0.799999999999999,-0.784615384615384,-0.769230769230768,
-0.753846153846153,-0.738461538461538,-0.723076923076922,-0.707692307692307,
-0.692307692307692,-0.676923076923076,-0.661538461538461,-0.646153846153846,
-0.63076923076923,-0.615384615384615,-0.6,-0.584615384615384,-0.569230769230769,
-0.553846153846154,-0.538461538461538,-0.523076923076923,-0.507692307692308,
-0.492307692307692,-0.476923076923077,-0.461538461538462,-0.446153846153846,
-0.430769230769231,-0.415384615384615,-0.4,-0.384615384615385,-0.369230769230769,
-0.353846153846154,-0.338461538461538,-0.323076923076923,-0.307692307692308,
-0.292307692307692,-0.276923076923077,-0.261538461538462,-0.246153846153846,
-0.230769230769231,-0.215384615384615,-0.2,-0.184615384615385,-0.169230769230769,
-0.153846153846154,-0.138461538461538,-0.123076923076923,-0.107692307692308,
-0.0923076923076923,-0.0769230769230769,-0.0615384615384615,-0.0461538461538462,
-0.0307692307692308,-0.0153846153846154,0.),(-1.,1.),.UNSPECIFIED.)
GEOMETRIC_REPRESENTATION_ITEM()
RATIONAL_B_SPLINE_SURFACE(((1.,1.),(1.,1.),(1.,1.),(1.,1.),(1.,1.),(1.,
1.),(1.,1.),(1.,1.),(1.,1.),(1.,1.),(1.,1.),(1.,1.),(1.,1.),(1.,1.),(1.,
1.),(1.,1.),(1.,1.),(1.,1.),(1.,1.),(1.,1.),(1.,1.),(1.,1.),(1.,1.),(1.,
1.),(1.,1.),(1.,1.),(1.,1.),(1.,1.),(1.,1.),(1.,1.),(1.,1.),(1.,1.),(1.,
1.),(1.,1.),(1.,1.),(1.,1.),(1.,1.),(1.,1.),(1.,1.),(1.,1.),(1.,1.),(1.,
1.),(1.,1.),(1.,1.),(1.,1.),(1.,1.),(1.,1.),(1.,1.),(1.,1.),(1.,1.),(1.,
1.),(1.,1.),(1.,1.),(1.,1.),(1.,1.),(1.,1.),(1.,1.),(1.,1.),(1.,1.),(1.,
1.),(1.,1.),(1.,1.),(1.,1.),(1.,1.),(1.,1.),(1.,1.),(1.,1.),(1.,1.),(1.,
1.),(1.,1.)))
REPRESENTATION_ITEM('')
SURFACE()
);
#49=(
BOUNDED_SURFACE()
B_SPLINE_SURFACE(5,1,((#36854,#36855),(#36856,#36857),(#36858,#36859),(#36860,
#36861),(#36862,#36863),(#36864,#36865),(#36866,#36867),(#36868,#36869),
(#36870,#36871),(#36872,#36873),(#36874,#36875),(#36876,#36877),(#36878,
#36879),(#36880,#36881),(#36882,#36883),(#36884,#36885),(#36886,#36887),
(#36888,#36889),(#36890,#36891),(#36892,#36893),(#36894,#36895),(#36896,
#36897),(#36898,#36899),(#36900,#36901),(#36902,#36903),(#36904,#36905),
(#36906,#36907),(#36908,#36909),(#36910,#36911),(#36912,#36913),(#36914,
#36915),(#36916,#36917),(#36918,#36919),(#36920,#36921),(#36922,#36923),
(#36924,#36925),(#36926,#36927),(#36928,#36929),(#36930,#36931),(#36932,
#36933),(#36934,#36935),(#36936,#36937),(#36938,#36939),(#36940,#36941),
(#36942,#36943),(#36944,#36945),(#36946,#36947),(#36948,#36949),(#36950,
#36951),(#36952,#36953),(#36954,#36955),(#36956,#36957),(#36958,#36959),
(#36960,#36961),(#36962,#36963),(#36964,#36965),(#36966,#36967),(#36968,
#36969),(#36970,#36971),(#36972,#36973),(#36974,#36975),(#36976,#36977),
(#36978,#36979),(#36980,#36981),(#36982,#36983),(#36984,#36985),(#36986,
#36987),(#36988,#36989),(#36990,#36991),(#36992,#36993)),.UNSPECIFIED.,
 .F.,.F.,.F.)
B_SPLINE_SURFACE_WITH_KNOTS((6,1,1,1,1,1,1,1,1,1,1,1,1,1,1,1,1,1,1,1,1,
1,1,1,1,1,1,1,1,1,1,1,1,1,1,1,1,1,1,1,1,1,1,1,1,1,1,1,1,1,1,1,1,1,1,1,1,
1,1,1,1,1,1,1,1,6),(2,2),(-1.,-0.984615384615383,-0.969230769230768,-0.953846153846152,
-0.938461538461537,-0.923076923076922,-0.907692307692306,-0.892307692307691,
-0.876923076923076,-0.86153846153846,-0.846153846153845,-0.83076923076923,
-0.815384615384614,-0.799999999999999,-0.784615384615384,-0.769230769230768,
-0.753846153846153,-0.738461538461538,-0.723076923076922,-0.707692307692307,
-0.692307692307692,-0.676923076923076,-0.661538461538461,-0.646153846153846,
-0.63076923076923,-0.615384615384615,-0.6,-0.584615384615384,-0.569230769230769,
-0.553846153846154,-0.538461538461538,-0.523076923076923,-0.507692307692308,
-0.492307692307692,-0.476923076923077,-0.461538461538462,-0.446153846153846,
-0.430769230769231,-0.415384615384615,-0.4,-0.384615384615385,-0.369230769230769,
-0.353846153846154,-0.338461538461538,-0.323076923076923,-0.307692307692308,
-0.292307692307692,-0.276923076923077,-0.261538461538462,-0.246153846153846,
-0.230769230769231,-0.215384615384615,-0.2,-0.184615384615385,-0.169230769230769,
-0.153846153846154,-0.138461538461538,-0.123076923076923,-0.107692307692308,
-0.0923076923076923,-0.0769230769230769,-0.0615384615384615,-0.0461538461538462,
-0.0307692307692308,-0.0153846153846154,0.),(-1.,1.),.UNSPECIFIED.)
GEOMETRIC_REPRESENTATION_ITEM()
RATIONAL_B_SPLINE_SURFACE(((1.,1.),(1.,1.),(1.,1.),(1.,1.),(1.,1.),(1.,
1.),(1.,1.),(1.,1.),(1.,1.),(1.,1.),(1.,1.),(1.,1.),(1.,1.),(1.,1.),(1.,
1.),(1.,1.),(1.,1.),(1.,1.),(1.,1.),(1.,1.),(1.,1.),(1.,1.),(1.,1.),(1.,
1.),(1.,1.),(1.,1.),(1.,1.),(1.,1.),(1.,1.),(1.,1.),(1.,1.),(1.,1.),(1.,
1.),(1.,1.),(1.,1.),(1.,1.),(1.,1.),(1.,1.),(1.,1.),(1.,1.),(1.,1.),(1.,
1.),(1.,1.),(1.,1.),(1.,1.),(1.,1.),(1.,1.),(1.,1.),(1.,1.),(1.,1.),(1.,
1.),(1.,1.),(1.,1.),(1.,1.),(1.,1.),(1.,1.),(1.,1.),(1.,1.),(1.,1.),(1.,
1.),(1.,1.),(1.,1.),(1.,1.),(1.,1.),(1.,1.),(1.,1.),(1.,1.),(1.,1.),(1.,
1.),(1.,1.)))
REPRESENTATION_ITEM('')
SURFACE()
);
#50=(
BOUNDED_SURFACE()
B_SPLINE_SURFACE(5,1,((#37070,#37071),(#37072,#37073),(#37074,#37075),(#37076,
#37077),(#37078,#37079),(#37080,#37081),(#37082,#37083),(#37084,#37085),
(#37086,#37087),(#37088,#37089),(#37090,#37091),(#37092,#37093),(#37094,
#37095),(#37096,#37097),(#37098,#37099),(#37100,#37101),(#37102,#37103),
(#37104,#37105),(#37106,#37107),(#37108,#37109),(#37110,#37111),(#37112,
#37113),(#37114,#37115),(#37116,#37117),(#37118,#37119),(#37120,#37121),
(#37122,#37123),(#37124,#37125),(#37126,#37127),(#37128,#37129),(#37130,
#37131),(#37132,#37133),(#37134,#37135),(#37136,#37137),(#37138,#37139),
(#37140,#37141),(#37142,#37143),(#37144,#37145),(#37146,#37147),(#37148,
#37149),(#37150,#37151),(#37152,#37153),(#37154,#37155),(#37156,#37157),
(#37158,#37159),(#37160,#37161),(#37162,#37163),(#37164,#37165),(#37166,
#37167),(#37168,#37169),(#37170,#37171),(#37172,#37173),(#37174,#37175),
(#37176,#37177),(#37178,#37179),(#37180,#37181),(#37182,#37183),(#37184,
#37185),(#37186,#37187),(#37188,#37189),(#37190,#37191),(#37192,#37193),
(#37194,#37195),(#37196,#37197),(#37198,#37199),(#37200,#37201),(#37202,
#37203),(#37204,#37205),(#37206,#37207),(#37208,#37209)),.UNSPECIFIED.,
 .F.,.F.,.F.)
B_SPLINE_SURFACE_WITH_KNOTS((6,1,1,1,1,1,1,1,1,1,1,1,1,1,1,1,1,1,1,1,1,
1,1,1,1,1,1,1,1,1,1,1,1,1,1,1,1,1,1,1,1,1,1,1,1,1,1,1,1,1,1,1,1,1,1,1,1,
1,1,1,1,1,1,1,1,6),(2,2),(-1.,-0.984615384615383,-0.969230769230768,-0.953846153846152,
-0.938461538461537,-0.923076923076922,-0.907692307692306,-0.892307692307691,
-0.876923076923076,-0.86153846153846,-0.846153846153845,-0.83076923076923,
-0.815384615384614,-0.799999999999999,-0.784615384615384,-0.769230769230768,
-0.753846153846153,-0.738461538461538,-0.723076923076922,-0.707692307692307,
-0.692307692307692,-0.676923076923076,-0.661538461538461,-0.646153846153846,
-0.63076923076923,-0.615384615384615,-0.6,-0.584615384615384,-0.569230769230769,
-0.553846153846154,-0.538461538461538,-0.523076923076923,-0.507692307692308,
-0.492307692307692,-0.476923076923077,-0.461538461538462,-0.446153846153846,
-0.430769230769231,-0.415384615384615,-0.4,-0.384615384615385,-0.369230769230769,
-0.353846153846154,-0.338461538461538,-0.323076923076923,-0.307692307692308,
-0.292307692307692,-0.276923076923077,-0.261538461538462,-0.246153846153846,
-0.230769230769231,-0.215384615384615,-0.2,-0.184615384615385,-0.169230769230769,
-0.153846153846154,-0.138461538461538,-0.123076923076923,-0.107692307692308,
-0.0923076923076923,-0.0769230769230769,-0.0615384615384615,-0.0461538461538462,
-0.0307692307692308,-0.0153846153846154,0.),(-1.,1.),.UNSPECIFIED.)
GEOMETRIC_REPRESENTATION_ITEM()
RATIONAL_B_SPLINE_SURFACE(((1.,1.),(1.,1.),(1.,1.),(1.,1.),(1.,1.),(1.,
1.),(1.,1.),(1.,1.),(1.,1.),(1.,1.),(1.,1.),(1.,1.),(1.,1.),(1.,1.),(1.,
1.),(1.,1.),(1.,1.),(1.,1.),(1.,1.),(1.,1.),(1.,1.),(1.,1.),(1.,1.),(1.,
1.),(1.,1.),(1.,1.),(1.,1.),(1.,1.),(1.,1.),(1.,1.),(1.,1.),(1.,1.),(1.,
1.),(1.,1.),(1.,1.),(1.,1.),(1.,1.),(1.,1.),(1.,1.),(1.,1.),(1.,1.),(1.,
1.),(1.,1.),(1.,1.),(1.,1.),(1.,1.),(1.,1.),(1.,1.),(1.,1.),(1.,1.),(1.,
1.),(1.,1.),(1.,1.),(1.,1.),(1.,1.),(1.,1.),(1.,1.),(1.,1.),(1.,1.),(1.,
1.),(1.,1.),(1.,1.),(1.,1.),(1.,1.),(1.,1.),(1.,1.),(1.,1.),(1.,1.),(1.,
1.),(1.,1.)))
REPRESENTATION_ITEM('')
SURFACE()
);
#171=(
BOUNDED_CURVE()
B_SPLINE_CURVE(5,(#25718,#25719,#25720,#25721,#25722,#25723,#25724,#25725,
#25726,#25727,#25728,#25729,#25730,#25731,#25732,#25733,#25734,#25735,#25736,
#25737,#25738,#25739,#25740,#25741,#25742,#25743,#25744,#25745,#25746,#25747,
#25748,#25749,#25750,#25751,#25752,#25753,#25754,#25755,#25756,#25757,#25758,
#25759,#25760,#25761,#25762,#25763,#25764,#25765,#25766,#25767,#25768,#25769,
#25770,#25771,#25772,#25773,#25774,#25775,#25776,#25777,#25778,#25779,#25780,
#25781,#25782,#25783,#25784,#25785,#25786,#25787),.UNSPECIFIED.,.F.,.F.)
B_SPLINE_CURVE_WITH_KNOTS((6,1,1,1,1,1,1,1,1,1,1,1,1,1,1,1,1,1,1,1,1,1,
1,1,1,1,1,1,1,1,1,1,1,1,1,1,1,1,1,1,1,1,1,1,1,1,1,1,1,1,1,1,1,1,1,1,1,1,
1,1,1,1,1,1,1,6),(0.,0.0153846153846154,0.0307692307692308,0.0461538461538462,
0.0615384615384615,0.0769230769230769,0.0923076923076923,0.107692307692308,
0.123076923076923,0.138461538461538,0.153846153846154,0.169230769230769,
0.184615384615385,0.2,0.215384615384615,0.230769230769231,0.246153846153846,
0.261538461538462,0.276923076923077,0.292307692307692,0.307692307692308,
0.323076923076923,0.338461538461538,0.353846153846154,0.369230769230769,
0.384615384615385,0.4,0.415384615384615,0.430769230769231,0.446153846153846,
0.461538461538462,0.476923076923077,0.492307692307692,0.507692307692308,
0.523076923076923,0.538461538461538,0.553846153846154,0.569230769230769,
0.584615384615384,0.6,0.615384615384615,0.63076923076923,0.646153846153846,
0.661538461538461,0.676923076923076,0.692307692307692,0.707692307692307,
0.723076923076922,0.738461538461538,0.753846153846153,0.769230769230768,
0.784615384615384,0.799999999999999,0.815384615384614,0.83076923076923,
0.846153846153845,0.86153846153846,0.876923076923076,0.892307692307691,
0.907692307692306,0.923076923076922,0.938461538461537,0.953846153846152,
0.969230769230768,0.984615384615383,1.),.UNSPECIFIED.)
CURVE()
GEOMETRIC_REPRESENTATION_ITEM()
RATIONAL_B_SPLINE_CURVE((1.,1.,1.,1.,1.,1.,1.,1.,1.,1.,1.,1.,1.,1.,1.,1.,
1.,1.,1.,1.,1.,1.,1.,1.,1.,1.,1.,1.,1.,1.,1.,1.,1.,1.,1.,1.,1.,1.,1.,1.,
1.,1.,1.,1.,1.,1.,1.,1.,1.,1.,1.,1.,1.,1.,1.,1.,1.,1.,1.,1.,1.,1.,1.,1.,
1.,1.,1.,1.,1.,1.))
REPRESENTATION_ITEM('')
);
#172=(
BOUNDED_CURVE()
B_SPLINE_CURVE(5,(#25791,#25792,#25793,#25794,#25795,#25796,#25797,#25798,
#25799,#25800,#25801,#25802,#25803,#25804,#25805,#25806,#25807,#25808,#25809,
#25810,#25811,#25812,#25813,#25814,#25815,#25816,#25817,#25818,#25819,#25820,
#25821,#25822,#25823,#25824,#25825,#25826,#25827,#25828,#25829,#25830,#25831,
#25832,#25833,#25834,#25835,#25836,#25837,#25838,#25839,#25840,#25841,#25842,
#25843,#25844,#25845,#25846,#25847,#25848,#25849,#25850,#25851,#25852,#25853,
#25854,#25855,#25856,#25857,#25858,#25859,#25860),.UNSPECIFIED.,.F.,.F.)
B_SPLINE_CURVE_WITH_KNOTS((6,1,1,1,1,1,1,1,1,1,1,1,1,1,1,1,1,1,1,1,1,1,
1,1,1,1,1,1,1,1,1,1,1,1,1,1,1,1,1,1,1,1,1,1,1,1,1,1,1,1,1,1,1,1,1,1,1,1,
1,1,1,1,1,1,1,6),(0.,0.0153846153846154,0.0307692307692308,0.0461538461538462,
0.0615384615384615,0.0769230769230769,0.0923076923076923,0.107692307692308,
0.123076923076923,0.138461538461538,0.153846153846154,0.169230769230769,
0.184615384615385,0.2,0.215384615384615,0.230769230769231,0.246153846153846,
0.261538461538462,0.276923076923077,0.292307692307692,0.307692307692308,
0.323076923076923,0.338461538461538,0.353846153846154,0.369230769230769,
0.384615384615385,0.4,0.415384615384615,0.430769230769231,0.446153846153846,
0.461538461538462,0.476923076923077,0.492307692307692,0.507692307692308,
0.523076923076923,0.538461538461538,0.553846153846154,0.569230769230769,
0.584615384615384,0.6,0.615384615384615,0.63076923076923,0.646153846153846,
0.661538461538461,0.676923076923076,0.692307692307692,0.707692307692307,
0.723076923076922,0.738461538461538,0.753846153846153,0.769230769230768,
0.784615384615384,0.799999999999999,0.815384615384614,0.83076923076923,
0.846153846153845,0.86153846153846,0.876923076923076,0.892307692307691,
0.907692307692306,0.923076923076922,0.938461538461537,0.953846153846152,
0.969230769230768,0.984615384615383,1.),.UNSPECIFIED.)
CURVE()
GEOMETRIC_REPRESENTATION_ITEM()
RATIONAL_B_SPLINE_CURVE((1.,1.,1.,1.,1.,1.,1.,1.,1.,1.,1.,1.,1.,1.,1.,1.,
1.,1.,1.,1.,1.,1.,1.,1.,1.,1.,1.,1.,1.,1.,1.,1.,1.,1.,1.,1.,1.,1.,1.,1.,
1.,1.,1.,1.,1.,1.,1.,1.,1.,1.,1.,1.,1.,1.,1.,1.,1.,1.,1.,1.,1.,1.,1.,1.,
1.,1.,1.,1.,1.,1.))
REPRESENTATION_ITEM('')
);
#173=(
BOUNDED_CURVE()
B_SPLINE_CURVE(5,(#25864,#25865,#25866,#25867,#25868,#25869,#25870,#25871,
#25872,#25873,#25874,#25875,#25876,#25877,#25878,#25879,#25880,#25881,#25882,
#25883,#25884,#25885,#25886,#25887,#25888,#25889,#25890,#25891,#25892,#25893,
#25894,#25895,#25896,#25897,#25898,#25899,#25900,#25901,#25902,#25903,#25904,
#25905,#25906,#25907,#25908,#25909,#25910,#25911,#25912,#25913,#25914,#25915,
#25916,#25917,#25918,#25919,#25920,#25921,#25922,#25923,#25924,#25925,#25926,
#25927,#25928,#25929,#25930,#25931,#25932,#25933),.UNSPECIFIED.,.F.,.F.)
B_SPLINE_CURVE_WITH_KNOTS((6,1,1,1,1,1,1,1,1,1,1,1,1,1,1,1,1,1,1,1,1,1,
1,1,1,1,1,1,1,1,1,1,1,1,1,1,1,1,1,1,1,1,1,1,1,1,1,1,1,1,1,1,1,1,1,1,1,1,
1,1,1,1,1,1,1,6),(0.,0.0153846153846154,0.0307692307692308,0.0461538461538462,
0.0615384615384615,0.0769230769230769,0.0923076923076923,0.107692307692308,
0.123076923076923,0.138461538461538,0.153846153846154,0.169230769230769,
0.184615384615385,0.2,0.215384615384615,0.230769230769231,0.246153846153846,
0.261538461538462,0.276923076923077,0.292307692307692,0.307692307692308,
0.323076923076923,0.338461538461538,0.353846153846154,0.369230769230769,
0.384615384615385,0.4,0.415384615384615,0.430769230769231,0.446153846153846,
0.461538461538462,0.476923076923077,0.492307692307692,0.507692307692308,
0.523076923076923,0.538461538461538,0.553846153846154,0.569230769230769,
0.584615384615384,0.6,0.615384615384615,0.63076923076923,0.646153846153846,
0.661538461538461,0.676923076923076,0.692307692307692,0.707692307692307,
0.723076923076922,0.738461538461538,0.753846153846153,0.769230769230768,
0.784615384615384,0.799999999999999,0.815384615384614,0.83076923076923,
0.846153846153845,0.86153846153846,0.876923076923076,0.892307692307691,
0.907692307692306,0.923076923076922,0.938461538461537,0.953846153846152,
0.969230769230768,0.984615384615383,1.),.UNSPECIFIED.)
CURVE()
GEOMETRIC_REPRESENTATION_ITEM()
RATIONAL_B_SPLINE_CURVE((1.,1.,1.,1.,1.,1.,1.,1.,1.,1.,1.,1.,1.,1.,1.,1.,
1.,1.,1.,1.,1.,1.,1.,1.,1.,1.,1.,1.,1.,1.,1.,1.,1.,1.,1.,1.,1.,1.,1.,1.,
1.,1.,1.,1.,1.,1.,1.,1.,1.,1.,1.,1.,1.,1.,1.,1.,1.,1.,1.,1.,1.,1.,1.,1.,
1.,1.,1.,1.,1.,1.))
REPRESENTATION_ITEM('')
);
#174=(
BOUNDED_CURVE()
B_SPLINE_CURVE(5,(#25937,#25938,#25939,#25940,#25941,#25942,#25943,#25944,
#25945,#25946,#25947,#25948,#25949,#25950,#25951,#25952,#25953,#25954,#25955,
#25956,#25957,#25958,#25959,#25960,#25961,#25962,#25963,#25964,#25965,#25966,
#25967,#25968,#25969,#25970,#25971,#25972,#25973,#25974,#25975,#25976,#25977,
#25978,#25979,#25980,#25981,#25982,#25983,#25984,#25985,#25986,#25987,#25988,
#25989,#25990,#25991,#25992,#25993,#25994,#25995,#25996,#25997,#25998,#25999,
#26000,#26001,#26002,#26003,#26004,#26005,#26006),.UNSPECIFIED.,.F.,.F.)
B_SPLINE_CURVE_WITH_KNOTS((6,1,1,1,1,1,1,1,1,1,1,1,1,1,1,1,1,1,1,1,1,1,
1,1,1,1,1,1,1,1,1,1,1,1,1,1,1,1,1,1,1,1,1,1,1,1,1,1,1,1,1,1,1,1,1,1,1,1,
1,1,1,1,1,1,1,6),(0.,0.0153846153846154,0.0307692307692308,0.0461538461538462,
0.0615384615384615,0.0769230769230769,0.0923076923076923,0.107692307692308,
0.123076923076923,0.138461538461538,0.153846153846154,0.169230769230769,
0.184615384615385,0.2,0.215384615384615,0.230769230769231,0.246153846153846,
0.261538461538462,0.276923076923077,0.292307692307692,0.307692307692308,
0.323076923076923,0.338461538461538,0.353846153846154,0.369230769230769,
0.384615384615385,0.4,0.415384615384615,0.430769230769231,0.446153846153846,
0.461538461538462,0.476923076923077,0.492307692307692,0.507692307692308,
0.523076923076923,0.538461538461538,0.553846153846154,0.569230769230769,
0.584615384615384,0.6,0.615384615384615,0.63076923076923,0.646153846153846,
0.661538461538461,0.676923076923076,0.692307692307692,0.707692307692307,
0.723076923076922,0.738461538461538,0.753846153846153,0.769230769230768,
0.784615384615384,0.799999999999999,0.815384615384614,0.83076923076923,
0.846153846153845,0.86153846153846,0.876923076923076,0.892307692307691,
0.907692307692306,0.923076923076922,0.938461538461537,0.953846153846152,
0.969230769230768,0.984615384615383,1.),.UNSPECIFIED.)
CURVE()
GEOMETRIC_REPRESENTATION_ITEM()
RATIONAL_B_SPLINE_CURVE((1.,1.,1.,1.,1.,1.,1.,1.,1.,1.,1.,1.,1.,1.,1.,1.,
1.,1.,1.,1.,1.,1.,1.,1.,1.,1.,1.,1.,1.,1.,1.,1.,1.,1.,1.,1.,1.,1.,1.,1.,
1.,1.,1.,1.,1.,1.,1.,1.,1.,1.,1.,1.,1.,1.,1.,1.,1.,1.,1.,1.,1.,1.,1.,1.,
1.,1.,1.,1.,1.,1.))
REPRESENTATION_ITEM('')
);
#175=(
BOUNDED_CURVE()
B_SPLINE_CURVE(5,(#26010,#26011,#26012,#26013,#26014,#26015,#26016,#26017,
#26018,#26019,#26020,#26021,#26022,#26023,#26024,#26025,#26026,#26027,#26028,
#26029,#26030,#26031,#26032,#26033,#26034,#26035,#26036,#26037,#26038,#26039,
#26040,#26041,#26042,#26043,#26044,#26045,#26046,#26047,#26048,#26049,#26050,
#26051,#26052,#26053,#26054,#26055,#26056,#26057,#26058,#26059,#26060,#26061,
#26062,#26063,#26064,#26065,#26066,#26067,#26068,#26069,#26070,#26071,#26072,
#26073,#26074,#26075,#26076,#26077,#26078,#26079),.UNSPECIFIED.,.F.,.F.)
B_SPLINE_CURVE_WITH_KNOTS((6,1,1,1,1,1,1,1,1,1,1,1,1,1,1,1,1,1,1,1,1,1,
1,1,1,1,1,1,1,1,1,1,1,1,1,1,1,1,1,1,1,1,1,1,1,1,1,1,1,1,1,1,1,1,1,1,1,1,
1,1,1,1,1,1,1,6),(0.,0.0153846153846154,0.0307692307692308,0.0461538461538462,
0.0615384615384615,0.0769230769230769,0.0923076923076923,0.107692307692308,
0.123076923076923,0.138461538461538,0.153846153846154,0.169230769230769,
0.184615384615385,0.2,0.215384615384615,0.230769230769231,0.246153846153846,
0.261538461538462,0.276923076923077,0.292307692307692,0.307692307692308,
0.323076923076923,0.338461538461538,0.353846153846154,0.369230769230769,
0.384615384615385,0.4,0.415384615384615,0.430769230769231,0.446153846153846,
0.461538461538462,0.476923076923077,0.492307692307692,0.507692307692308,
0.523076923076923,0.538461538461538,0.553846153846154,0.569230769230769,
0.584615384615384,0.6,0.615384615384615,0.63076923076923,0.646153846153846,
0.661538461538461,0.676923076923076,0.692307692307692,0.707692307692307,
0.723076923076922,0.738461538461538,0.753846153846153,0.769230769230768,
0.784615384615384,0.799999999999999,0.815384615384614,0.83076923076923,
0.846153846153845,0.86153846153846,0.876923076923076,0.892307692307691,
0.907692307692306,0.923076923076922,0.938461538461537,0.953846153846152,
0.969230769230768,0.984615384615383,1.),.UNSPECIFIED.)
CURVE()
GEOMETRIC_REPRESENTATION_ITEM()
RATIONAL_B_SPLINE_CURVE((1.,1.,1.,1.,1.,1.,1.,1.,1.,1.,1.,1.,1.,1.,1.,1.,
1.,1.,1.,1.,1.,1.,1.,1.,1.,1.,1.,1.,1.,1.,1.,1.,1.,1.,1.,1.,1.,1.,1.,1.,
1.,1.,1.,1.,1.,1.,1.,1.,1.,1.,1.,1.,1.,1.,1.,1.,1.,1.,1.,1.,1.,1.,1.,1.,
1.,1.,1.,1.,1.,1.))
REPRESENTATION_ITEM('')
);
#176=(
BOUNDED_CURVE()
B_SPLINE_CURVE(5,(#26083,#26084,#26085,#26086,#26087,#26088,#26089,#26090,
#26091,#26092,#26093,#26094,#26095,#26096,#26097,#26098,#26099,#26100,#26101,
#26102,#26103,#26104,#26105,#26106,#26107,#26108,#26109,#26110,#26111,#26112,
#26113,#26114,#26115,#26116,#26117,#26118,#26119,#26120,#26121,#26122,#26123,
#26124,#26125,#26126,#26127,#26128,#26129,#26130,#26131,#26132,#26133,#26134,
#26135,#26136,#26137,#26138,#26139,#26140,#26141,#26142,#26143,#26144,#26145,
#26146,#26147,#26148,#26149,#26150,#26151,#26152),.UNSPECIFIED.,.F.,.F.)
B_SPLINE_CURVE_WITH_KNOTS((6,1,1,1,1,1,1,1,1,1,1,1,1,1,1,1,1,1,1,1,1,1,
1,1,1,1,1,1,1,1,1,1,1,1,1,1,1,1,1,1,1,1,1,1,1,1,1,1,1,1,1,1,1,1,1,1,1,1,
1,1,1,1,1,1,1,6),(0.,0.0153846153846154,0.0307692307692308,0.0461538461538462,
0.0615384615384615,0.0769230769230769,0.0923076923076923,0.107692307692308,
0.123076923076923,0.138461538461538,0.153846153846154,0.169230769230769,
0.184615384615385,0.2,0.215384615384615,0.230769230769231,0.246153846153846,
0.261538461538462,0.276923076923077,0.292307692307692,0.307692307692308,
0.323076923076923,0.338461538461538,0.353846153846154,0.369230769230769,
0.384615384615385,0.4,0.415384615384615,0.430769230769231,0.446153846153846,
0.461538461538462,0.476923076923077,0.492307692307692,0.507692307692308,
0.523076923076923,0.538461538461538,0.553846153846154,0.569230769230769,
0.584615384615384,0.6,0.615384615384615,0.63076923076923,0.646153846153846,
0.661538461538461,0.676923076923076,0.692307692307692,0.707692307692307,
0.723076923076922,0.738461538461538,0.753846153846153,0.769230769230768,
0.784615384615384,0.799999999999999,0.815384615384614,0.83076923076923,
0.846153846153845,0.86153846153846,0.876923076923076,0.892307692307691,
0.907692307692306,0.923076923076922,0.938461538461537,0.953846153846152,
0.969230769230768,0.984615384615383,1.),.UNSPECIFIED.)
CURVE()
GEOMETRIC_REPRESENTATION_ITEM()
RATIONAL_B_SPLINE_CURVE((1.,1.,1.,1.,1.,1.,1.,1.,1.,1.,1.,1.,1.,1.,1.,1.,
1.,1.,1.,1.,1.,1.,1.,1.,1.,1.,1.,1.,1.,1.,1.,1.,1.,1.,1.,1.,1.,1.,1.,1.,
1.,1.,1.,1.,1.,1.,1.,1.,1.,1.,1.,1.,1.,1.,1.,1.,1.,1.,1.,1.,1.,1.,1.,1.,
1.,1.,1.,1.,1.,1.))
REPRESENTATION_ITEM('')
);
#177=(
BOUNDED_CURVE()
B_SPLINE_CURVE(5,(#26156,#26157,#26158,#26159,#26160,#26161,#26162,#26163,
#26164,#26165,#26166,#26167,#26168,#26169,#26170,#26171,#26172,#26173,#26174,
#26175,#26176,#26177,#26178,#26179,#26180,#26181,#26182,#26183,#26184,#26185,
#26186,#26187,#26188,#26189,#26190,#26191,#26192,#26193,#26194,#26195,#26196,
#26197,#26198,#26199,#26200,#26201,#26202,#26203,#26204,#26205,#26206,#26207,
#26208,#26209,#26210,#26211,#26212,#26213,#26214,#26215,#26216,#26217,#26218,
#26219,#26220,#26221,#26222,#26223,#26224,#26225),.UNSPECIFIED.,.F.,.F.)
B_SPLINE_CURVE_WITH_KNOTS((6,1,1,1,1,1,1,1,1,1,1,1,1,1,1,1,1,1,1,1,1,1,
1,1,1,1,1,1,1,1,1,1,1,1,1,1,1,1,1,1,1,1,1,1,1,1,1,1,1,1,1,1,1,1,1,1,1,1,
1,1,1,1,1,1,1,6),(0.,0.0153846153846154,0.0307692307692308,0.0461538461538462,
0.0615384615384615,0.0769230769230769,0.0923076923076923,0.107692307692308,
0.123076923076923,0.138461538461538,0.153846153846154,0.169230769230769,
0.184615384615385,0.2,0.215384615384615,0.230769230769231,0.246153846153846,
0.261538461538462,0.276923076923077,0.292307692307692,0.307692307692308,
0.323076923076923,0.338461538461538,0.353846153846154,0.369230769230769,
0.384615384615385,0.4,0.415384615384615,0.430769230769231,0.446153846153846,
0.461538461538462,0.476923076923077,0.492307692307692,0.507692307692308,
0.523076923076923,0.538461538461538,0.553846153846154,0.569230769230769,
0.584615384615384,0.6,0.615384615384615,0.63076923076923,0.646153846153846,
0.661538461538461,0.676923076923076,0.692307692307692,0.707692307692307,
0.723076923076922,0.738461538461538,0.753846153846153,0.769230769230768,
0.784615384615384,0.799999999999999,0.815384615384614,0.83076923076923,
0.846153846153845,0.86153846153846,0.876923076923076,0.892307692307691,
0.907692307692306,0.923076923076922,0.938461538461537,0.953846153846152,
0.969230769230768,0.984615384615383,1.),.UNSPECIFIED.)
CURVE()
GEOMETRIC_REPRESENTATION_ITEM()
RATIONAL_B_SPLINE_CURVE((1.,1.,1.,1.,1.,1.,1.,1.,1.,1.,1.,1.,1.,1.,1.,1.,
1.,1.,1.,1.,1.,1.,1.,1.,1.,1.,1.,1.,1.,1.,1.,1.,1.,1.,1.,1.,1.,1.,1.,1.,
1.,1.,1.,1.,1.,1.,1.,1.,1.,1.,1.,1.,1.,1.,1.,1.,1.,1.,1.,1.,1.,1.,1.,1.,
1.,1.,1.,1.,1.,1.))
REPRESENTATION_ITEM('')
);
#178=(
BOUNDED_CURVE()
B_SPLINE_CURVE(5,(#26229,#26230,#26231,#26232,#26233,#26234,#26235,#26236,
#26237,#26238,#26239,#26240,#26241,#26242,#26243,#26244,#26245,#26246,#26247,
#26248,#26249,#26250,#26251,#26252,#26253,#26254,#26255,#26256,#26257,#26258,
#26259,#26260,#26261,#26262,#26263,#26264,#26265,#26266,#26267,#26268,#26269,
#26270,#26271,#26272,#26273,#26274,#26275,#26276,#26277,#26278,#26279,#26280,
#26281,#26282,#26283,#26284,#26285,#26286,#26287,#26288,#26289,#26290,#26291,
#26292,#26293,#26294,#26295,#26296,#26297,#26298),.UNSPECIFIED.,.F.,.F.)
B_SPLINE_CURVE_WITH_KNOTS((6,1,1,1,1,1,1,1,1,1,1,1,1,1,1,1,1,1,1,1,1,1,
1,1,1,1,1,1,1,1,1,1,1,1,1,1,1,1,1,1,1,1,1,1,1,1,1,1,1,1,1,1,1,1,1,1,1,1,
1,1,1,1,1,1,1,6),(0.,0.0153846153846154,0.0307692307692308,0.0461538461538462,
0.0615384615384615,0.0769230769230769,0.0923076923076923,0.107692307692308,
0.123076923076923,0.138461538461538,0.153846153846154,0.169230769230769,
0.184615384615385,0.2,0.215384615384615,0.230769230769231,0.246153846153846,
0.261538461538462,0.276923076923077,0.292307692307692,0.307692307692308,
0.323076923076923,0.338461538461538,0.353846153846154,0.369230769230769,
0.384615384615385,0.4,0.415384615384615,0.430769230769231,0.446153846153846,
0.461538461538462,0.476923076923077,0.492307692307692,0.507692307692308,
0.523076923076923,0.538461538461538,0.553846153846154,0.569230769230769,
0.584615384615384,0.6,0.615384615384615,0.63076923076923,0.646153846153846,
0.661538461538461,0.676923076923076,0.692307692307692,0.707692307692307,
0.723076923076922,0.738461538461538,0.753846153846153,0.769230769230768,
0.784615384615384,0.799999999999999,0.815384615384614,0.83076923076923,
0.846153846153845,0.86153846153846,0.876923076923076,0.892307692307691,
0.907692307692306,0.923076923076922,0.938461538461537,0.953846153846152,
0.969230769230768,0.984615384615383,1.),.UNSPECIFIED.)
CURVE()
GEOMETRIC_REPRESENTATION_ITEM()
RATIONAL_B_SPLINE_CURVE((1.,1.,1.,1.,1.,1.,1.,1.,1.,1.,1.,1.,1.,1.,1.,1.,
1.,1.,1.,1.,1.,1.,1.,1.,1.,1.,1.,1.,1.,1.,1.,1.,1.,1.,1.,1.,1.,1.,1.,1.,
1.,1.,1.,1.,1.,1.,1.,1.,1.,1.,1.,1.,1.,1.,1.,1.,1.,1.,1.,1.,1.,1.,1.,1.,
1.,1.,1.,1.,1.,1.))
REPRESENTATION_ITEM('')
);
#179=(
BOUNDED_CURVE()
B_SPLINE_CURVE(5,(#26302,#26303,#26304,#26305,#26306,#26307,#26308,#26309,
#26310,#26311,#26312,#26313,#26314,#26315,#26316,#26317,#26318,#26319,#26320,
#26321,#26322,#26323,#26324,#26325,#26326,#26327,#26328,#26329,#26330,#26331,
#26332,#26333,#26334,#26335,#26336,#26337,#26338,#26339,#26340,#26341,#26342,
#26343,#26344,#26345,#26346,#26347,#26348,#26349,#26350,#26351,#26352,#26353,
#26354,#26355,#26356,#26357,#26358,#26359,#26360,#26361,#26362,#26363,#26364,
#26365,#26366,#26367,#26368,#26369,#26370,#26371),.UNSPECIFIED.,.F.,.F.)
B_SPLINE_CURVE_WITH_KNOTS((6,1,1,1,1,1,1,1,1,1,1,1,1,1,1,1,1,1,1,1,1,1,
1,1,1,1,1,1,1,1,1,1,1,1,1,1,1,1,1,1,1,1,1,1,1,1,1,1,1,1,1,1,1,1,1,1,1,1,
1,1,1,1,1,1,1,6),(0.,0.0153846153846154,0.0307692307692308,0.0461538461538462,
0.0615384615384615,0.0769230769230769,0.0923076923076923,0.107692307692308,
0.123076923076923,0.138461538461538,0.153846153846154,0.169230769230769,
0.184615384615385,0.2,0.215384615384615,0.230769230769231,0.246153846153846,
0.261538461538462,0.276923076923077,0.292307692307692,0.307692307692308,
0.323076923076923,0.338461538461538,0.353846153846154,0.369230769230769,
0.384615384615385,0.4,0.415384615384615,0.430769230769231,0.446153846153846,
0.461538461538462,0.476923076923077,0.492307692307692,0.507692307692308,
0.523076923076923,0.538461538461538,0.553846153846154,0.569230769230769,
0.584615384615384,0.6,0.615384615384615,0.63076923076923,0.646153846153846,
0.661538461538461,0.676923076923076,0.692307692307692,0.707692307692307,
0.723076923076922,0.738461538461538,0.753846153846153,0.769230769230768,
0.784615384615384,0.799999999999999,0.815384615384614,0.83076923076923,
0.846153846153845,0.86153846153846,0.876923076923076,0.892307692307691,
0.907692307692306,0.923076923076922,0.938461538461537,0.953846153846152,
0.969230769230768,0.984615384615383,1.),.UNSPECIFIED.)
CURVE()
GEOMETRIC_REPRESENTATION_ITEM()
RATIONAL_B_SPLINE_CURVE((1.,1.,1.,1.,1.,1.,1.,1.,1.,1.,1.,1.,1.,1.,1.,1.,
1.,1.,1.,1.,1.,1.,1.,1.,1.,1.,1.,1.,1.,1.,1.,1.,1.,1.,1.,1.,1.,1.,1.,1.,
1.,1.,1.,1.,1.,1.,1.,1.,1.,1.,1.,1.,1.,1.,1.,1.,1.,1.,1.,1.,1.,1.,1.,1.,
1.,1.,1.,1.,1.,1.))
REPRESENTATION_ITEM('')
);
#180=(
BOUNDED_CURVE()
B_SPLINE_CURVE(5,(#26375,#26376,#26377,#26378,#26379,#26380,#26381,#26382,
#26383,#26384,#26385,#26386,#26387,#26388,#26389,#26390,#26391,#26392,#26393,
#26394,#26395,#26396,#26397,#26398,#26399,#26400,#26401,#26402,#26403,#26404,
#26405,#26406,#26407,#26408,#26409,#26410,#26411,#26412,#26413,#26414,#26415,
#26416,#26417,#26418,#26419,#26420,#26421,#26422,#26423,#26424,#26425,#26426,
#26427,#26428,#26429,#26430,#26431,#26432,#26433,#26434,#26435,#26436,#26437,
#26438,#26439,#26440,#26441,#26442,#26443,#26444),.UNSPECIFIED.,.F.,.F.)
B_SPLINE_CURVE_WITH_KNOTS((6,1,1,1,1,1,1,1,1,1,1,1,1,1,1,1,1,1,1,1,1,1,
1,1,1,1,1,1,1,1,1,1,1,1,1,1,1,1,1,1,1,1,1,1,1,1,1,1,1,1,1,1,1,1,1,1,1,1,
1,1,1,1,1,1,1,6),(0.,0.0153846153846154,0.0307692307692308,0.0461538461538462,
0.0615384615384615,0.0769230769230769,0.0923076923076923,0.107692307692308,
0.123076923076923,0.138461538461538,0.153846153846154,0.169230769230769,
0.184615384615385,0.2,0.215384615384615,0.230769230769231,0.246153846153846,
0.261538461538462,0.276923076923077,0.292307692307692,0.307692307692308,
0.323076923076923,0.338461538461538,0.353846153846154,0.369230769230769,
0.384615384615385,0.4,0.415384615384615,0.430769230769231,0.446153846153846,
0.461538461538462,0.476923076923077,0.492307692307692,0.507692307692308,
0.523076923076923,0.538461538461538,0.553846153846154,0.569230769230769,
0.584615384615384,0.6,0.615384615384615,0.63076923076923,0.646153846153846,
0.661538461538461,0.676923076923076,0.692307692307692,0.707692307692307,
0.723076923076922,0.738461538461538,0.753846153846153,0.769230769230768,
0.784615384615384,0.799999999999999,0.815384615384614,0.83076923076923,
0.846153846153845,0.86153846153846,0.876923076923076,0.892307692307691,
0.907692307692306,0.923076923076922,0.938461538461537,0.953846153846152,
0.969230769230768,0.984615384615383,1.),.UNSPECIFIED.)
CURVE()
GEOMETRIC_REPRESENTATION_ITEM()
RATIONAL_B_SPLINE_CURVE((1.,1.,1.,1.,1.,1.,1.,1.,1.,1.,1.,1.,1.,1.,1.,1.,
1.,1.,1.,1.,1.,1.,1.,1.,1.,1.,1.,1.,1.,1.,1.,1.,1.,1.,1.,1.,1.,1.,1.,1.,
1.,1.,1.,1.,1.,1.,1.,1.,1.,1.,1.,1.,1.,1.,1.,1.,1.,1.,1.,1.,1.,1.,1.,1.,
1.,1.,1.,1.,1.,1.))
REPRESENTATION_ITEM('')
);
#181=(
BOUNDED_CURVE()
B_SPLINE_CURVE(5,(#26448,#26449,#26450,#26451,#26452,#26453,#26454,#26455,
#26456,#26457,#26458,#26459,#26460,#26461,#26462,#26463,#26464,#26465,#26466,
#26467,#26468,#26469,#26470,#26471,#26472,#26473,#26474,#26475,#26476,#26477,
#26478,#26479,#26480,#26481,#26482,#26483,#26484,#26485,#26486,#26487,#26488,
#26489,#26490,#26491,#26492,#26493,#26494,#26495,#26496,#26497,#26498,#26499,
#26500,#26501,#26502,#26503,#26504,#26505,#26506,#26507,#26508,#26509,#26510,
#26511,#26512,#26513,#26514,#26515,#26516,#26517),.UNSPECIFIED.,.F.,.F.)
B_SPLINE_CURVE_WITH_KNOTS((6,1,1,1,1,1,1,1,1,1,1,1,1,1,1,1,1,1,1,1,1,1,
1,1,1,1,1,1,1,1,1,1,1,1,1,1,1,1,1,1,1,1,1,1,1,1,1,1,1,1,1,1,1,1,1,1,1,1,
1,1,1,1,1,1,1,6),(0.,0.0153846153846154,0.0307692307692308,0.0461538461538462,
0.0615384615384615,0.0769230769230769,0.0923076923076923,0.107692307692308,
0.123076923076923,0.138461538461538,0.153846153846154,0.169230769230769,
0.184615384615385,0.2,0.215384615384615,0.230769230769231,0.246153846153846,
0.261538461538462,0.276923076923077,0.292307692307692,0.307692307692308,
0.323076923076923,0.338461538461538,0.353846153846154,0.369230769230769,
0.384615384615385,0.4,0.415384615384615,0.430769230769231,0.446153846153846,
0.461538461538462,0.476923076923077,0.492307692307692,0.507692307692308,
0.523076923076923,0.538461538461538,0.553846153846154,0.569230769230769,
0.584615384615384,0.6,0.615384615384615,0.63076923076923,0.646153846153846,
0.661538461538461,0.676923076923076,0.692307692307692,0.707692307692307,
0.723076923076922,0.738461538461538,0.753846153846153,0.769230769230768,
0.784615384615384,0.799999999999999,0.815384615384614,0.83076923076923,
0.846153846153845,0.86153846153846,0.876923076923076,0.892307692307691,
0.907692307692306,0.923076923076922,0.938461538461537,0.953846153846152,
0.969230769230768,0.984615384615383,1.),.UNSPECIFIED.)
CURVE()
GEOMETRIC_REPRESENTATION_ITEM()
RATIONAL_B_SPLINE_CURVE((1.,1.,1.,1.,1.,1.,1.,1.,1.,1.,1.,1.,1.,1.,1.,1.,
1.,1.,1.,1.,1.,1.,1.,1.,1.,1.,1.,1.,1.,1.,1.,1.,1.,1.,1.,1.,1.,1.,1.,1.,
1.,1.,1.,1.,1.,1.,1.,1.,1.,1.,1.,1.,1.,1.,1.,1.,1.,1.,1.,1.,1.,1.,1.,1.,
1.,1.,1.,1.,1.,1.))
REPRESENTATION_ITEM('')
);
#182=(
BOUNDED_CURVE()
B_SPLINE_CURVE(5,(#26521,#26522,#26523,#26524,#26525,#26526,#26527,#26528,
#26529,#26530,#26531,#26532,#26533,#26534,#26535,#26536,#26537,#26538,#26539,
#26540,#26541,#26542,#26543,#26544,#26545,#26546,#26547,#26548,#26549,#26550,
#26551,#26552,#26553,#26554,#26555,#26556,#26557,#26558,#26559,#26560,#26561,
#26562,#26563,#26564,#26565,#26566,#26567,#26568,#26569,#26570,#26571,#26572,
#26573,#26574,#26575,#26576,#26577,#26578,#26579,#26580,#26581,#26582,#26583,
#26584,#26585,#26586,#26587,#26588,#26589,#26590),.UNSPECIFIED.,.F.,.F.)
B_SPLINE_CURVE_WITH_KNOTS((6,1,1,1,1,1,1,1,1,1,1,1,1,1,1,1,1,1,1,1,1,1,
1,1,1,1,1,1,1,1,1,1,1,1,1,1,1,1,1,1,1,1,1,1,1,1,1,1,1,1,1,1,1,1,1,1,1,1,
1,1,1,1,1,1,1,6),(0.,0.0153846153846154,0.0307692307692308,0.0461538461538462,
0.0615384615384615,0.0769230769230769,0.0923076923076923,0.107692307692308,
0.123076923076923,0.138461538461538,0.153846153846154,0.169230769230769,
0.184615384615385,0.2,0.215384615384615,0.230769230769231,0.246153846153846,
0.261538461538462,0.276923076923077,0.292307692307692,0.307692307692308,
0.323076923076923,0.338461538461538,0.353846153846154,0.369230769230769,
0.384615384615385,0.4,0.415384615384615,0.430769230769231,0.446153846153846,
0.461538461538462,0.476923076923077,0.492307692307692,0.507692307692308,
0.523076923076923,0.538461538461538,0.553846153846154,0.569230769230769,
0.584615384615384,0.6,0.615384615384615,0.63076923076923,0.646153846153846,
0.661538461538461,0.676923076923076,0.692307692307692,0.707692307692307,
0.723076923076922,0.738461538461538,0.753846153846153,0.769230769230768,
0.784615384615384,0.799999999999999,0.815384615384614,0.83076923076923,
0.846153846153845,0.86153846153846,0.876923076923076,0.892307692307691,
0.907692307692306,0.923076923076922,0.938461538461537,0.953846153846152,
0.969230769230768,0.984615384615383,1.),.UNSPECIFIED.)
CURVE()
GEOMETRIC_REPRESENTATION_ITEM()
RATIONAL_B_SPLINE_CURVE((1.,1.,1.,1.,1.,1.,1.,1.,1.,1.,1.,1.,1.,1.,1.,1.,
1.,1.,1.,1.,1.,1.,1.,1.,1.,1.,1.,1.,1.,1.,1.,1.,1.,1.,1.,1.,1.,1.,1.,1.,
1.,1.,1.,1.,1.,1.,1.,1.,1.,1.,1.,1.,1.,1.,1.,1.,1.,1.,1.,1.,1.,1.,1.,1.,
1.,1.,1.,1.,1.,1.))
REPRESENTATION_ITEM('')
);
#183=(
BOUNDED_CURVE()
B_SPLINE_CURVE(5,(#26594,#26595,#26596,#26597,#26598,#26599,#26600,#26601,
#26602,#26603,#26604,#26605,#26606,#26607,#26608,#26609,#26610,#26611,#26612,
#26613,#26614,#26615,#26616,#26617,#26618,#26619,#26620,#26621,#26622,#26623,
#26624,#26625,#26626,#26627,#26628,#26629,#26630,#26631,#26632,#26633,#26634,
#26635,#26636,#26637,#26638,#26639,#26640,#26641,#26642,#26643,#26644,#26645,
#26646,#26647,#26648,#26649,#26650,#26651,#26652,#26653,#26654,#26655,#26656,
#26657,#26658,#26659,#26660,#26661,#26662,#26663),.UNSPECIFIED.,.F.,.F.)
B_SPLINE_CURVE_WITH_KNOTS((6,1,1,1,1,1,1,1,1,1,1,1,1,1,1,1,1,1,1,1,1,1,
1,1,1,1,1,1,1,1,1,1,1,1,1,1,1,1,1,1,1,1,1,1,1,1,1,1,1,1,1,1,1,1,1,1,1,1,
1,1,1,1,1,1,1,6),(0.,0.0153846153846154,0.0307692307692308,0.0461538461538462,
0.0615384615384615,0.0769230769230769,0.0923076923076923,0.107692307692308,
0.123076923076923,0.138461538461538,0.153846153846154,0.169230769230769,
0.184615384615385,0.2,0.215384615384615,0.230769230769231,0.246153846153846,
0.261538461538462,0.276923076923077,0.292307692307692,0.307692307692308,
0.323076923076923,0.338461538461538,0.353846153846154,0.369230769230769,
0.384615384615385,0.4,0.415384615384615,0.430769230769231,0.446153846153846,
0.461538461538462,0.476923076923077,0.492307692307692,0.507692307692308,
0.523076923076923,0.538461538461538,0.553846153846154,0.569230769230769,
0.584615384615384,0.6,0.615384615384615,0.63076923076923,0.646153846153846,
0.661538461538461,0.676923076923076,0.692307692307692,0.707692307692307,
0.723076923076922,0.738461538461538,0.753846153846153,0.769230769230768,
0.784615384615384,0.799999999999999,0.815384615384614,0.83076923076923,
0.846153846153845,0.86153846153846,0.876923076923076,0.892307692307691,
0.907692307692306,0.923076923076922,0.938461538461537,0.953846153846152,
0.969230769230768,0.984615384615383,1.),.UNSPECIFIED.)
CURVE()
GEOMETRIC_REPRESENTATION_ITEM()
RATIONAL_B_SPLINE_CURVE((1.,1.,1.,1.,1.,1.,1.,1.,1.,1.,1.,1.,1.,1.,1.,1.,
1.,1.,1.,1.,1.,1.,1.,1.,1.,1.,1.,1.,1.,1.,1.,1.,1.,1.,1.,1.,1.,1.,1.,1.,
1.,1.,1.,1.,1.,1.,1.,1.,1.,1.,1.,1.,1.,1.,1.,1.,1.,1.,1.,1.,1.,1.,1.,1.,
1.,1.,1.,1.,1.,1.))
REPRESENTATION_ITEM('')
);
#184=(
BOUNDED_CURVE()
B_SPLINE_CURVE(5,(#26667,#26668,#26669,#26670,#26671,#26672,#26673,#26674,
#26675,#26676,#26677,#26678,#26679,#26680,#26681,#26682,#26683,#26684,#26685,
#26686,#26687,#26688,#26689,#26690,#26691,#26692,#26693,#26694,#26695,#26696,
#26697,#26698,#26699,#26700,#26701,#26702,#26703,#26704,#26705,#26706,#26707,
#26708,#26709,#26710,#26711,#26712,#26713,#26714,#26715,#26716,#26717,#26718,
#26719,#26720,#26721,#26722,#26723,#26724,#26725,#26726,#26727,#26728,#26729,
#26730,#26731,#26732,#26733,#26734,#26735,#26736),.UNSPECIFIED.,.F.,.F.)
B_SPLINE_CURVE_WITH_KNOTS((6,1,1,1,1,1,1,1,1,1,1,1,1,1,1,1,1,1,1,1,1,1,
1,1,1,1,1,1,1,1,1,1,1,1,1,1,1,1,1,1,1,1,1,1,1,1,1,1,1,1,1,1,1,1,1,1,1,1,
1,1,1,1,1,1,1,6),(0.,0.0153846153846154,0.0307692307692308,0.0461538461538462,
0.0615384615384615,0.0769230769230769,0.0923076923076923,0.107692307692308,
0.123076923076923,0.138461538461538,0.153846153846154,0.169230769230769,
0.184615384615385,0.2,0.215384615384615,0.230769230769231,0.246153846153846,
0.261538461538462,0.276923076923077,0.292307692307692,0.307692307692308,
0.323076923076923,0.338461538461538,0.353846153846154,0.369230769230769,
0.384615384615385,0.4,0.415384615384615,0.430769230769231,0.446153846153846,
0.461538461538462,0.476923076923077,0.492307692307692,0.507692307692308,
0.523076923076923,0.538461538461538,0.553846153846154,0.569230769230769,
0.584615384615384,0.6,0.615384615384615,0.63076923076923,0.646153846153846,
0.661538461538461,0.676923076923076,0.692307692307692,0.707692307692307,
0.723076923076922,0.738461538461538,0.753846153846153,0.769230769230768,
0.784615384615384,0.799999999999999,0.815384615384614,0.83076923076923,
0.846153846153845,0.86153846153846,0.876923076923076,0.892307692307691,
0.907692307692306,0.923076923076922,0.938461538461537,0.953846153846152,
0.969230769230768,0.984615384615383,1.),.UNSPECIFIED.)
CURVE()
GEOMETRIC_REPRESENTATION_ITEM()
RATIONAL_B_SPLINE_CURVE((1.,1.,1.,1.,1.,1.,1.,1.,1.,1.,1.,1.,1.,1.,1.,1.,
1.,1.,1.,1.,1.,1.,1.,1.,1.,1.,1.,1.,1.,1.,1.,1.,1.,1.,1.,1.,1.,1.,1.,1.,
1.,1.,1.,1.,1.,1.,1.,1.,1.,1.,1.,1.,1.,1.,1.,1.,1.,1.,1.,1.,1.,1.,1.,1.,
1.,1.,1.,1.,1.,1.))
REPRESENTATION_ITEM('')
);
#185=(
BOUNDED_CURVE()
B_SPLINE_CURVE(5,(#26740,#26741,#26742,#26743,#26744,#26745,#26746,#26747,
#26748,#26749,#26750,#26751,#26752,#26753,#26754,#26755,#26756,#26757,#26758,
#26759,#26760,#26761,#26762,#26763,#26764,#26765,#26766,#26767,#26768,#26769,
#26770,#26771,#26772,#26773,#26774,#26775,#26776,#26777,#26778,#26779,#26780,
#26781,#26782,#26783,#26784,#26785,#26786,#26787,#26788,#26789,#26790,#26791,
#26792,#26793,#26794,#26795,#26796,#26797,#26798,#26799,#26800,#26801,#26802,
#26803,#26804,#26805,#26806,#26807,#26808,#26809),.UNSPECIFIED.,.F.,.F.)
B_SPLINE_CURVE_WITH_KNOTS((6,1,1,1,1,1,1,1,1,1,1,1,1,1,1,1,1,1,1,1,1,1,
1,1,1,1,1,1,1,1,1,1,1,1,1,1,1,1,1,1,1,1,1,1,1,1,1,1,1,1,1,1,1,1,1,1,1,1,
1,1,1,1,1,1,1,6),(0.,0.0153846153846154,0.0307692307692308,0.0461538461538462,
0.0615384615384615,0.0769230769230769,0.0923076923076923,0.107692307692308,
0.123076923076923,0.138461538461538,0.153846153846154,0.169230769230769,
0.184615384615385,0.2,0.215384615384615,0.230769230769231,0.246153846153846,
0.261538461538462,0.276923076923077,0.292307692307692,0.307692307692308,
0.323076923076923,0.338461538461538,0.353846153846154,0.369230769230769,
0.384615384615385,0.4,0.415384615384615,0.430769230769231,0.446153846153846,
0.461538461538462,0.476923076923077,0.492307692307692,0.507692307692308,
0.523076923076923,0.538461538461538,0.553846153846154,0.569230769230769,
0.584615384615384,0.6,0.615384615384615,0.63076923076923,0.646153846153846,
0.661538461538461,0.676923076923076,0.692307692307692,0.707692307692307,
0.723076923076922,0.738461538461538,0.753846153846153,0.769230769230768,
0.784615384615384,0.799999999999999,0.815384615384614,0.83076923076923,
0.846153846153845,0.86153846153846,0.876923076923076,0.892307692307691,
0.907692307692306,0.923076923076922,0.938461538461537,0.953846153846152,
0.969230769230768,0.984615384615383,1.),.UNSPECIFIED.)
CURVE()
GEOMETRIC_REPRESENTATION_ITEM()
RATIONAL_B_SPLINE_CURVE((1.,1.,1.,1.,1.,1.,1.,1.,1.,1.,1.,1.,1.,1.,1.,1.,
1.,1.,1.,1.,1.,1.,1.,1.,1.,1.,1.,1.,1.,1.,1.,1.,1.,1.,1.,1.,1.,1.,1.,1.,
1.,1.,1.,1.,1.,1.,1.,1.,1.,1.,1.,1.,1.,1.,1.,1.,1.,1.,1.,1.,1.,1.,1.,1.,
1.,1.,1.,1.,1.,1.))
REPRESENTATION_ITEM('')
);
#186=(
BOUNDED_CURVE()
B_SPLINE_CURVE(5,(#26813,#26814,#26815,#26816,#26817,#26818,#26819,#26820,
#26821,#26822,#26823,#26824,#26825,#26826,#26827,#26828,#26829,#26830,#26831,
#26832,#26833,#26834,#26835,#26836,#26837,#26838,#26839,#26840,#26841,#26842,
#26843,#26844,#26845,#26846,#26847,#26848,#26849,#26850,#26851,#26852,#26853,
#26854,#26855,#26856,#26857,#26858,#26859,#26860,#26861,#26862,#26863,#26864,
#26865,#26866,#26867,#26868,#26869,#26870,#26871,#26872,#26873,#26874,#26875,
#26876,#26877,#26878,#26879,#26880,#26881,#26882),.UNSPECIFIED.,.F.,.F.)
B_SPLINE_CURVE_WITH_KNOTS((6,1,1,1,1,1,1,1,1,1,1,1,1,1,1,1,1,1,1,1,1,1,
1,1,1,1,1,1,1,1,1,1,1,1,1,1,1,1,1,1,1,1,1,1,1,1,1,1,1,1,1,1,1,1,1,1,1,1,
1,1,1,1,1,1,1,6),(0.,0.0153846153846154,0.0307692307692308,0.0461538461538462,
0.0615384615384615,0.0769230769230769,0.0923076923076923,0.107692307692308,
0.123076923076923,0.138461538461538,0.153846153846154,0.169230769230769,
0.184615384615385,0.2,0.215384615384615,0.230769230769231,0.246153846153846,
0.261538461538462,0.276923076923077,0.292307692307692,0.307692307692308,
0.323076923076923,0.338461538461538,0.353846153846154,0.369230769230769,
0.384615384615385,0.4,0.415384615384615,0.430769230769231,0.446153846153846,
0.461538461538462,0.476923076923077,0.492307692307692,0.507692307692308,
0.523076923076923,0.538461538461538,0.553846153846154,0.569230769230769,
0.584615384615384,0.6,0.615384615384615,0.63076923076923,0.646153846153846,
0.661538461538461,0.676923076923076,0.692307692307692,0.707692307692307,
0.723076923076922,0.738461538461538,0.753846153846153,0.769230769230768,
0.784615384615384,0.799999999999999,0.815384615384614,0.83076923076923,
0.846153846153845,0.86153846153846,0.876923076923076,0.892307692307691,
0.907692307692306,0.923076923076922,0.938461538461537,0.953846153846152,
0.969230769230768,0.984615384615383,1.),.UNSPECIFIED.)
CURVE()
GEOMETRIC_REPRESENTATION_ITEM()
RATIONAL_B_SPLINE_CURVE((1.,1.,1.,1.,1.,1.,1.,1.,1.,1.,1.,1.,1.,1.,1.,1.,
1.,1.,1.,1.,1.,1.,1.,1.,1.,1.,1.,1.,1.,1.,1.,1.,1.,1.,1.,1.,1.,1.,1.,1.,
1.,1.,1.,1.,1.,1.,1.,1.,1.,1.,1.,1.,1.,1.,1.,1.,1.,1.,1.,1.,1.,1.,1.,1.,
1.,1.,1.,1.,1.,1.))
REPRESENTATION_ITEM('')
);
#187=(
BOUNDED_CURVE()
B_SPLINE_CURVE(5,(#26886,#26887,#26888,#26889,#26890,#26891,#26892,#26893,
#26894,#26895,#26896,#26897,#26898,#26899,#26900,#26901,#26902,#26903,#26904,
#26905,#26906,#26907,#26908,#26909,#26910,#26911,#26912,#26913,#26914,#26915,
#26916,#26917,#26918,#26919,#26920,#26921,#26922,#26923,#26924,#26925,#26926,
#26927,#26928,#26929,#26930,#26931,#26932,#26933,#26934,#26935,#26936,#26937,
#26938,#26939,#26940,#26941,#26942,#26943,#26944,#26945,#26946,#26947,#26948,
#26949,#26950,#26951,#26952,#26953,#26954,#26955),.UNSPECIFIED.,.F.,.F.)
B_SPLINE_CURVE_WITH_KNOTS((6,1,1,1,1,1,1,1,1,1,1,1,1,1,1,1,1,1,1,1,1,1,
1,1,1,1,1,1,1,1,1,1,1,1,1,1,1,1,1,1,1,1,1,1,1,1,1,1,1,1,1,1,1,1,1,1,1,1,
1,1,1,1,1,1,1,6),(0.,0.0153846153846154,0.0307692307692308,0.0461538461538462,
0.0615384615384615,0.0769230769230769,0.0923076923076923,0.107692307692308,
0.123076923076923,0.138461538461538,0.153846153846154,0.169230769230769,
0.184615384615385,0.2,0.215384615384615,0.230769230769231,0.246153846153846,
0.261538461538462,0.276923076923077,0.292307692307692,0.307692307692308,
0.323076923076923,0.338461538461538,0.353846153846154,0.369230769230769,
0.384615384615385,0.4,0.415384615384615,0.430769230769231,0.446153846153846,
0.461538461538462,0.476923076923077,0.492307692307692,0.507692307692308,
0.523076923076923,0.538461538461538,0.553846153846154,0.569230769230769,
0.584615384615384,0.6,0.615384615384615,0.63076923076923,0.646153846153846,
0.661538461538461,0.676923076923076,0.692307692307692,0.707692307692307,
0.723076923076922,0.738461538461538,0.753846153846153,0.769230769230768,
0.784615384615384,0.799999999999999,0.815384615384614,0.83076923076923,
0.846153846153845,0.86153846153846,0.876923076923076,0.892307692307691,
0.907692307692306,0.923076923076922,0.938461538461537,0.953846153846152,
0.969230769230768,0.984615384615383,1.),.UNSPECIFIED.)
CURVE()
GEOMETRIC_REPRESENTATION_ITEM()
RATIONAL_B_SPLINE_CURVE((1.,1.,1.,1.,1.,1.,1.,1.,1.,1.,1.,1.,1.,1.,1.,1.,
1.,1.,1.,1.,1.,1.,1.,1.,1.,1.,1.,1.,1.,1.,1.,1.,1.,1.,1.,1.,1.,1.,1.,1.,
1.,1.,1.,1.,1.,1.,1.,1.,1.,1.,1.,1.,1.,1.,1.,1.,1.,1.,1.,1.,1.,1.,1.,1.,
1.,1.,1.,1.,1.,1.))
REPRESENTATION_ITEM('')
);
#188=(
BOUNDED_CURVE()
B_SPLINE_CURVE(5,(#26959,#26960,#26961,#26962,#26963,#26964,#26965,#26966,
#26967,#26968,#26969,#26970,#26971,#26972,#26973,#26974,#26975,#26976,#26977,
#26978,#26979,#26980,#26981,#26982,#26983,#26984,#26985,#26986,#26987,#26988,
#26989,#26990,#26991,#26992,#26993,#26994,#26995,#26996,#26997,#26998,#26999,
#27000,#27001,#27002,#27003,#27004,#27005,#27006,#27007,#27008,#27009,#27010,
#27011,#27012,#27013,#27014,#27015,#27016,#27017,#27018,#27019,#27020,#27021,
#27022,#27023,#27024,#27025,#27026,#27027,#27028),.UNSPECIFIED.,.F.,.F.)
B_SPLINE_CURVE_WITH_KNOTS((6,1,1,1,1,1,1,1,1,1,1,1,1,1,1,1,1,1,1,1,1,1,
1,1,1,1,1,1,1,1,1,1,1,1,1,1,1,1,1,1,1,1,1,1,1,1,1,1,1,1,1,1,1,1,1,1,1,1,
1,1,1,1,1,1,1,6),(0.,0.0153846153846154,0.0307692307692308,0.0461538461538462,
0.0615384615384615,0.0769230769230769,0.0923076923076923,0.107692307692308,
0.123076923076923,0.138461538461538,0.153846153846154,0.169230769230769,
0.184615384615385,0.2,0.215384615384615,0.230769230769231,0.246153846153846,
0.261538461538462,0.276923076923077,0.292307692307692,0.307692307692308,
0.323076923076923,0.338461538461538,0.353846153846154,0.369230769230769,
0.384615384615385,0.4,0.415384615384615,0.430769230769231,0.446153846153846,
0.461538461538462,0.476923076923077,0.492307692307692,0.507692307692308,
0.523076923076923,0.538461538461538,0.553846153846154,0.569230769230769,
0.584615384615384,0.6,0.615384615384615,0.63076923076923,0.646153846153846,
0.661538461538461,0.676923076923076,0.692307692307692,0.707692307692307,
0.723076923076922,0.738461538461538,0.753846153846153,0.769230769230768,
0.784615384615384,0.799999999999999,0.815384615384614,0.83076923076923,
0.846153846153845,0.86153846153846,0.876923076923076,0.892307692307691,
0.907692307692306,0.923076923076922,0.938461538461537,0.953846153846152,
0.969230769230768,0.984615384615383,1.),.UNSPECIFIED.)
CURVE()
GEOMETRIC_REPRESENTATION_ITEM()
RATIONAL_B_SPLINE_CURVE((1.,1.,1.,1.,1.,1.,1.,1.,1.,1.,1.,1.,1.,1.,1.,1.,
1.,1.,1.,1.,1.,1.,1.,1.,1.,1.,1.,1.,1.,1.,1.,1.,1.,1.,1.,1.,1.,1.,1.,1.,
1.,1.,1.,1.,1.,1.,1.,1.,1.,1.,1.,1.,1.,1.,1.,1.,1.,1.,1.,1.,1.,1.,1.,1.,
1.,1.,1.,1.,1.,1.))
REPRESENTATION_ITEM('')
);
#189=(
BOUNDED_CURVE()
B_SPLINE_CURVE(5,(#27032,#27033,#27034,#27035,#27036,#27037,#27038,#27039,
#27040,#27041,#27042,#27043,#27044,#27045,#27046,#27047,#27048,#27049,#27050,
#27051,#27052,#27053,#27054,#27055,#27056,#27057,#27058,#27059,#27060,#27061,
#27062,#27063,#27064,#27065,#27066,#27067,#27068,#27069,#27070,#27071,#27072,
#27073,#27074,#27075,#27076,#27077,#27078,#27079,#27080,#27081,#27082,#27083,
#27084,#27085,#27086,#27087,#27088,#27089,#27090,#27091,#27092,#27093,#27094,
#27095,#27096,#27097,#27098,#27099,#27100,#27101),.UNSPECIFIED.,.F.,.F.)
B_SPLINE_CURVE_WITH_KNOTS((6,1,1,1,1,1,1,1,1,1,1,1,1,1,1,1,1,1,1,1,1,1,
1,1,1,1,1,1,1,1,1,1,1,1,1,1,1,1,1,1,1,1,1,1,1,1,1,1,1,1,1,1,1,1,1,1,1,1,
1,1,1,1,1,1,1,6),(0.,0.0153846153846154,0.0307692307692308,0.0461538461538462,
0.0615384615384615,0.0769230769230769,0.0923076923076923,0.107692307692308,
0.123076923076923,0.138461538461538,0.153846153846154,0.169230769230769,
0.184615384615385,0.2,0.215384615384615,0.230769230769231,0.246153846153846,
0.261538461538462,0.276923076923077,0.292307692307692,0.307692307692308,
0.323076923076923,0.338461538461538,0.353846153846154,0.369230769230769,
0.384615384615385,0.4,0.415384615384615,0.430769230769231,0.446153846153846,
0.461538461538462,0.476923076923077,0.492307692307692,0.507692307692308,
0.523076923076923,0.538461538461538,0.553846153846154,0.569230769230769,
0.584615384615384,0.6,0.615384615384615,0.63076923076923,0.646153846153846,
0.661538461538461,0.676923076923076,0.692307692307692,0.707692307692307,
0.723076923076922,0.738461538461538,0.753846153846153,0.769230769230768,
0.784615384615384,0.799999999999999,0.815384615384614,0.83076923076923,
0.846153846153845,0.86153846153846,0.876923076923076,0.892307692307691,
0.907692307692306,0.923076923076922,0.938461538461537,0.953846153846152,
0.969230769230768,0.984615384615383,1.),.UNSPECIFIED.)
CURVE()
GEOMETRIC_REPRESENTATION_ITEM()
RATIONAL_B_SPLINE_CURVE((1.,1.,1.,1.,1.,1.,1.,1.,1.,1.,1.,1.,1.,1.,1.,1.,
1.,1.,1.,1.,1.,1.,1.,1.,1.,1.,1.,1.,1.,1.,1.,1.,1.,1.,1.,1.,1.,1.,1.,1.,
1.,1.,1.,1.,1.,1.,1.,1.,1.,1.,1.,1.,1.,1.,1.,1.,1.,1.,1.,1.,1.,1.,1.,1.,
1.,1.,1.,1.,1.,1.))
REPRESENTATION_ITEM('')
);
#190=(
BOUNDED_CURVE()
B_SPLINE_CURVE(5,(#27105,#27106,#27107,#27108,#27109,#27110,#27111,#27112,
#27113,#27114,#27115,#27116,#27117,#27118,#27119,#27120,#27121,#27122,#27123,
#27124,#27125,#27126,#27127,#27128,#27129,#27130,#27131,#27132,#27133,#27134,
#27135,#27136,#27137,#27138,#27139,#27140,#27141,#27142,#27143,#27144,#27145,
#27146,#27147,#27148,#27149,#27150,#27151,#27152,#27153,#27154,#27155,#27156,
#27157,#27158,#27159,#27160,#27161,#27162,#27163,#27164,#27165,#27166,#27167,
#27168,#27169,#27170,#27171,#27172,#27173,#27174),.UNSPECIFIED.,.F.,.F.)
B_SPLINE_CURVE_WITH_KNOTS((6,1,1,1,1,1,1,1,1,1,1,1,1,1,1,1,1,1,1,1,1,1,
1,1,1,1,1,1,1,1,1,1,1,1,1,1,1,1,1,1,1,1,1,1,1,1,1,1,1,1,1,1,1,1,1,1,1,1,
1,1,1,1,1,1,1,6),(0.,0.0153846153846154,0.0307692307692308,0.0461538461538462,
0.0615384615384615,0.0769230769230769,0.0923076923076923,0.107692307692308,
0.123076923076923,0.138461538461538,0.153846153846154,0.169230769230769,
0.184615384615385,0.2,0.215384615384615,0.230769230769231,0.246153846153846,
0.261538461538462,0.276923076923077,0.292307692307692,0.307692307692308,
0.323076923076923,0.338461538461538,0.353846153846154,0.369230769230769,
0.384615384615385,0.4,0.415384615384615,0.430769230769231,0.446153846153846,
0.461538461538462,0.476923076923077,0.492307692307692,0.507692307692308,
0.523076923076923,0.538461538461538,0.553846153846154,0.569230769230769,
0.584615384615384,0.6,0.615384615384615,0.63076923076923,0.646153846153846,
0.661538461538461,0.676923076923076,0.692307692307692,0.707692307692307,
0.723076923076922,0.738461538461538,0.753846153846153,0.769230769230768,
0.784615384615384,0.799999999999999,0.815384615384614,0.83076923076923,
0.846153846153845,0.86153846153846,0.876923076923076,0.892307692307691,
0.907692307692306,0.923076923076922,0.938461538461537,0.953846153846152,
0.969230769230768,0.984615384615383,1.),.UNSPECIFIED.)
CURVE()
GEOMETRIC_REPRESENTATION_ITEM()
RATIONAL_B_SPLINE_CURVE((1.,1.,1.,1.,1.,1.,1.,1.,1.,1.,1.,1.,1.,1.,1.,1.,
1.,1.,1.,1.,1.,1.,1.,1.,1.,1.,1.,1.,1.,1.,1.,1.,1.,1.,1.,1.,1.,1.,1.,1.,
1.,1.,1.,1.,1.,1.,1.,1.,1.,1.,1.,1.,1.,1.,1.,1.,1.,1.,1.,1.,1.,1.,1.,1.,
1.,1.,1.,1.,1.,1.))
REPRESENTATION_ITEM('')
);
#191=(
BOUNDED_CURVE()
B_SPLINE_CURVE(5,(#27178,#27179,#27180,#27181,#27182,#27183,#27184,#27185,
#27186,#27187,#27188,#27189,#27190,#27191,#27192,#27193,#27194,#27195,#27196,
#27197,#27198,#27199,#27200,#27201,#27202,#27203,#27204,#27205,#27206,#27207,
#27208,#27209,#27210,#27211,#27212,#27213,#27214,#27215,#27216,#27217,#27218,
#27219,#27220,#27221,#27222,#27223,#27224,#27225,#27226,#27227,#27228,#27229,
#27230,#27231,#27232,#27233,#27234,#27235,#27236,#27237,#27238,#27239,#27240,
#27241,#27242,#27243,#27244,#27245,#27246,#27247),.UNSPECIFIED.,.F.,.F.)
B_SPLINE_CURVE_WITH_KNOTS((6,1,1,1,1,1,1,1,1,1,1,1,1,1,1,1,1,1,1,1,1,1,
1,1,1,1,1,1,1,1,1,1,1,1,1,1,1,1,1,1,1,1,1,1,1,1,1,1,1,1,1,1,1,1,1,1,1,1,
1,1,1,1,1,1,1,6),(0.,0.0153846153846154,0.0307692307692308,0.0461538461538462,
0.0615384615384615,0.0769230769230769,0.0923076923076923,0.107692307692308,
0.123076923076923,0.138461538461538,0.153846153846154,0.169230769230769,
0.184615384615385,0.2,0.215384615384615,0.230769230769231,0.246153846153846,
0.261538461538462,0.276923076923077,0.292307692307692,0.307692307692308,
0.323076923076923,0.338461538461538,0.353846153846154,0.369230769230769,
0.384615384615385,0.4,0.415384615384615,0.430769230769231,0.446153846153846,
0.461538461538462,0.476923076923077,0.492307692307692,0.507692307692308,
0.523076923076923,0.538461538461538,0.553846153846154,0.569230769230769,
0.584615384615384,0.6,0.615384615384615,0.63076923076923,0.646153846153846,
0.661538461538461,0.676923076923076,0.692307692307692,0.707692307692307,
0.723076923076922,0.738461538461538,0.753846153846153,0.769230769230768,
0.784615384615384,0.799999999999999,0.815384615384614,0.83076923076923,
0.846153846153845,0.86153846153846,0.876923076923076,0.892307692307691,
0.907692307692306,0.923076923076922,0.938461538461537,0.953846153846152,
0.969230769230768,0.984615384615383,1.),.UNSPECIFIED.)
CURVE()
GEOMETRIC_REPRESENTATION_ITEM()
RATIONAL_B_SPLINE_CURVE((1.,1.,1.,1.,1.,1.,1.,1.,1.,1.,1.,1.,1.,1.,1.,1.,
1.,1.,1.,1.,1.,1.,1.,1.,1.,1.,1.,1.,1.,1.,1.,1.,1.,1.,1.,1.,1.,1.,1.,1.,
1.,1.,1.,1.,1.,1.,1.,1.,1.,1.,1.,1.,1.,1.,1.,1.,1.,1.,1.,1.,1.,1.,1.,1.,
1.,1.,1.,1.,1.,1.))
REPRESENTATION_ITEM('')
);
#192=(
BOUNDED_CURVE()
B_SPLINE_CURVE(5,(#27251,#27252,#27253,#27254,#27255,#27256,#27257,#27258,
#27259,#27260,#27261,#27262,#27263,#27264,#27265,#27266,#27267,#27268,#27269,
#27270,#27271,#27272,#27273,#27274,#27275,#27276,#27277,#27278,#27279,#27280,
#27281,#27282,#27283,#27284,#27285,#27286,#27287,#27288,#27289,#27290,#27291,
#27292,#27293,#27294,#27295,#27296,#27297,#27298,#27299,#27300,#27301,#27302,
#27303,#27304,#27305,#27306,#27307,#27308,#27309,#27310,#27311,#27312,#27313,
#27314,#27315,#27316,#27317,#27318,#27319,#27320),.UNSPECIFIED.,.F.,.F.)
B_SPLINE_CURVE_WITH_KNOTS((6,1,1,1,1,1,1,1,1,1,1,1,1,1,1,1,1,1,1,1,1,1,
1,1,1,1,1,1,1,1,1,1,1,1,1,1,1,1,1,1,1,1,1,1,1,1,1,1,1,1,1,1,1,1,1,1,1,1,
1,1,1,1,1,1,1,6),(0.,0.0153846153846154,0.0307692307692308,0.0461538461538462,
0.0615384615384615,0.0769230769230769,0.0923076923076923,0.107692307692308,
0.123076923076923,0.138461538461538,0.153846153846154,0.169230769230769,
0.184615384615385,0.2,0.215384615384615,0.230769230769231,0.246153846153846,
0.261538461538462,0.276923076923077,0.292307692307692,0.307692307692308,
0.323076923076923,0.338461538461538,0.353846153846154,0.369230769230769,
0.384615384615385,0.4,0.415384615384615,0.430769230769231,0.446153846153846,
0.461538461538462,0.476923076923077,0.492307692307692,0.507692307692308,
0.523076923076923,0.538461538461538,0.553846153846154,0.569230769230769,
0.584615384615384,0.6,0.615384615384615,0.63076923076923,0.646153846153846,
0.661538461538461,0.676923076923076,0.692307692307692,0.707692307692307,
0.723076923076922,0.738461538461538,0.753846153846153,0.769230769230768,
0.784615384615384,0.799999999999999,0.815384615384614,0.83076923076923,
0.846153846153845,0.86153846153846,0.876923076923076,0.892307692307691,
0.907692307692306,0.923076923076922,0.938461538461537,0.953846153846152,
0.969230769230768,0.984615384615383,1.),.UNSPECIFIED.)
CURVE()
GEOMETRIC_REPRESENTATION_ITEM()
RATIONAL_B_SPLINE_CURVE((1.,1.,1.,1.,1.,1.,1.,1.,1.,1.,1.,1.,1.,1.,1.,1.,
1.,1.,1.,1.,1.,1.,1.,1.,1.,1.,1.,1.,1.,1.,1.,1.,1.,1.,1.,1.,1.,1.,1.,1.,
1.,1.,1.,1.,1.,1.,1.,1.,1.,1.,1.,1.,1.,1.,1.,1.,1.,1.,1.,1.,1.,1.,1.,1.,
1.,1.,1.,1.,1.,1.))
REPRESENTATION_ITEM('')
);
#193=(
BOUNDED_CURVE()
B_SPLINE_CURVE(5,(#27324,#27325,#27326,#27327,#27328,#27329,#27330,#27331,
#27332,#27333,#27334,#27335,#27336,#27337,#27338,#27339,#27340,#27341,#27342,
#27343,#27344,#27345,#27346,#27347,#27348,#27349,#27350,#27351,#27352,#27353,
#27354,#27355,#27356,#27357,#27358,#27359,#27360,#27361,#27362,#27363,#27364,
#27365,#27366,#27367,#27368,#27369,#27370,#27371,#27372,#27373,#27374,#27375,
#27376,#27377,#27378,#27379,#27380,#27381,#27382,#27383,#27384,#27385,#27386,
#27387,#27388,#27389,#27390,#27391,#27392,#27393),.UNSPECIFIED.,.F.,.F.)
B_SPLINE_CURVE_WITH_KNOTS((6,1,1,1,1,1,1,1,1,1,1,1,1,1,1,1,1,1,1,1,1,1,
1,1,1,1,1,1,1,1,1,1,1,1,1,1,1,1,1,1,1,1,1,1,1,1,1,1,1,1,1,1,1,1,1,1,1,1,
1,1,1,1,1,1,1,6),(0.,0.0153846153846154,0.0307692307692308,0.0461538461538462,
0.0615384615384615,0.0769230769230769,0.0923076923076923,0.107692307692308,
0.123076923076923,0.138461538461538,0.153846153846154,0.169230769230769,
0.184615384615385,0.2,0.215384615384615,0.230769230769231,0.246153846153846,
0.261538461538462,0.276923076923077,0.292307692307692,0.307692307692308,
0.323076923076923,0.338461538461538,0.353846153846154,0.369230769230769,
0.384615384615385,0.4,0.415384615384615,0.430769230769231,0.446153846153846,
0.461538461538462,0.476923076923077,0.492307692307692,0.507692307692308,
0.523076923076923,0.538461538461538,0.553846153846154,0.569230769230769,
0.584615384615384,0.6,0.615384615384615,0.63076923076923,0.646153846153846,
0.661538461538461,0.676923076923076,0.692307692307692,0.707692307692307,
0.723076923076922,0.738461538461538,0.753846153846153,0.769230769230768,
0.784615384615384,0.799999999999999,0.815384615384614,0.83076923076923,
0.846153846153845,0.86153846153846,0.876923076923076,0.892307692307691,
0.907692307692306,0.923076923076922,0.938461538461537,0.953846153846152,
0.969230769230768,0.984615384615383,1.),.UNSPECIFIED.)
CURVE()
GEOMETRIC_REPRESENTATION_ITEM()
RATIONAL_B_SPLINE_CURVE((1.,1.,1.,1.,1.,1.,1.,1.,1.,1.,1.,1.,1.,1.,1.,1.,
1.,1.,1.,1.,1.,1.,1.,1.,1.,1.,1.,1.,1.,1.,1.,1.,1.,1.,1.,1.,1.,1.,1.,1.,
1.,1.,1.,1.,1.,1.,1.,1.,1.,1.,1.,1.,1.,1.,1.,1.,1.,1.,1.,1.,1.,1.,1.,1.,
1.,1.,1.,1.,1.,1.))
REPRESENTATION_ITEM('')
);
#194=(
BOUNDED_CURVE()
B_SPLINE_CURVE(5,(#27397,#27398,#27399,#27400,#27401,#27402,#27403,#27404,
#27405,#27406,#27407,#27408,#27409,#27410,#27411,#27412,#27413,#27414,#27415,
#27416,#27417,#27418,#27419,#27420,#27421,#27422,#27423,#27424,#27425,#27426,
#27427,#27428,#27429,#27430,#27431,#27432,#27433,#27434,#27435,#27436,#27437,
#27438,#27439,#27440,#27441,#27442,#27443,#27444,#27445,#27446,#27447,#27448,
#27449,#27450,#27451,#27452,#27453,#27454,#27455,#27456,#27457,#27458,#27459,
#27460,#27461,#27462,#27463,#27464,#27465,#27466),.UNSPECIFIED.,.F.,.F.)
B_SPLINE_CURVE_WITH_KNOTS((6,1,1,1,1,1,1,1,1,1,1,1,1,1,1,1,1,1,1,1,1,1,
1,1,1,1,1,1,1,1,1,1,1,1,1,1,1,1,1,1,1,1,1,1,1,1,1,1,1,1,1,1,1,1,1,1,1,1,
1,1,1,1,1,1,1,6),(0.,0.0153846153846154,0.0307692307692308,0.0461538461538462,
0.0615384615384615,0.0769230769230769,0.0923076923076923,0.107692307692308,
0.123076923076923,0.138461538461538,0.153846153846154,0.169230769230769,
0.184615384615385,0.2,0.215384615384615,0.230769230769231,0.246153846153846,
0.261538461538462,0.276923076923077,0.292307692307692,0.307692307692308,
0.323076923076923,0.338461538461538,0.353846153846154,0.369230769230769,
0.384615384615385,0.4,0.415384615384615,0.430769230769231,0.446153846153846,
0.461538461538462,0.476923076923077,0.492307692307692,0.507692307692308,
0.523076923076923,0.538461538461538,0.553846153846154,0.569230769230769,
0.584615384615384,0.6,0.615384615384615,0.63076923076923,0.646153846153846,
0.661538461538461,0.676923076923076,0.692307692307692,0.707692307692307,
0.723076923076922,0.738461538461538,0.753846153846153,0.769230769230768,
0.784615384615384,0.799999999999999,0.815384615384614,0.83076923076923,
0.846153846153845,0.86153846153846,0.876923076923076,0.892307692307691,
0.907692307692306,0.923076923076922,0.938461538461537,0.953846153846152,
0.969230769230768,0.984615384615383,1.),.UNSPECIFIED.)
CURVE()
GEOMETRIC_REPRESENTATION_ITEM()
RATIONAL_B_SPLINE_CURVE((1.,1.,1.,1.,1.,1.,1.,1.,1.,1.,1.,1.,1.,1.,1.,1.,
1.,1.,1.,1.,1.,1.,1.,1.,1.,1.,1.,1.,1.,1.,1.,1.,1.,1.,1.,1.,1.,1.,1.,1.,
1.,1.,1.,1.,1.,1.,1.,1.,1.,1.,1.,1.,1.,1.,1.,1.,1.,1.,1.,1.,1.,1.,1.,1.,
1.,1.,1.,1.,1.,1.))
REPRESENTATION_ITEM('')
);
#195=(
BOUNDED_CURVE()
B_SPLINE_CURVE(5,(#27470,#27471,#27472,#27473,#27474,#27475,#27476,#27477,
#27478,#27479,#27480,#27481,#27482,#27483,#27484,#27485,#27486,#27487,#27488,
#27489,#27490,#27491,#27492,#27493,#27494,#27495,#27496,#27497,#27498,#27499,
#27500,#27501,#27502,#27503,#27504,#27505,#27506,#27507,#27508,#27509,#27510,
#27511,#27512,#27513,#27514,#27515,#27516,#27517,#27518,#27519,#27520,#27521,
#27522,#27523,#27524,#27525,#27526,#27527,#27528,#27529,#27530,#27531,#27532,
#27533,#27534,#27535,#27536,#27537,#27538,#27539),.UNSPECIFIED.,.F.,.F.)
B_SPLINE_CURVE_WITH_KNOTS((6,1,1,1,1,1,1,1,1,1,1,1,1,1,1,1,1,1,1,1,1,1,
1,1,1,1,1,1,1,1,1,1,1,1,1,1,1,1,1,1,1,1,1,1,1,1,1,1,1,1,1,1,1,1,1,1,1,1,
1,1,1,1,1,1,1,6),(0.,0.0153846153846154,0.0307692307692308,0.0461538461538462,
0.0615384615384615,0.0769230769230769,0.0923076923076923,0.107692307692308,
0.123076923076923,0.138461538461538,0.153846153846154,0.169230769230769,
0.184615384615385,0.2,0.215384615384615,0.230769230769231,0.246153846153846,
0.261538461538462,0.276923076923077,0.292307692307692,0.307692307692308,
0.323076923076923,0.338461538461538,0.353846153846154,0.369230769230769,
0.384615384615385,0.4,0.415384615384615,0.430769230769231,0.446153846153846,
0.461538461538462,0.476923076923077,0.492307692307692,0.507692307692308,
0.523076923076923,0.538461538461538,0.553846153846154,0.569230769230769,
0.584615384615384,0.6,0.615384615384615,0.63076923076923,0.646153846153846,
0.661538461538461,0.676923076923076,0.692307692307692,0.707692307692307,
0.723076923076922,0.738461538461538,0.753846153846153,0.769230769230768,
0.784615384615384,0.799999999999999,0.815384615384614,0.83076923076923,
0.846153846153845,0.86153846153846,0.876923076923076,0.892307692307691,
0.907692307692306,0.923076923076922,0.938461538461537,0.953846153846152,
0.969230769230768,0.984615384615383,1.),.UNSPECIFIED.)
CURVE()
GEOMETRIC_REPRESENTATION_ITEM()
RATIONAL_B_SPLINE_CURVE((1.,1.,1.,1.,1.,1.,1.,1.,1.,1.,1.,1.,1.,1.,1.,1.,
1.,1.,1.,1.,1.,1.,1.,1.,1.,1.,1.,1.,1.,1.,1.,1.,1.,1.,1.,1.,1.,1.,1.,1.,
1.,1.,1.,1.,1.,1.,1.,1.,1.,1.,1.,1.,1.,1.,1.,1.,1.,1.,1.,1.,1.,1.,1.,1.,
1.,1.,1.,1.,1.,1.))
REPRESENTATION_ITEM('')
);
#196=(
BOUNDED_CURVE()
B_SPLINE_CURVE(5,(#27543,#27544,#27545,#27546,#27547,#27548,#27549,#27550,
#27551,#27552,#27553,#27554,#27555,#27556,#27557,#27558,#27559,#27560,#27561,
#27562,#27563,#27564,#27565,#27566,#27567,#27568,#27569,#27570,#27571,#27572,
#27573,#27574,#27575,#27576,#27577,#27578,#27579,#27580,#27581,#27582,#27583,
#27584,#27585,#27586,#27587,#27588,#27589,#27590,#27591,#27592,#27593,#27594,
#27595,#27596,#27597,#27598,#27599,#27600,#27601,#27602,#27603,#27604,#27605,
#27606,#27607,#27608,#27609,#27610,#27611,#27612),.UNSPECIFIED.,.F.,.F.)
B_SPLINE_CURVE_WITH_KNOTS((6,1,1,1,1,1,1,1,1,1,1,1,1,1,1,1,1,1,1,1,1,1,
1,1,1,1,1,1,1,1,1,1,1,1,1,1,1,1,1,1,1,1,1,1,1,1,1,1,1,1,1,1,1,1,1,1,1,1,
1,1,1,1,1,1,1,6),(0.,0.0153846153846154,0.0307692307692308,0.0461538461538462,
0.0615384615384615,0.0769230769230769,0.0923076923076923,0.107692307692308,
0.123076923076923,0.138461538461538,0.153846153846154,0.169230769230769,
0.184615384615385,0.2,0.215384615384615,0.230769230769231,0.246153846153846,
0.261538461538462,0.276923076923077,0.292307692307692,0.307692307692308,
0.323076923076923,0.338461538461538,0.353846153846154,0.369230769230769,
0.384615384615385,0.4,0.415384615384615,0.430769230769231,0.446153846153846,
0.461538461538462,0.476923076923077,0.492307692307692,0.507692307692308,
0.523076923076923,0.538461538461538,0.553846153846154,0.569230769230769,
0.584615384615384,0.6,0.615384615384615,0.63076923076923,0.646153846153846,
0.661538461538461,0.676923076923076,0.692307692307692,0.707692307692307,
0.723076923076922,0.738461538461538,0.753846153846153,0.769230769230768,
0.784615384615384,0.799999999999999,0.815384615384614,0.83076923076923,
0.846153846153845,0.86153846153846,0.876923076923076,0.892307692307691,
0.907692307692306,0.923076923076922,0.938461538461537,0.953846153846152,
0.969230769230768,0.984615384615383,1.),.UNSPECIFIED.)
CURVE()
GEOMETRIC_REPRESENTATION_ITEM()
RATIONAL_B_SPLINE_CURVE((1.,1.,1.,1.,1.,1.,1.,1.,1.,1.,1.,1.,1.,1.,1.,1.,
1.,1.,1.,1.,1.,1.,1.,1.,1.,1.,1.,1.,1.,1.,1.,1.,1.,1.,1.,1.,1.,1.,1.,1.,
1.,1.,1.,1.,1.,1.,1.,1.,1.,1.,1.,1.,1.,1.,1.,1.,1.,1.,1.,1.,1.,1.,1.,1.,
1.,1.,1.,1.,1.,1.))
REPRESENTATION_ITEM('')
);
#197=(
BOUNDED_CURVE()
B_SPLINE_CURVE(5,(#27616,#27617,#27618,#27619,#27620,#27621,#27622,#27623,
#27624,#27625,#27626,#27627,#27628,#27629,#27630,#27631,#27632,#27633,#27634,
#27635,#27636,#27637,#27638,#27639,#27640,#27641,#27642,#27643,#27644,#27645,
#27646,#27647,#27648,#27649,#27650,#27651,#27652,#27653,#27654,#27655,#27656,
#27657,#27658,#27659,#27660,#27661,#27662,#27663,#27664,#27665,#27666,#27667,
#27668,#27669,#27670,#27671,#27672,#27673,#27674,#27675,#27676,#27677,#27678,
#27679,#27680,#27681,#27682,#27683,#27684,#27685),.UNSPECIFIED.,.F.,.F.)
B_SPLINE_CURVE_WITH_KNOTS((6,1,1,1,1,1,1,1,1,1,1,1,1,1,1,1,1,1,1,1,1,1,
1,1,1,1,1,1,1,1,1,1,1,1,1,1,1,1,1,1,1,1,1,1,1,1,1,1,1,1,1,1,1,1,1,1,1,1,
1,1,1,1,1,1,1,6),(0.,0.0153846153846154,0.0307692307692308,0.0461538461538462,
0.0615384615384615,0.0769230769230769,0.0923076923076923,0.107692307692308,
0.123076923076923,0.138461538461538,0.153846153846154,0.169230769230769,
0.184615384615385,0.2,0.215384615384615,0.230769230769231,0.246153846153846,
0.261538461538462,0.276923076923077,0.292307692307692,0.307692307692308,
0.323076923076923,0.338461538461538,0.353846153846154,0.369230769230769,
0.384615384615385,0.4,0.415384615384615,0.430769230769231,0.446153846153846,
0.461538461538462,0.476923076923077,0.492307692307692,0.507692307692308,
0.523076923076923,0.538461538461538,0.553846153846154,0.569230769230769,
0.584615384615384,0.6,0.615384615384615,0.63076923076923,0.646153846153846,
0.661538461538461,0.676923076923076,0.692307692307692,0.707692307692307,
0.723076923076922,0.738461538461538,0.753846153846153,0.769230769230768,
0.784615384615384,0.799999999999999,0.815384615384614,0.83076923076923,
0.846153846153845,0.86153846153846,0.876923076923076,0.892307692307691,
0.907692307692306,0.923076923076922,0.938461538461537,0.953846153846152,
0.969230769230768,0.984615384615383,1.),.UNSPECIFIED.)
CURVE()
GEOMETRIC_REPRESENTATION_ITEM()
RATIONAL_B_SPLINE_CURVE((1.,1.,1.,1.,1.,1.,1.,1.,1.,1.,1.,1.,1.,1.,1.,1.,
1.,1.,1.,1.,1.,1.,1.,1.,1.,1.,1.,1.,1.,1.,1.,1.,1.,1.,1.,1.,1.,1.,1.,1.,
1.,1.,1.,1.,1.,1.,1.,1.,1.,1.,1.,1.,1.,1.,1.,1.,1.,1.,1.,1.,1.,1.,1.,1.,
1.,1.,1.,1.,1.,1.))
REPRESENTATION_ITEM('')
);
#198=(
BOUNDED_CURVE()
B_SPLINE_CURVE(5,(#27689,#27690,#27691,#27692,#27693,#27694,#27695,#27696,
#27697,#27698,#27699,#27700,#27701,#27702,#27703,#27704,#27705,#27706,#27707,
#27708,#27709,#27710,#27711,#27712,#27713,#27714,#27715,#27716,#27717,#27718,
#27719,#27720,#27721,#27722,#27723,#27724,#27725,#27726,#27727,#27728,#27729,
#27730,#27731,#27732,#27733,#27734,#27735,#27736,#27737,#27738,#27739,#27740,
#27741,#27742,#27743,#27744,#27745,#27746,#27747,#27748,#27749,#27750,#27751,
#27752,#27753,#27754,#27755,#27756,#27757,#27758),.UNSPECIFIED.,.F.,.F.)
B_SPLINE_CURVE_WITH_KNOTS((6,1,1,1,1,1,1,1,1,1,1,1,1,1,1,1,1,1,1,1,1,1,
1,1,1,1,1,1,1,1,1,1,1,1,1,1,1,1,1,1,1,1,1,1,1,1,1,1,1,1,1,1,1,1,1,1,1,1,
1,1,1,1,1,1,1,6),(0.,0.0153846153846154,0.0307692307692308,0.0461538461538462,
0.0615384615384615,0.0769230769230769,0.0923076923076923,0.107692307692308,
0.123076923076923,0.138461538461538,0.153846153846154,0.169230769230769,
0.184615384615385,0.2,0.215384615384615,0.230769230769231,0.246153846153846,
0.261538461538462,0.276923076923077,0.292307692307692,0.307692307692308,
0.323076923076923,0.338461538461538,0.353846153846154,0.369230769230769,
0.384615384615385,0.4,0.415384615384615,0.430769230769231,0.446153846153846,
0.461538461538462,0.476923076923077,0.492307692307692,0.507692307692308,
0.523076923076923,0.538461538461538,0.553846153846154,0.569230769230769,
0.584615384615384,0.6,0.615384615384615,0.63076923076923,0.646153846153846,
0.661538461538461,0.676923076923076,0.692307692307692,0.707692307692307,
0.723076923076922,0.738461538461538,0.753846153846153,0.769230769230768,
0.784615384615384,0.799999999999999,0.815384615384614,0.83076923076923,
0.846153846153845,0.86153846153846,0.876923076923076,0.892307692307691,
0.907692307692306,0.923076923076922,0.938461538461537,0.953846153846152,
0.969230769230768,0.984615384615383,1.),.UNSPECIFIED.)
CURVE()
GEOMETRIC_REPRESENTATION_ITEM()
RATIONAL_B_SPLINE_CURVE((1.,1.,1.,1.,1.,1.,1.,1.,1.,1.,1.,1.,1.,1.,1.,1.,
1.,1.,1.,1.,1.,1.,1.,1.,1.,1.,1.,1.,1.,1.,1.,1.,1.,1.,1.,1.,1.,1.,1.,1.,
1.,1.,1.,1.,1.,1.,1.,1.,1.,1.,1.,1.,1.,1.,1.,1.,1.,1.,1.,1.,1.,1.,1.,1.,
1.,1.,1.,1.,1.,1.))
REPRESENTATION_ITEM('')
);
#199=(
BOUNDED_CURVE()
B_SPLINE_CURVE(5,(#27762,#27763,#27764,#27765,#27766,#27767,#27768,#27769,
#27770,#27771,#27772,#27773,#27774,#27775,#27776,#27777,#27778,#27779,#27780,
#27781,#27782,#27783,#27784,#27785,#27786,#27787,#27788,#27789,#27790,#27791,
#27792,#27793,#27794,#27795,#27796,#27797,#27798,#27799,#27800,#27801,#27802,
#27803,#27804,#27805,#27806,#27807,#27808,#27809,#27810,#27811,#27812,#27813,
#27814,#27815,#27816,#27817,#27818,#27819,#27820,#27821,#27822,#27823,#27824,
#27825,#27826,#27827,#27828,#27829,#27830,#27831),.UNSPECIFIED.,.F.,.F.)
B_SPLINE_CURVE_WITH_KNOTS((6,1,1,1,1,1,1,1,1,1,1,1,1,1,1,1,1,1,1,1,1,1,
1,1,1,1,1,1,1,1,1,1,1,1,1,1,1,1,1,1,1,1,1,1,1,1,1,1,1,1,1,1,1,1,1,1,1,1,
1,1,1,1,1,1,1,6),(0.,0.0153846153846154,0.0307692307692308,0.0461538461538462,
0.0615384615384615,0.0769230769230769,0.0923076923076923,0.107692307692308,
0.123076923076923,0.138461538461538,0.153846153846154,0.169230769230769,
0.184615384615385,0.2,0.215384615384615,0.230769230769231,0.246153846153846,
0.261538461538462,0.276923076923077,0.292307692307692,0.307692307692308,
0.323076923076923,0.338461538461538,0.353846153846154,0.369230769230769,
0.384615384615385,0.4,0.415384615384615,0.430769230769231,0.446153846153846,
0.461538461538462,0.476923076923077,0.492307692307692,0.507692307692308,
0.523076923076923,0.538461538461538,0.553846153846154,0.569230769230769,
0.584615384615384,0.6,0.615384615384615,0.63076923076923,0.646153846153846,
0.661538461538461,0.676923076923076,0.692307692307692,0.707692307692307,
0.723076923076922,0.738461538461538,0.753846153846153,0.769230769230768,
0.784615384615384,0.799999999999999,0.815384615384614,0.83076923076923,
0.846153846153845,0.86153846153846,0.876923076923076,0.892307692307691,
0.907692307692306,0.923076923076922,0.938461538461537,0.953846153846152,
0.969230769230768,0.984615384615383,1.),.UNSPECIFIED.)
CURVE()
GEOMETRIC_REPRESENTATION_ITEM()
RATIONAL_B_SPLINE_CURVE((1.,1.,1.,1.,1.,1.,1.,1.,1.,1.,1.,1.,1.,1.,1.,1.,
1.,1.,1.,1.,1.,1.,1.,1.,1.,1.,1.,1.,1.,1.,1.,1.,1.,1.,1.,1.,1.,1.,1.,1.,
1.,1.,1.,1.,1.,1.,1.,1.,1.,1.,1.,1.,1.,1.,1.,1.,1.,1.,1.,1.,1.,1.,1.,1.,
1.,1.,1.,1.,1.,1.))
REPRESENTATION_ITEM('')
);
#200=(
BOUNDED_CURVE()
B_SPLINE_CURVE(5,(#27835,#27836,#27837,#27838,#27839,#27840,#27841,#27842,
#27843,#27844,#27845,#27846,#27847,#27848,#27849,#27850,#27851,#27852,#27853,
#27854,#27855,#27856,#27857,#27858,#27859,#27860,#27861,#27862,#27863,#27864,
#27865,#27866,#27867,#27868,#27869,#27870,#27871,#27872,#27873,#27874,#27875,
#27876,#27877,#27878,#27879,#27880,#27881,#27882,#27883,#27884,#27885,#27886,
#27887,#27888,#27889,#27890,#27891,#27892,#27893,#27894,#27895,#27896,#27897,
#27898,#27899,#27900,#27901,#27902,#27903,#27904),.UNSPECIFIED.,.F.,.F.)
B_SPLINE_CURVE_WITH_KNOTS((6,1,1,1,1,1,1,1,1,1,1,1,1,1,1,1,1,1,1,1,1,1,
1,1,1,1,1,1,1,1,1,1,1,1,1,1,1,1,1,1,1,1,1,1,1,1,1,1,1,1,1,1,1,1,1,1,1,1,
1,1,1,1,1,1,1,6),(0.,0.0153846153846154,0.0307692307692308,0.0461538461538462,
0.0615384615384615,0.0769230769230769,0.0923076923076923,0.107692307692308,
0.123076923076923,0.138461538461538,0.153846153846154,0.169230769230769,
0.184615384615385,0.2,0.215384615384615,0.230769230769231,0.246153846153846,
0.261538461538462,0.276923076923077,0.292307692307692,0.307692307692308,
0.323076923076923,0.338461538461538,0.353846153846154,0.369230769230769,
0.384615384615385,0.4,0.415384615384615,0.430769230769231,0.446153846153846,
0.461538461538462,0.476923076923077,0.492307692307692,0.507692307692308,
0.523076923076923,0.538461538461538,0.553846153846154,0.569230769230769,
0.584615384615384,0.6,0.615384615384615,0.63076923076923,0.646153846153846,
0.661538461538461,0.676923076923076,0.692307692307692,0.707692307692307,
0.723076923076922,0.738461538461538,0.753846153846153,0.769230769230768,
0.784615384615384,0.799999999999999,0.815384615384614,0.83076923076923,
0.846153846153845,0.86153846153846,0.876923076923076,0.892307692307691,
0.907692307692306,0.923076923076922,0.938461538461537,0.953846153846152,
0.969230769230768,0.984615384615383,1.),.UNSPECIFIED.)
CURVE()
GEOMETRIC_REPRESENTATION_ITEM()
RATIONAL_B_SPLINE_CURVE((1.,1.,1.,1.,1.,1.,1.,1.,1.,1.,1.,1.,1.,1.,1.,1.,
1.,1.,1.,1.,1.,1.,1.,1.,1.,1.,1.,1.,1.,1.,1.,1.,1.,1.,1.,1.,1.,1.,1.,1.,
1.,1.,1.,1.,1.,1.,1.,1.,1.,1.,1.,1.,1.,1.,1.,1.,1.,1.,1.,1.,1.,1.,1.,1.,
1.,1.,1.,1.,1.,1.))
REPRESENTATION_ITEM('')
);
#201=(
BOUNDED_CURVE()
B_SPLINE_CURVE(5,(#27908,#27909,#27910,#27911,#27912,#27913,#27914,#27915,
#27916,#27917,#27918,#27919,#27920,#27921,#27922,#27923,#27924,#27925,#27926,
#27927,#27928,#27929,#27930,#27931,#27932,#27933,#27934,#27935,#27936,#27937,
#27938,#27939,#27940,#27941,#27942,#27943,#27944,#27945,#27946,#27947,#27948,
#27949,#27950,#27951,#27952,#27953,#27954,#27955,#27956,#27957,#27958,#27959,
#27960,#27961,#27962,#27963,#27964,#27965,#27966,#27967,#27968,#27969,#27970,
#27971,#27972,#27973,#27974,#27975,#27976,#27977),.UNSPECIFIED.,.F.,.F.)
B_SPLINE_CURVE_WITH_KNOTS((6,1,1,1,1,1,1,1,1,1,1,1,1,1,1,1,1,1,1,1,1,1,
1,1,1,1,1,1,1,1,1,1,1,1,1,1,1,1,1,1,1,1,1,1,1,1,1,1,1,1,1,1,1,1,1,1,1,1,
1,1,1,1,1,1,1,6),(0.,0.0153846153846154,0.0307692307692308,0.0461538461538462,
0.0615384615384615,0.0769230769230769,0.0923076923076923,0.107692307692308,
0.123076923076923,0.138461538461538,0.153846153846154,0.169230769230769,
0.184615384615385,0.2,0.215384615384615,0.230769230769231,0.246153846153846,
0.261538461538462,0.276923076923077,0.292307692307692,0.307692307692308,
0.323076923076923,0.338461538461538,0.353846153846154,0.369230769230769,
0.384615384615385,0.4,0.415384615384615,0.430769230769231,0.446153846153846,
0.461538461538462,0.476923076923077,0.492307692307692,0.507692307692308,
0.523076923076923,0.538461538461538,0.553846153846154,0.569230769230769,
0.584615384615384,0.6,0.615384615384615,0.63076923076923,0.646153846153846,
0.661538461538461,0.676923076923076,0.692307692307692,0.707692307692307,
0.723076923076922,0.738461538461538,0.753846153846153,0.769230769230768,
0.784615384615384,0.799999999999999,0.815384615384614,0.83076923076923,
0.846153846153845,0.86153846153846,0.876923076923076,0.892307692307691,
0.907692307692306,0.923076923076922,0.938461538461537,0.953846153846152,
0.969230769230768,0.984615384615383,1.),.UNSPECIFIED.)
CURVE()
GEOMETRIC_REPRESENTATION_ITEM()
RATIONAL_B_SPLINE_CURVE((1.,1.,1.,1.,1.,1.,1.,1.,1.,1.,1.,1.,1.,1.,1.,1.,
1.,1.,1.,1.,1.,1.,1.,1.,1.,1.,1.,1.,1.,1.,1.,1.,1.,1.,1.,1.,1.,1.,1.,1.,
1.,1.,1.,1.,1.,1.,1.,1.,1.,1.,1.,1.,1.,1.,1.,1.,1.,1.,1.,1.,1.,1.,1.,1.,
1.,1.,1.,1.,1.,1.))
REPRESENTATION_ITEM('')
);
#202=(
BOUNDED_CURVE()
B_SPLINE_CURVE(5,(#27981,#27982,#27983,#27984,#27985,#27986,#27987,#27988,
#27989,#27990,#27991,#27992,#27993,#27994,#27995,#27996,#27997,#27998,#27999,
#28000,#28001,#28002,#28003,#28004,#28005,#28006,#28007,#28008,#28009,#28010,
#28011,#28012,#28013,#28014,#28015,#28016,#28017,#28018,#28019,#28020,#28021,
#28022,#28023,#28024,#28025,#28026,#28027,#28028,#28029,#28030,#28031,#28032,
#28033,#28034,#28035,#28036,#28037,#28038,#28039,#28040,#28041,#28042,#28043,
#28044,#28045,#28046,#28047,#28048,#28049,#28050),.UNSPECIFIED.,.F.,.F.)
B_SPLINE_CURVE_WITH_KNOTS((6,1,1,1,1,1,1,1,1,1,1,1,1,1,1,1,1,1,1,1,1,1,
1,1,1,1,1,1,1,1,1,1,1,1,1,1,1,1,1,1,1,1,1,1,1,1,1,1,1,1,1,1,1,1,1,1,1,1,
1,1,1,1,1,1,1,6),(0.,0.0153846153846154,0.0307692307692308,0.0461538461538462,
0.0615384615384615,0.0769230769230769,0.0923076923076923,0.107692307692308,
0.123076923076923,0.138461538461538,0.153846153846154,0.169230769230769,
0.184615384615385,0.2,0.215384615384615,0.230769230769231,0.246153846153846,
0.261538461538462,0.276923076923077,0.292307692307692,0.307692307692308,
0.323076923076923,0.338461538461538,0.353846153846154,0.369230769230769,
0.384615384615385,0.4,0.415384615384615,0.430769230769231,0.446153846153846,
0.461538461538462,0.476923076923077,0.492307692307692,0.507692307692308,
0.523076923076923,0.538461538461538,0.553846153846154,0.569230769230769,
0.584615384615384,0.6,0.615384615384615,0.63076923076923,0.646153846153846,
0.661538461538461,0.676923076923076,0.692307692307692,0.707692307692307,
0.723076923076922,0.738461538461538,0.753846153846153,0.769230769230768,
0.784615384615384,0.799999999999999,0.815384615384614,0.83076923076923,
0.846153846153845,0.86153846153846,0.876923076923076,0.892307692307691,
0.907692307692306,0.923076923076922,0.938461538461537,0.953846153846152,
0.969230769230768,0.984615384615383,1.),.UNSPECIFIED.)
CURVE()
GEOMETRIC_REPRESENTATION_ITEM()
RATIONAL_B_SPLINE_CURVE((1.,1.,1.,1.,1.,1.,1.,1.,1.,1.,1.,1.,1.,1.,1.,1.,
1.,1.,1.,1.,1.,1.,1.,1.,1.,1.,1.,1.,1.,1.,1.,1.,1.,1.,1.,1.,1.,1.,1.,1.,
1.,1.,1.,1.,1.,1.,1.,1.,1.,1.,1.,1.,1.,1.,1.,1.,1.,1.,1.,1.,1.,1.,1.,1.,
1.,1.,1.,1.,1.,1.))
REPRESENTATION_ITEM('')
);
#203=(
BOUNDED_CURVE()
B_SPLINE_CURVE(5,(#28054,#28055,#28056,#28057,#28058,#28059,#28060,#28061,
#28062,#28063,#28064,#28065,#28066,#28067,#28068,#28069,#28070,#28071,#28072,
#28073,#28074,#28075,#28076,#28077,#28078,#28079,#28080,#28081,#28082,#28083,
#28084,#28085,#28086,#28087,#28088,#28089,#28090,#28091,#28092,#28093,#28094,
#28095,#28096,#28097,#28098,#28099,#28100,#28101,#28102,#28103,#28104,#28105,
#28106,#28107,#28108,#28109,#28110,#28111,#28112,#28113,#28114,#28115,#28116,
#28117,#28118,#28119,#28120,#28121,#28122,#28123),.UNSPECIFIED.,.F.,.F.)
B_SPLINE_CURVE_WITH_KNOTS((6,1,1,1,1,1,1,1,1,1,1,1,1,1,1,1,1,1,1,1,1,1,
1,1,1,1,1,1,1,1,1,1,1,1,1,1,1,1,1,1,1,1,1,1,1,1,1,1,1,1,1,1,1,1,1,1,1,1,
1,1,1,1,1,1,1,6),(0.,0.0153846153846154,0.0307692307692308,0.0461538461538462,
0.0615384615384615,0.0769230769230769,0.0923076923076923,0.107692307692308,
0.123076923076923,0.138461538461538,0.153846153846154,0.169230769230769,
0.184615384615385,0.2,0.215384615384615,0.230769230769231,0.246153846153846,
0.261538461538462,0.276923076923077,0.292307692307692,0.307692307692308,
0.323076923076923,0.338461538461538,0.353846153846154,0.369230769230769,
0.384615384615385,0.4,0.415384615384615,0.430769230769231,0.446153846153846,
0.461538461538462,0.476923076923077,0.492307692307692,0.507692307692308,
0.523076923076923,0.538461538461538,0.553846153846154,0.569230769230769,
0.584615384615384,0.6,0.615384615384615,0.63076923076923,0.646153846153846,
0.661538461538461,0.676923076923076,0.692307692307692,0.707692307692307,
0.723076923076922,0.738461538461538,0.753846153846153,0.769230769230768,
0.784615384615384,0.799999999999999,0.815384615384614,0.83076923076923,
0.846153846153845,0.86153846153846,0.876923076923076,0.892307692307691,
0.907692307692306,0.923076923076922,0.938461538461537,0.953846153846152,
0.969230769230768,0.984615384615383,1.),.UNSPECIFIED.)
CURVE()
GEOMETRIC_REPRESENTATION_ITEM()
RATIONAL_B_SPLINE_CURVE((1.,1.,1.,1.,1.,1.,1.,1.,1.,1.,1.,1.,1.,1.,1.,1.,
1.,1.,1.,1.,1.,1.,1.,1.,1.,1.,1.,1.,1.,1.,1.,1.,1.,1.,1.,1.,1.,1.,1.,1.,
1.,1.,1.,1.,1.,1.,1.,1.,1.,1.,1.,1.,1.,1.,1.,1.,1.,1.,1.,1.,1.,1.,1.,1.,
1.,1.,1.,1.,1.,1.))
REPRESENTATION_ITEM('')
);
#204=(
BOUNDED_CURVE()
B_SPLINE_CURVE(5,(#28127,#28128,#28129,#28130,#28131,#28132,#28133,#28134,
#28135,#28136,#28137,#28138,#28139,#28140,#28141,#28142,#28143,#28144,#28145,
#28146,#28147,#28148,#28149,#28150,#28151,#28152,#28153,#28154,#28155,#28156,
#28157,#28158,#28159,#28160,#28161,#28162,#28163,#28164,#28165,#28166,#28167,
#28168,#28169,#28170,#28171,#28172,#28173,#28174,#28175,#28176,#28177,#28178,
#28179,#28180,#28181,#28182,#28183,#28184,#28185,#28186,#28187,#28188,#28189,
#28190,#28191,#28192,#28193,#28194,#28195,#28196),.UNSPECIFIED.,.F.,.F.)
B_SPLINE_CURVE_WITH_KNOTS((6,1,1,1,1,1,1,1,1,1,1,1,1,1,1,1,1,1,1,1,1,1,
1,1,1,1,1,1,1,1,1,1,1,1,1,1,1,1,1,1,1,1,1,1,1,1,1,1,1,1,1,1,1,1,1,1,1,1,
1,1,1,1,1,1,1,6),(0.,0.0153846153846154,0.0307692307692308,0.0461538461538462,
0.0615384615384615,0.0769230769230769,0.0923076923076923,0.107692307692308,
0.123076923076923,0.138461538461538,0.153846153846154,0.169230769230769,
0.184615384615385,0.2,0.215384615384615,0.230769230769231,0.246153846153846,
0.261538461538462,0.276923076923077,0.292307692307692,0.307692307692308,
0.323076923076923,0.338461538461538,0.353846153846154,0.369230769230769,
0.384615384615385,0.4,0.415384615384615,0.430769230769231,0.446153846153846,
0.461538461538462,0.476923076923077,0.492307692307692,0.507692307692308,
0.523076923076923,0.538461538461538,0.553846153846154,0.569230769230769,
0.584615384615384,0.6,0.615384615384615,0.63076923076923,0.646153846153846,
0.661538461538461,0.676923076923076,0.692307692307692,0.707692307692307,
0.723076923076922,0.738461538461538,0.753846153846153,0.769230769230768,
0.784615384615384,0.799999999999999,0.815384615384614,0.83076923076923,
0.846153846153845,0.86153846153846,0.876923076923076,0.892307692307691,
0.907692307692306,0.923076923076922,0.938461538461537,0.953846153846152,
0.969230769230768,0.984615384615383,1.),.UNSPECIFIED.)
CURVE()
GEOMETRIC_REPRESENTATION_ITEM()
RATIONAL_B_SPLINE_CURVE((1.,1.,1.,1.,1.,1.,1.,1.,1.,1.,1.,1.,1.,1.,1.,1.,
1.,1.,1.,1.,1.,1.,1.,1.,1.,1.,1.,1.,1.,1.,1.,1.,1.,1.,1.,1.,1.,1.,1.,1.,
1.,1.,1.,1.,1.,1.,1.,1.,1.,1.,1.,1.,1.,1.,1.,1.,1.,1.,1.,1.,1.,1.,1.,1.,
1.,1.,1.,1.,1.,1.))
REPRESENTATION_ITEM('')
);
#205=(
BOUNDED_CURVE()
B_SPLINE_CURVE(5,(#28200,#28201,#28202,#28203,#28204,#28205,#28206,#28207,
#28208,#28209,#28210,#28211,#28212,#28213,#28214,#28215,#28216,#28217,#28218,
#28219,#28220,#28221,#28222,#28223,#28224,#28225,#28226,#28227,#28228,#28229,
#28230,#28231,#28232,#28233,#28234,#28235,#28236,#28237,#28238,#28239,#28240,
#28241,#28242,#28243,#28244,#28245,#28246,#28247,#28248,#28249,#28250,#28251,
#28252,#28253,#28254,#28255,#28256,#28257,#28258,#28259,#28260,#28261,#28262,
#28263,#28264,#28265,#28266,#28267,#28268,#28269),.UNSPECIFIED.,.F.,.F.)
B_SPLINE_CURVE_WITH_KNOTS((6,1,1,1,1,1,1,1,1,1,1,1,1,1,1,1,1,1,1,1,1,1,
1,1,1,1,1,1,1,1,1,1,1,1,1,1,1,1,1,1,1,1,1,1,1,1,1,1,1,1,1,1,1,1,1,1,1,1,
1,1,1,1,1,1,1,6),(0.,0.0153846153846154,0.0307692307692308,0.0461538461538462,
0.0615384615384615,0.0769230769230769,0.0923076923076923,0.107692307692308,
0.123076923076923,0.138461538461538,0.153846153846154,0.169230769230769,
0.184615384615385,0.2,0.215384615384615,0.230769230769231,0.246153846153846,
0.261538461538462,0.276923076923077,0.292307692307692,0.307692307692308,
0.323076923076923,0.338461538461538,0.353846153846154,0.369230769230769,
0.384615384615385,0.4,0.415384615384615,0.430769230769231,0.446153846153846,
0.461538461538462,0.476923076923077,0.492307692307692,0.507692307692308,
0.523076923076923,0.538461538461538,0.553846153846154,0.569230769230769,
0.584615384615384,0.6,0.615384615384615,0.63076923076923,0.646153846153846,
0.661538461538461,0.676923076923076,0.692307692307692,0.707692307692307,
0.723076923076922,0.738461538461538,0.753846153846153,0.769230769230768,
0.784615384615384,0.799999999999999,0.815384615384614,0.83076923076923,
0.846153846153845,0.86153846153846,0.876923076923076,0.892307692307691,
0.907692307692306,0.923076923076922,0.938461538461537,0.953846153846152,
0.969230769230768,0.984615384615383,1.),.UNSPECIFIED.)
CURVE()
GEOMETRIC_REPRESENTATION_ITEM()
RATIONAL_B_SPLINE_CURVE((1.,1.,1.,1.,1.,1.,1.,1.,1.,1.,1.,1.,1.,1.,1.,1.,
1.,1.,1.,1.,1.,1.,1.,1.,1.,1.,1.,1.,1.,1.,1.,1.,1.,1.,1.,1.,1.,1.,1.,1.,
1.,1.,1.,1.,1.,1.,1.,1.,1.,1.,1.,1.,1.,1.,1.,1.,1.,1.,1.,1.,1.,1.,1.,1.,
1.,1.,1.,1.,1.,1.))
REPRESENTATION_ITEM('')
);
#206=(
BOUNDED_CURVE()
B_SPLINE_CURVE(5,(#28273,#28274,#28275,#28276,#28277,#28278,#28279,#28280,
#28281,#28282,#28283,#28284,#28285,#28286,#28287,#28288,#28289,#28290,#28291,
#28292,#28293,#28294,#28295,#28296,#28297,#28298,#28299,#28300,#28301,#28302,
#28303,#28304,#28305,#28306,#28307,#28308,#28309,#28310,#28311,#28312,#28313,
#28314,#28315,#28316,#28317,#28318,#28319,#28320,#28321,#28322,#28323,#28324,
#28325,#28326,#28327,#28328,#28329,#28330,#28331,#28332,#28333,#28334,#28335,
#28336,#28337,#28338,#28339,#28340,#28341,#28342),.UNSPECIFIED.,.F.,.F.)
B_SPLINE_CURVE_WITH_KNOTS((6,1,1,1,1,1,1,1,1,1,1,1,1,1,1,1,1,1,1,1,1,1,
1,1,1,1,1,1,1,1,1,1,1,1,1,1,1,1,1,1,1,1,1,1,1,1,1,1,1,1,1,1,1,1,1,1,1,1,
1,1,1,1,1,1,1,6),(0.,0.0153846153846154,0.0307692307692308,0.0461538461538462,
0.0615384615384615,0.0769230769230769,0.0923076923076923,0.107692307692308,
0.123076923076923,0.138461538461538,0.153846153846154,0.169230769230769,
0.184615384615385,0.2,0.215384615384615,0.230769230769231,0.246153846153846,
0.261538461538462,0.276923076923077,0.292307692307692,0.307692307692308,
0.323076923076923,0.338461538461538,0.353846153846154,0.369230769230769,
0.384615384615385,0.4,0.415384615384615,0.430769230769231,0.446153846153846,
0.461538461538462,0.476923076923077,0.492307692307692,0.507692307692308,
0.523076923076923,0.538461538461538,0.553846153846154,0.569230769230769,
0.584615384615384,0.6,0.615384615384615,0.63076923076923,0.646153846153846,
0.661538461538461,0.676923076923076,0.692307692307692,0.707692307692307,
0.723076923076922,0.738461538461538,0.753846153846153,0.769230769230768,
0.784615384615384,0.799999999999999,0.815384615384614,0.83076923076923,
0.846153846153845,0.86153846153846,0.876923076923076,0.892307692307691,
0.907692307692306,0.923076923076922,0.938461538461537,0.953846153846152,
0.969230769230768,0.984615384615383,1.),.UNSPECIFIED.)
CURVE()
GEOMETRIC_REPRESENTATION_ITEM()
RATIONAL_B_SPLINE_CURVE((1.,1.,1.,1.,1.,1.,1.,1.,1.,1.,1.,1.,1.,1.,1.,1.,
1.,1.,1.,1.,1.,1.,1.,1.,1.,1.,1.,1.,1.,1.,1.,1.,1.,1.,1.,1.,1.,1.,1.,1.,
1.,1.,1.,1.,1.,1.,1.,1.,1.,1.,1.,1.,1.,1.,1.,1.,1.,1.,1.,1.,1.,1.,1.,1.,
1.,1.,1.,1.,1.,1.))
REPRESENTATION_ITEM('')
);
#207=(
BOUNDED_CURVE()
B_SPLINE_CURVE(5,(#28346,#28347,#28348,#28349,#28350,#28351,#28352,#28353,
#28354,#28355,#28356,#28357,#28358,#28359,#28360,#28361,#28362,#28363,#28364,
#28365,#28366,#28367,#28368,#28369,#28370,#28371,#28372,#28373,#28374,#28375,
#28376,#28377,#28378,#28379,#28380,#28381,#28382,#28383,#28384,#28385,#28386,
#28387,#28388,#28389,#28390,#28391,#28392,#28393,#28394,#28395,#28396,#28397,
#28398,#28399,#28400,#28401,#28402,#28403,#28404,#28405,#28406,#28407,#28408,
#28409,#28410,#28411,#28412,#28413,#28414,#28415),.UNSPECIFIED.,.F.,.F.)
B_SPLINE_CURVE_WITH_KNOTS((6,1,1,1,1,1,1,1,1,1,1,1,1,1,1,1,1,1,1,1,1,1,
1,1,1,1,1,1,1,1,1,1,1,1,1,1,1,1,1,1,1,1,1,1,1,1,1,1,1,1,1,1,1,1,1,1,1,1,
1,1,1,1,1,1,1,6),(0.,0.0153846153846154,0.0307692307692308,0.0461538461538462,
0.0615384615384615,0.0769230769230769,0.0923076923076923,0.107692307692308,
0.123076923076923,0.138461538461538,0.153846153846154,0.169230769230769,
0.184615384615385,0.2,0.215384615384615,0.230769230769231,0.246153846153846,
0.261538461538462,0.276923076923077,0.292307692307692,0.307692307692308,
0.323076923076923,0.338461538461538,0.353846153846154,0.369230769230769,
0.384615384615385,0.4,0.415384615384615,0.430769230769231,0.446153846153846,
0.461538461538462,0.476923076923077,0.492307692307692,0.507692307692308,
0.523076923076923,0.538461538461538,0.553846153846154,0.569230769230769,
0.584615384615384,0.6,0.615384615384615,0.63076923076923,0.646153846153846,
0.661538461538461,0.676923076923076,0.692307692307692,0.707692307692307,
0.723076923076922,0.738461538461538,0.753846153846153,0.769230769230768,
0.784615384615384,0.799999999999999,0.815384615384614,0.83076923076923,
0.846153846153845,0.86153846153846,0.876923076923076,0.892307692307691,
0.907692307692306,0.923076923076922,0.938461538461537,0.953846153846152,
0.969230769230768,0.984615384615383,1.),.UNSPECIFIED.)
CURVE()
GEOMETRIC_REPRESENTATION_ITEM()
RATIONAL_B_SPLINE_CURVE((1.,1.,1.,1.,1.,1.,1.,1.,1.,1.,1.,1.,1.,1.,1.,1.,
1.,1.,1.,1.,1.,1.,1.,1.,1.,1.,1.,1.,1.,1.,1.,1.,1.,1.,1.,1.,1.,1.,1.,1.,
1.,1.,1.,1.,1.,1.,1.,1.,1.,1.,1.,1.,1.,1.,1.,1.,1.,1.,1.,1.,1.,1.,1.,1.,
1.,1.,1.,1.,1.,1.))
REPRESENTATION_ITEM('')
);
#208=(
BOUNDED_CURVE()
B_SPLINE_CURVE(5,(#28419,#28420,#28421,#28422,#28423,#28424,#28425,#28426,
#28427,#28428,#28429,#28430,#28431,#28432,#28433,#28434,#28435,#28436,#28437,
#28438,#28439,#28440,#28441,#28442,#28443,#28444,#28445,#28446,#28447,#28448,
#28449,#28450,#28451,#28452,#28453,#28454,#28455,#28456,#28457,#28458,#28459,
#28460,#28461,#28462,#28463,#28464,#28465,#28466,#28467,#28468,#28469,#28470,
#28471,#28472,#28473,#28474,#28475,#28476,#28477,#28478,#28479,#28480,#28481,
#28482,#28483,#28484,#28485,#28486,#28487,#28488),.UNSPECIFIED.,.F.,.F.)
B_SPLINE_CURVE_WITH_KNOTS((6,1,1,1,1,1,1,1,1,1,1,1,1,1,1,1,1,1,1,1,1,1,
1,1,1,1,1,1,1,1,1,1,1,1,1,1,1,1,1,1,1,1,1,1,1,1,1,1,1,1,1,1,1,1,1,1,1,1,
1,1,1,1,1,1,1,6),(0.,0.0153846153846154,0.0307692307692308,0.0461538461538462,
0.0615384615384615,0.0769230769230769,0.0923076923076923,0.107692307692308,
0.123076923076923,0.138461538461538,0.153846153846154,0.169230769230769,
0.184615384615385,0.2,0.215384615384615,0.230769230769231,0.246153846153846,
0.261538461538462,0.276923076923077,0.292307692307692,0.307692307692308,
0.323076923076923,0.338461538461538,0.353846153846154,0.369230769230769,
0.384615384615385,0.4,0.415384615384615,0.430769230769231,0.446153846153846,
0.461538461538462,0.476923076923077,0.492307692307692,0.507692307692308,
0.523076923076923,0.538461538461538,0.553846153846154,0.569230769230769,
0.584615384615384,0.6,0.615384615384615,0.63076923076923,0.646153846153846,
0.661538461538461,0.676923076923076,0.692307692307692,0.707692307692307,
0.723076923076922,0.738461538461538,0.753846153846153,0.769230769230768,
0.784615384615384,0.799999999999999,0.815384615384614,0.83076923076923,
0.846153846153845,0.86153846153846,0.876923076923076,0.892307692307691,
0.907692307692306,0.923076923076922,0.938461538461537,0.953846153846152,
0.969230769230768,0.984615384615383,1.),.UNSPECIFIED.)
CURVE()
GEOMETRIC_REPRESENTATION_ITEM()
RATIONAL_B_SPLINE_CURVE((1.,1.,1.,1.,1.,1.,1.,1.,1.,1.,1.,1.,1.,1.,1.,1.,
1.,1.,1.,1.,1.,1.,1.,1.,1.,1.,1.,1.,1.,1.,1.,1.,1.,1.,1.,1.,1.,1.,1.,1.,
1.,1.,1.,1.,1.,1.,1.,1.,1.,1.,1.,1.,1.,1.,1.,1.,1.,1.,1.,1.,1.,1.,1.,1.,
1.,1.,1.,1.,1.,1.))
REPRESENTATION_ITEM('')
);
#209=(
BOUNDED_CURVE()
B_SPLINE_CURVE(5,(#28492,#28493,#28494,#28495,#28496,#28497,#28498,#28499,
#28500,#28501,#28502,#28503,#28504,#28505,#28506,#28507,#28508,#28509,#28510,
#28511,#28512,#28513,#28514,#28515,#28516,#28517,#28518,#28519,#28520,#28521,
#28522,#28523,#28524,#28525,#28526,#28527,#28528,#28529,#28530,#28531,#28532,
#28533,#28534,#28535,#28536,#28537,#28538,#28539,#28540,#28541,#28542,#28543,
#28544,#28545,#28546,#28547,#28548,#28549,#28550,#28551,#28552,#28553,#28554,
#28555,#28556,#28557,#28558,#28559,#28560,#28561),.UNSPECIFIED.,.F.,.F.)
B_SPLINE_CURVE_WITH_KNOTS((6,1,1,1,1,1,1,1,1,1,1,1,1,1,1,1,1,1,1,1,1,1,
1,1,1,1,1,1,1,1,1,1,1,1,1,1,1,1,1,1,1,1,1,1,1,1,1,1,1,1,1,1,1,1,1,1,1,1,
1,1,1,1,1,1,1,6),(0.,0.0153846153846154,0.0307692307692308,0.0461538461538462,
0.0615384615384615,0.0769230769230769,0.0923076923076923,0.107692307692308,
0.123076923076923,0.138461538461538,0.153846153846154,0.169230769230769,
0.184615384615385,0.2,0.215384615384615,0.230769230769231,0.246153846153846,
0.261538461538462,0.276923076923077,0.292307692307692,0.307692307692308,
0.323076923076923,0.338461538461538,0.353846153846154,0.369230769230769,
0.384615384615385,0.4,0.415384615384615,0.430769230769231,0.446153846153846,
0.461538461538462,0.476923076923077,0.492307692307692,0.507692307692308,
0.523076923076923,0.538461538461538,0.553846153846154,0.569230769230769,
0.584615384615384,0.6,0.615384615384615,0.63076923076923,0.646153846153846,
0.661538461538461,0.676923076923076,0.692307692307692,0.707692307692307,
0.723076923076922,0.738461538461538,0.753846153846153,0.769230769230768,
0.784615384615384,0.799999999999999,0.815384615384614,0.83076923076923,
0.846153846153845,0.86153846153846,0.876923076923076,0.892307692307691,
0.907692307692306,0.923076923076922,0.938461538461537,0.953846153846152,
0.969230769230768,0.984615384615383,1.),.UNSPECIFIED.)
CURVE()
GEOMETRIC_REPRESENTATION_ITEM()
RATIONAL_B_SPLINE_CURVE((1.,1.,1.,1.,1.,1.,1.,1.,1.,1.,1.,1.,1.,1.,1.,1.,
1.,1.,1.,1.,1.,1.,1.,1.,1.,1.,1.,1.,1.,1.,1.,1.,1.,1.,1.,1.,1.,1.,1.,1.,
1.,1.,1.,1.,1.,1.,1.,1.,1.,1.,1.,1.,1.,1.,1.,1.,1.,1.,1.,1.,1.,1.,1.,1.,
1.,1.,1.,1.,1.,1.))
REPRESENTATION_ITEM('')
);
#210=(
BOUNDED_CURVE()
B_SPLINE_CURVE(5,(#28564,#28565,#28566,#28567,#28568,#28569,#28570,#28571,
#28572,#28573,#28574,#28575,#28576,#28577,#28578,#28579,#28580,#28581,#28582,
#28583,#28584,#28585,#28586,#28587,#28588,#28589,#28590,#28591,#28592,#28593,
#28594,#28595,#28596,#28597,#28598,#28599,#28600,#28601,#28602,#28603,#28604,
#28605,#28606,#28607,#28608,#28609,#28610,#28611,#28612,#28613,#28614,#28615,
#28616,#28617,#28618,#28619,#28620,#28621,#28622,#28623,#28624,#28625,#28626,
#28627,#28628,#28629,#28630,#28631,#28632,#28633),.UNSPECIFIED.,.F.,.F.)
B_SPLINE_CURVE_WITH_KNOTS((6,1,1,1,1,1,1,1,1,1,1,1,1,1,1,1,1,1,1,1,1,1,
1,1,1,1,1,1,1,1,1,1,1,1,1,1,1,1,1,1,1,1,1,1,1,1,1,1,1,1,1,1,1,1,1,1,1,1,
1,1,1,1,1,1,1,6),(0.,0.0153846153846154,0.0307692307692308,0.0461538461538462,
0.0615384615384615,0.0769230769230769,0.0923076923076923,0.107692307692308,
0.123076923076923,0.138461538461538,0.153846153846154,0.169230769230769,
0.184615384615385,0.2,0.215384615384615,0.230769230769231,0.246153846153846,
0.261538461538462,0.276923076923077,0.292307692307692,0.307692307692308,
0.323076923076923,0.338461538461538,0.353846153846154,0.369230769230769,
0.384615384615385,0.4,0.415384615384615,0.430769230769231,0.446153846153846,
0.461538461538462,0.476923076923077,0.492307692307692,0.507692307692308,
0.523076923076923,0.538461538461538,0.553846153846154,0.569230769230769,
0.584615384615384,0.6,0.615384615384615,0.63076923076923,0.646153846153846,
0.661538461538461,0.676923076923076,0.692307692307692,0.707692307692307,
0.723076923076922,0.738461538461538,0.753846153846153,0.769230769230768,
0.784615384615384,0.799999999999999,0.815384615384614,0.83076923076923,
0.846153846153845,0.86153846153846,0.876923076923076,0.892307692307691,
0.907692307692306,0.923076923076922,0.938461538461537,0.953846153846152,
0.969230769230768,0.984615384615383,1.),.UNSPECIFIED.)
CURVE()
GEOMETRIC_REPRESENTATION_ITEM()
RATIONAL_B_SPLINE_CURVE((1.,1.,1.,1.,1.,1.,1.,1.,1.,1.,1.,1.,1.,1.,1.,1.,
1.,1.,1.,1.,1.,1.,1.,1.,1.,1.,1.,1.,1.,1.,1.,1.,1.,1.,1.,1.,1.,1.,1.,1.,
1.,1.,1.,1.,1.,1.,1.,1.,1.,1.,1.,1.,1.,1.,1.,1.,1.,1.,1.,1.,1.,1.,1.,1.,
1.,1.,1.,1.,1.,1.))
REPRESENTATION_ITEM('')
);
#211=(
BOUNDED_CURVE()
B_SPLINE_CURVE(5,(#28787,#28788,#28789,#28790,#28791,#28792,#28793,#28794,
#28795,#28796,#28797,#28798,#28799,#28800,#28801,#28802,#28803,#28804,#28805,
#28806,#28807,#28808,#28809,#28810,#28811,#28812,#28813,#28814,#28815,#28816,
#28817,#28818,#28819,#28820,#28821,#28822,#28823,#28824,#28825,#28826,#28827,
#28828,#28829,#28830,#28831,#28832,#28833,#28834,#28835,#28836,#28837,#28838,
#28839,#28840,#28841,#28842,#28843,#28844,#28845,#28846,#28847,#28848,#28849,
#28850,#28851,#28852,#28853,#28854,#28855,#28856),.UNSPECIFIED.,.F.,.F.)
B_SPLINE_CURVE_WITH_KNOTS((6,1,1,1,1,1,1,1,1,1,1,1,1,1,1,1,1,1,1,1,1,1,
1,1,1,1,1,1,1,1,1,1,1,1,1,1,1,1,1,1,1,1,1,1,1,1,1,1,1,1,1,1,1,1,1,1,1,1,
1,1,1,1,1,1,1,6),(-1.,-0.984615384615383,-0.969230769230768,-0.953846153846152,
-0.938461538461537,-0.923076923076922,-0.907692307692306,-0.892307692307691,
-0.876923076923076,-0.86153846153846,-0.846153846153845,-0.83076923076923,
-0.815384615384614,-0.799999999999999,-0.784615384615384,-0.769230769230768,
-0.753846153846153,-0.738461538461538,-0.723076923076922,-0.707692307692307,
-0.692307692307692,-0.676923076923076,-0.661538461538461,-0.646153846153846,
-0.63076923076923,-0.615384615384615,-0.6,-0.584615384615384,-0.569230769230769,
-0.553846153846154,-0.538461538461538,-0.523076923076923,-0.507692307692308,
-0.492307692307692,-0.476923076923077,-0.461538461538462,-0.446153846153846,
-0.430769230769231,-0.415384615384615,-0.4,-0.384615384615385,-0.369230769230769,
-0.353846153846154,-0.338461538461538,-0.323076923076923,-0.307692307692308,
-0.292307692307692,-0.276923076923077,-0.261538461538462,-0.246153846153846,
-0.230769230769231,-0.215384615384615,-0.2,-0.184615384615385,-0.169230769230769,
-0.153846153846154,-0.138461538461538,-0.123076923076923,-0.107692307692308,
-0.0923076923076923,-0.0769230769230769,-0.0615384615384615,-0.0461538461538462,
-0.0307692307692308,-0.0153846153846154,0.),.UNSPECIFIED.)
CURVE()
GEOMETRIC_REPRESENTATION_ITEM()
RATIONAL_B_SPLINE_CURVE((1.,1.,1.,1.,1.,1.,1.,1.,1.,1.,1.,1.,1.,1.,1.,1.,
1.,1.,1.,1.,1.,1.,1.,1.,1.,1.,1.,1.,1.,1.,1.,1.,1.,1.,1.,1.,1.,1.,1.,1.,
1.,1.,1.,1.,1.,1.,1.,1.,1.,1.,1.,1.,1.,1.,1.,1.,1.,1.,1.,1.,1.,1.,1.,1.,
1.,1.,1.,1.,1.,1.))
REPRESENTATION_ITEM('')
);
#212=(
BOUNDED_CURVE()
B_SPLINE_CURVE(5,(#29003,#29004,#29005,#29006,#29007,#29008,#29009,#29010,
#29011,#29012,#29013,#29014,#29015,#29016,#29017,#29018,#29019,#29020,#29021,
#29022,#29023,#29024,#29025,#29026,#29027,#29028,#29029,#29030,#29031,#29032,
#29033,#29034,#29035,#29036,#29037,#29038,#29039,#29040,#29041,#29042,#29043,
#29044,#29045,#29046,#29047,#29048,#29049,#29050,#29051,#29052,#29053,#29054,
#29055,#29056,#29057,#29058,#29059,#29060,#29061,#29062,#29063,#29064,#29065,
#29066,#29067,#29068,#29069,#29070,#29071,#29072),.UNSPECIFIED.,.F.,.F.)
B_SPLINE_CURVE_WITH_KNOTS((6,1,1,1,1,1,1,1,1,1,1,1,1,1,1,1,1,1,1,1,1,1,
1,1,1,1,1,1,1,1,1,1,1,1,1,1,1,1,1,1,1,1,1,1,1,1,1,1,1,1,1,1,1,1,1,1,1,1,
1,1,1,1,1,1,1,6),(-1.,-0.984615384615383,-0.969230769230768,-0.953846153846152,
-0.938461538461537,-0.923076923076922,-0.907692307692306,-0.892307692307691,
-0.876923076923076,-0.86153846153846,-0.846153846153845,-0.83076923076923,
-0.815384615384614,-0.799999999999999,-0.784615384615384,-0.769230769230768,
-0.753846153846153,-0.738461538461538,-0.723076923076922,-0.707692307692307,
-0.692307692307692,-0.676923076923076,-0.661538461538461,-0.646153846153846,
-0.63076923076923,-0.615384615384615,-0.6,-0.584615384615384,-0.569230769230769,
-0.553846153846154,-0.538461538461538,-0.523076923076923,-0.507692307692308,
-0.492307692307692,-0.476923076923077,-0.461538461538462,-0.446153846153846,
-0.430769230769231,-0.415384615384615,-0.4,-0.384615384615385,-0.369230769230769,
-0.353846153846154,-0.338461538461538,-0.323076923076923,-0.307692307692308,
-0.292307692307692,-0.276923076923077,-0.261538461538462,-0.246153846153846,
-0.230769230769231,-0.215384615384615,-0.2,-0.184615384615385,-0.169230769230769,
-0.153846153846154,-0.138461538461538,-0.123076923076923,-0.107692307692308,
-0.0923076923076923,-0.0769230769230769,-0.0615384615384615,-0.0461538461538462,
-0.0307692307692308,-0.0153846153846154,0.),.UNSPECIFIED.)
CURVE()
GEOMETRIC_REPRESENTATION_ITEM()
RATIONAL_B_SPLINE_CURVE((1.,1.,1.,1.,1.,1.,1.,1.,1.,1.,1.,1.,1.,1.,1.,1.,
1.,1.,1.,1.,1.,1.,1.,1.,1.,1.,1.,1.,1.,1.,1.,1.,1.,1.,1.,1.,1.,1.,1.,1.,
1.,1.,1.,1.,1.,1.,1.,1.,1.,1.,1.,1.,1.,1.,1.,1.,1.,1.,1.,1.,1.,1.,1.,1.,
1.,1.,1.,1.,1.,1.))
REPRESENTATION_ITEM('')
);
#213=(
BOUNDED_CURVE()
B_SPLINE_CURVE(5,(#29219,#29220,#29221,#29222,#29223,#29224,#29225,#29226,
#29227,#29228,#29229,#29230,#29231,#29232,#29233,#29234,#29235,#29236,#29237,
#29238,#29239,#29240,#29241,#29242,#29243,#29244,#29245,#29246,#29247,#29248,
#29249,#29250,#29251,#29252,#29253,#29254,#29255,#29256,#29257,#29258,#29259,
#29260,#29261,#29262,#29263,#29264,#29265,#29266,#29267,#29268,#29269,#29270,
#29271,#29272,#29273,#29274,#29275,#29276,#29277,#29278,#29279,#29280,#29281,
#29282,#29283,#29284,#29285,#29286,#29287,#29288),.UNSPECIFIED.,.F.,.F.)
B_SPLINE_CURVE_WITH_KNOTS((6,1,1,1,1,1,1,1,1,1,1,1,1,1,1,1,1,1,1,1,1,1,
1,1,1,1,1,1,1,1,1,1,1,1,1,1,1,1,1,1,1,1,1,1,1,1,1,1,1,1,1,1,1,1,1,1,1,1,
1,1,1,1,1,1,1,6),(-1.,-0.984615384615383,-0.969230769230768,-0.953846153846152,
-0.938461538461537,-0.923076923076922,-0.907692307692306,-0.892307692307691,
-0.876923076923076,-0.86153846153846,-0.846153846153845,-0.83076923076923,
-0.815384615384614,-0.799999999999999,-0.784615384615384,-0.769230769230768,
-0.753846153846153,-0.738461538461538,-0.723076923076922,-0.707692307692307,
-0.692307692307692,-0.676923076923076,-0.661538461538461,-0.646153846153846,
-0.63076923076923,-0.615384615384615,-0.6,-0.584615384615384,-0.569230769230769,
-0.553846153846154,-0.538461538461538,-0.523076923076923,-0.507692307692308,
-0.492307692307692,-0.476923076923077,-0.461538461538462,-0.446153846153846,
-0.430769230769231,-0.415384615384615,-0.4,-0.384615384615385,-0.369230769230769,
-0.353846153846154,-0.338461538461538,-0.323076923076923,-0.307692307692308,
-0.292307692307692,-0.276923076923077,-0.261538461538462,-0.246153846153846,
-0.230769230769231,-0.215384615384615,-0.2,-0.184615384615385,-0.169230769230769,
-0.153846153846154,-0.138461538461538,-0.123076923076923,-0.107692307692308,
-0.0923076923076923,-0.0769230769230769,-0.0615384615384615,-0.0461538461538462,
-0.0307692307692308,-0.0153846153846154,0.),.UNSPECIFIED.)
CURVE()
GEOMETRIC_REPRESENTATION_ITEM()
RATIONAL_B_SPLINE_CURVE((1.,1.,1.,1.,1.,1.,1.,1.,1.,1.,1.,1.,1.,1.,1.,1.,
1.,1.,1.,1.,1.,1.,1.,1.,1.,1.,1.,1.,1.,1.,1.,1.,1.,1.,1.,1.,1.,1.,1.,1.,
1.,1.,1.,1.,1.,1.,1.,1.,1.,1.,1.,1.,1.,1.,1.,1.,1.,1.,1.,1.,1.,1.,1.,1.,
1.,1.,1.,1.,1.,1.))
REPRESENTATION_ITEM('')
);
#214=(
BOUNDED_CURVE()
B_SPLINE_CURVE(5,(#29435,#29436,#29437,#29438,#29439,#29440,#29441,#29442,
#29443,#29444,#29445,#29446,#29447,#29448,#29449,#29450,#29451,#29452,#29453,
#29454,#29455,#29456,#29457,#29458,#29459,#29460,#29461,#29462,#29463,#29464,
#29465,#29466,#29467,#29468,#29469,#29470,#29471,#29472,#29473,#29474,#29475,
#29476,#29477,#29478,#29479,#29480,#29481,#29482,#29483,#29484,#29485,#29486,
#29487,#29488,#29489,#29490,#29491,#29492,#29493,#29494,#29495,#29496,#29497,
#29498,#29499,#29500,#29501,#29502,#29503,#29504),.UNSPECIFIED.,.F.,.F.)
B_SPLINE_CURVE_WITH_KNOTS((6,1,1,1,1,1,1,1,1,1,1,1,1,1,1,1,1,1,1,1,1,1,
1,1,1,1,1,1,1,1,1,1,1,1,1,1,1,1,1,1,1,1,1,1,1,1,1,1,1,1,1,1,1,1,1,1,1,1,
1,1,1,1,1,1,1,6),(-1.,-0.984615384615383,-0.969230769230768,-0.953846153846152,
-0.938461538461537,-0.923076923076922,-0.907692307692306,-0.892307692307691,
-0.876923076923076,-0.86153846153846,-0.846153846153845,-0.83076923076923,
-0.815384615384614,-0.799999999999999,-0.784615384615384,-0.769230769230768,
-0.753846153846153,-0.738461538461538,-0.723076923076922,-0.707692307692307,
-0.692307692307692,-0.676923076923076,-0.661538461538461,-0.646153846153846,
-0.63076923076923,-0.615384615384615,-0.6,-0.584615384615384,-0.569230769230769,
-0.553846153846154,-0.538461538461538,-0.523076923076923,-0.507692307692308,
-0.492307692307692,-0.476923076923077,-0.461538461538462,-0.446153846153846,
-0.430769230769231,-0.415384615384615,-0.4,-0.384615384615385,-0.369230769230769,
-0.353846153846154,-0.338461538461538,-0.323076923076923,-0.307692307692308,
-0.292307692307692,-0.276923076923077,-0.261538461538462,-0.246153846153846,
-0.230769230769231,-0.215384615384615,-0.2,-0.184615384615385,-0.169230769230769,
-0.153846153846154,-0.138461538461538,-0.123076923076923,-0.107692307692308,
-0.0923076923076923,-0.0769230769230769,-0.0615384615384615,-0.0461538461538462,
-0.0307692307692308,-0.0153846153846154,0.),.UNSPECIFIED.)
CURVE()
GEOMETRIC_REPRESENTATION_ITEM()
RATIONAL_B_SPLINE_CURVE((1.,1.,1.,1.,1.,1.,1.,1.,1.,1.,1.,1.,1.,1.,1.,1.,
1.,1.,1.,1.,1.,1.,1.,1.,1.,1.,1.,1.,1.,1.,1.,1.,1.,1.,1.,1.,1.,1.,1.,1.,
1.,1.,1.,1.,1.,1.,1.,1.,1.,1.,1.,1.,1.,1.,1.,1.,1.,1.,1.,1.,1.,1.,1.,1.,
1.,1.,1.,1.,1.,1.))
REPRESENTATION_ITEM('')
);
#215=(
BOUNDED_CURVE()
B_SPLINE_CURVE(5,(#29651,#29652,#29653,#29654,#29655,#29656,#29657,#29658,
#29659,#29660,#29661,#29662,#29663,#29664,#29665,#29666,#29667,#29668,#29669,
#29670,#29671,#29672,#29673,#29674,#29675,#29676,#29677,#29678,#29679,#29680,
#29681,#29682,#29683,#29684,#29685,#29686,#29687,#29688,#29689,#29690,#29691,
#29692,#29693,#29694,#29695,#29696,#29697,#29698,#29699,#29700,#29701,#29702,
#29703,#29704,#29705,#29706,#29707,#29708,#29709,#29710,#29711,#29712,#29713,
#29714,#29715,#29716,#29717,#29718,#29719,#29720),.UNSPECIFIED.,.F.,.F.)
B_SPLINE_CURVE_WITH_KNOTS((6,1,1,1,1,1,1,1,1,1,1,1,1,1,1,1,1,1,1,1,1,1,
1,1,1,1,1,1,1,1,1,1,1,1,1,1,1,1,1,1,1,1,1,1,1,1,1,1,1,1,1,1,1,1,1,1,1,1,
1,1,1,1,1,1,1,6),(-1.,-0.984615384615383,-0.969230769230768,-0.953846153846152,
-0.938461538461537,-0.923076923076922,-0.907692307692306,-0.892307692307691,
-0.876923076923076,-0.86153846153846,-0.846153846153845,-0.83076923076923,
-0.815384615384614,-0.799999999999999,-0.784615384615384,-0.769230769230768,
-0.753846153846153,-0.738461538461538,-0.723076923076922,-0.707692307692307,
-0.692307692307692,-0.676923076923076,-0.661538461538461,-0.646153846153846,
-0.63076923076923,-0.615384615384615,-0.6,-0.584615384615384,-0.569230769230769,
-0.553846153846154,-0.538461538461538,-0.523076923076923,-0.507692307692308,
-0.492307692307692,-0.476923076923077,-0.461538461538462,-0.446153846153846,
-0.430769230769231,-0.415384615384615,-0.4,-0.384615384615385,-0.369230769230769,
-0.353846153846154,-0.338461538461538,-0.323076923076923,-0.307692307692308,
-0.292307692307692,-0.276923076923077,-0.261538461538462,-0.246153846153846,
-0.230769230769231,-0.215384615384615,-0.2,-0.184615384615385,-0.169230769230769,
-0.153846153846154,-0.138461538461538,-0.123076923076923,-0.107692307692308,
-0.0923076923076923,-0.0769230769230769,-0.0615384615384615,-0.0461538461538462,
-0.0307692307692308,-0.0153846153846154,0.),.UNSPECIFIED.)
CURVE()
GEOMETRIC_REPRESENTATION_ITEM()
RATIONAL_B_SPLINE_CURVE((1.,1.,1.,1.,1.,1.,1.,1.,1.,1.,1.,1.,1.,1.,1.,1.,
1.,1.,1.,1.,1.,1.,1.,1.,1.,1.,1.,1.,1.,1.,1.,1.,1.,1.,1.,1.,1.,1.,1.,1.,
1.,1.,1.,1.,1.,1.,1.,1.,1.,1.,1.,1.,1.,1.,1.,1.,1.,1.,1.,1.,1.,1.,1.,1.,
1.,1.,1.,1.,1.,1.))
REPRESENTATION_ITEM('')
);
#216=(
BOUNDED_CURVE()
B_SPLINE_CURVE(5,(#29867,#29868,#29869,#29870,#29871,#29872,#29873,#29874,
#29875,#29876,#29877,#29878,#29879,#29880,#29881,#29882,#29883,#29884,#29885,
#29886,#29887,#29888,#29889,#29890,#29891,#29892,#29893,#29894,#29895,#29896,
#29897,#29898,#29899,#29900,#29901,#29902,#29903,#29904,#29905,#29906,#29907,
#29908,#29909,#29910,#29911,#29912,#29913,#29914,#29915,#29916,#29917,#29918,
#29919,#29920,#29921,#29922,#29923,#29924,#29925,#29926,#29927,#29928,#29929,
#29930,#29931,#29932,#29933,#29934,#29935,#29936),.UNSPECIFIED.,.F.,.F.)
B_SPLINE_CURVE_WITH_KNOTS((6,1,1,1,1,1,1,1,1,1,1,1,1,1,1,1,1,1,1,1,1,1,
1,1,1,1,1,1,1,1,1,1,1,1,1,1,1,1,1,1,1,1,1,1,1,1,1,1,1,1,1,1,1,1,1,1,1,1,
1,1,1,1,1,1,1,6),(-1.,-0.984615384615383,-0.969230769230768,-0.953846153846152,
-0.938461538461537,-0.923076923076922,-0.907692307692306,-0.892307692307691,
-0.876923076923076,-0.86153846153846,-0.846153846153845,-0.83076923076923,
-0.815384615384614,-0.799999999999999,-0.784615384615384,-0.769230769230768,
-0.753846153846153,-0.738461538461538,-0.723076923076922,-0.707692307692307,
-0.692307692307692,-0.676923076923076,-0.661538461538461,-0.646153846153846,
-0.63076923076923,-0.615384615384615,-0.6,-0.584615384615384,-0.569230769230769,
-0.553846153846154,-0.538461538461538,-0.523076923076923,-0.507692307692308,
-0.492307692307692,-0.476923076923077,-0.461538461538462,-0.446153846153846,
-0.430769230769231,-0.415384615384615,-0.4,-0.384615384615385,-0.369230769230769,
-0.353846153846154,-0.338461538461538,-0.323076923076923,-0.307692307692308,
-0.292307692307692,-0.276923076923077,-0.261538461538462,-0.246153846153846,
-0.230769230769231,-0.215384615384615,-0.2,-0.184615384615385,-0.169230769230769,
-0.153846153846154,-0.138461538461538,-0.123076923076923,-0.107692307692308,
-0.0923076923076923,-0.0769230769230769,-0.0615384615384615,-0.0461538461538462,
-0.0307692307692308,-0.0153846153846154,0.),.UNSPECIFIED.)
CURVE()
GEOMETRIC_REPRESENTATION_ITEM()
RATIONAL_B_SPLINE_CURVE((1.,1.,1.,1.,1.,1.,1.,1.,1.,1.,1.,1.,1.,1.,1.,1.,
1.,1.,1.,1.,1.,1.,1.,1.,1.,1.,1.,1.,1.,1.,1.,1.,1.,1.,1.,1.,1.,1.,1.,1.,
1.,1.,1.,1.,1.,1.,1.,1.,1.,1.,1.,1.,1.,1.,1.,1.,1.,1.,1.,1.,1.,1.,1.,1.,
1.,1.,1.,1.,1.,1.))
REPRESENTATION_ITEM('')
);
#217=(
BOUNDED_CURVE()
B_SPLINE_CURVE(5,(#30083,#30084,#30085,#30086,#30087,#30088,#30089,#30090,
#30091,#30092,#30093,#30094,#30095,#30096,#30097,#30098,#30099,#30100,#30101,
#30102,#30103,#30104,#30105,#30106,#30107,#30108,#30109,#30110,#30111,#30112,
#30113,#30114,#30115,#30116,#30117,#30118,#30119,#30120,#30121,#30122,#30123,
#30124,#30125,#30126,#30127,#30128,#30129,#30130,#30131,#30132,#30133,#30134,
#30135,#30136,#30137,#30138,#30139,#30140,#30141,#30142,#30143,#30144,#30145,
#30146,#30147,#30148,#30149,#30150,#30151,#30152),.UNSPECIFIED.,.F.,.F.)
B_SPLINE_CURVE_WITH_KNOTS((6,1,1,1,1,1,1,1,1,1,1,1,1,1,1,1,1,1,1,1,1,1,
1,1,1,1,1,1,1,1,1,1,1,1,1,1,1,1,1,1,1,1,1,1,1,1,1,1,1,1,1,1,1,1,1,1,1,1,
1,1,1,1,1,1,1,6),(-1.,-0.984615384615383,-0.969230769230768,-0.953846153846152,
-0.938461538461537,-0.923076923076922,-0.907692307692306,-0.892307692307691,
-0.876923076923076,-0.86153846153846,-0.846153846153845,-0.83076923076923,
-0.815384615384614,-0.799999999999999,-0.784615384615384,-0.769230769230768,
-0.753846153846153,-0.738461538461538,-0.723076923076922,-0.707692307692307,
-0.692307692307692,-0.676923076923076,-0.661538461538461,-0.646153846153846,
-0.63076923076923,-0.615384615384615,-0.6,-0.584615384615384,-0.569230769230769,
-0.553846153846154,-0.538461538461538,-0.523076923076923,-0.507692307692308,
-0.492307692307692,-0.476923076923077,-0.461538461538462,-0.446153846153846,
-0.430769230769231,-0.415384615384615,-0.4,-0.384615384615385,-0.369230769230769,
-0.353846153846154,-0.338461538461538,-0.323076923076923,-0.307692307692308,
-0.292307692307692,-0.276923076923077,-0.261538461538462,-0.246153846153846,
-0.230769230769231,-0.215384615384615,-0.2,-0.184615384615385,-0.169230769230769,
-0.153846153846154,-0.138461538461538,-0.123076923076923,-0.107692307692308,
-0.0923076923076923,-0.0769230769230769,-0.0615384615384615,-0.0461538461538462,
-0.0307692307692308,-0.0153846153846154,0.),.UNSPECIFIED.)
CURVE()
GEOMETRIC_REPRESENTATION_ITEM()
RATIONAL_B_SPLINE_CURVE((1.,1.,1.,1.,1.,1.,1.,1.,1.,1.,1.,1.,1.,1.,1.,1.,
1.,1.,1.,1.,1.,1.,1.,1.,1.,1.,1.,1.,1.,1.,1.,1.,1.,1.,1.,1.,1.,1.,1.,1.,
1.,1.,1.,1.,1.,1.,1.,1.,1.,1.,1.,1.,1.,1.,1.,1.,1.,1.,1.,1.,1.,1.,1.,1.,
1.,1.,1.,1.,1.,1.))
REPRESENTATION_ITEM('')
);
#218=(
BOUNDED_CURVE()
B_SPLINE_CURVE(5,(#30299,#30300,#30301,#30302,#30303,#30304,#30305,#30306,
#30307,#30308,#30309,#30310,#30311,#30312,#30313,#30314,#30315,#30316,#30317,
#30318,#30319,#30320,#30321,#30322,#30323,#30324,#30325,#30326,#30327,#30328,
#30329,#30330,#30331,#30332,#30333,#30334,#30335,#30336,#30337,#30338,#30339,
#30340,#30341,#30342,#30343,#30344,#30345,#30346,#30347,#30348,#30349,#30350,
#30351,#30352,#30353,#30354,#30355,#30356,#30357,#30358,#30359,#30360,#30361,
#30362,#30363,#30364,#30365,#30366,#30367,#30368),.UNSPECIFIED.,.F.,.F.)
B_SPLINE_CURVE_WITH_KNOTS((6,1,1,1,1,1,1,1,1,1,1,1,1,1,1,1,1,1,1,1,1,1,
1,1,1,1,1,1,1,1,1,1,1,1,1,1,1,1,1,1,1,1,1,1,1,1,1,1,1,1,1,1,1,1,1,1,1,1,
1,1,1,1,1,1,1,6),(-1.,-0.984615384615383,-0.969230769230768,-0.953846153846152,
-0.938461538461537,-0.923076923076922,-0.907692307692306,-0.892307692307691,
-0.876923076923076,-0.86153846153846,-0.846153846153845,-0.83076923076923,
-0.815384615384614,-0.799999999999999,-0.784615384615384,-0.769230769230768,
-0.753846153846153,-0.738461538461538,-0.723076923076922,-0.707692307692307,
-0.692307692307692,-0.676923076923076,-0.661538461538461,-0.646153846153846,
-0.63076923076923,-0.615384615384615,-0.6,-0.584615384615384,-0.569230769230769,
-0.553846153846154,-0.538461538461538,-0.523076923076923,-0.507692307692308,
-0.492307692307692,-0.476923076923077,-0.461538461538462,-0.446153846153846,
-0.430769230769231,-0.415384615384615,-0.4,-0.384615384615385,-0.369230769230769,
-0.353846153846154,-0.338461538461538,-0.323076923076923,-0.307692307692308,
-0.292307692307692,-0.276923076923077,-0.261538461538462,-0.246153846153846,
-0.230769230769231,-0.215384615384615,-0.2,-0.184615384615385,-0.169230769230769,
-0.153846153846154,-0.138461538461538,-0.123076923076923,-0.107692307692308,
-0.0923076923076923,-0.0769230769230769,-0.0615384615384615,-0.0461538461538462,
-0.0307692307692308,-0.0153846153846154,0.),.UNSPECIFIED.)
CURVE()
GEOMETRIC_REPRESENTATION_ITEM()
RATIONAL_B_SPLINE_CURVE((1.,1.,1.,1.,1.,1.,1.,1.,1.,1.,1.,1.,1.,1.,1.,1.,
1.,1.,1.,1.,1.,1.,1.,1.,1.,1.,1.,1.,1.,1.,1.,1.,1.,1.,1.,1.,1.,1.,1.,1.,
1.,1.,1.,1.,1.,1.,1.,1.,1.,1.,1.,1.,1.,1.,1.,1.,1.,1.,1.,1.,1.,1.,1.,1.,
1.,1.,1.,1.,1.,1.))
REPRESENTATION_ITEM('')
);
#219=(
BOUNDED_CURVE()
B_SPLINE_CURVE(5,(#30515,#30516,#30517,#30518,#30519,#30520,#30521,#30522,
#30523,#30524,#30525,#30526,#30527,#30528,#30529,#30530,#30531,#30532,#30533,
#30534,#30535,#30536,#30537,#30538,#30539,#30540,#30541,#30542,#30543,#30544,
#30545,#30546,#30547,#30548,#30549,#30550,#30551,#30552,#30553,#30554,#30555,
#30556,#30557,#30558,#30559,#30560,#30561,#30562,#30563,#30564,#30565,#30566,
#30567,#30568,#30569,#30570,#30571,#30572,#30573,#30574,#30575,#30576,#30577,
#30578,#30579,#30580,#30581,#30582,#30583,#30584),.UNSPECIFIED.,.F.,.F.)
B_SPLINE_CURVE_WITH_KNOTS((6,1,1,1,1,1,1,1,1,1,1,1,1,1,1,1,1,1,1,1,1,1,
1,1,1,1,1,1,1,1,1,1,1,1,1,1,1,1,1,1,1,1,1,1,1,1,1,1,1,1,1,1,1,1,1,1,1,1,
1,1,1,1,1,1,1,6),(-1.,-0.984615384615383,-0.969230769230768,-0.953846153846152,
-0.938461538461537,-0.923076923076922,-0.907692307692306,-0.892307692307691,
-0.876923076923076,-0.86153846153846,-0.846153846153845,-0.83076923076923,
-0.815384615384614,-0.799999999999999,-0.784615384615384,-0.769230769230768,
-0.753846153846153,-0.738461538461538,-0.723076923076922,-0.707692307692307,
-0.692307692307692,-0.676923076923076,-0.661538461538461,-0.646153846153846,
-0.63076923076923,-0.615384615384615,-0.6,-0.584615384615384,-0.569230769230769,
-0.553846153846154,-0.538461538461538,-0.523076923076923,-0.507692307692308,
-0.492307692307692,-0.476923076923077,-0.461538461538462,-0.446153846153846,
-0.430769230769231,-0.415384615384615,-0.4,-0.384615384615385,-0.369230769230769,
-0.353846153846154,-0.338461538461538,-0.323076923076923,-0.307692307692308,
-0.292307692307692,-0.276923076923077,-0.261538461538462,-0.246153846153846,
-0.230769230769231,-0.215384615384615,-0.2,-0.184615384615385,-0.169230769230769,
-0.153846153846154,-0.138461538461538,-0.123076923076923,-0.107692307692308,
-0.0923076923076923,-0.0769230769230769,-0.0615384615384615,-0.0461538461538462,
-0.0307692307692308,-0.0153846153846154,0.),.UNSPECIFIED.)
CURVE()
GEOMETRIC_REPRESENTATION_ITEM()
RATIONAL_B_SPLINE_CURVE((1.,1.,1.,1.,1.,1.,1.,1.,1.,1.,1.,1.,1.,1.,1.,1.,
1.,1.,1.,1.,1.,1.,1.,1.,1.,1.,1.,1.,1.,1.,1.,1.,1.,1.,1.,1.,1.,1.,1.,1.,
1.,1.,1.,1.,1.,1.,1.,1.,1.,1.,1.,1.,1.,1.,1.,1.,1.,1.,1.,1.,1.,1.,1.,1.,
1.,1.,1.,1.,1.,1.))
REPRESENTATION_ITEM('')
);
#220=(
BOUNDED_CURVE()
B_SPLINE_CURVE(5,(#30731,#30732,#30733,#30734,#30735,#30736,#30737,#30738,
#30739,#30740,#30741,#30742,#30743,#30744,#30745,#30746,#30747,#30748,#30749,
#30750,#30751,#30752,#30753,#30754,#30755,#30756,#30757,#30758,#30759,#30760,
#30761,#30762,#30763,#30764,#30765,#30766,#30767,#30768,#30769,#30770,#30771,
#30772,#30773,#30774,#30775,#30776,#30777,#30778,#30779,#30780,#30781,#30782,
#30783,#30784,#30785,#30786,#30787,#30788,#30789,#30790,#30791,#30792,#30793,
#30794,#30795,#30796,#30797,#30798,#30799,#30800),.UNSPECIFIED.,.F.,.F.)
B_SPLINE_CURVE_WITH_KNOTS((6,1,1,1,1,1,1,1,1,1,1,1,1,1,1,1,1,1,1,1,1,1,
1,1,1,1,1,1,1,1,1,1,1,1,1,1,1,1,1,1,1,1,1,1,1,1,1,1,1,1,1,1,1,1,1,1,1,1,
1,1,1,1,1,1,1,6),(-1.,-0.984615384615383,-0.969230769230768,-0.953846153846152,
-0.938461538461537,-0.923076923076922,-0.907692307692306,-0.892307692307691,
-0.876923076923076,-0.86153846153846,-0.846153846153845,-0.83076923076923,
-0.815384615384614,-0.799999999999999,-0.784615384615384,-0.769230769230768,
-0.753846153846153,-0.738461538461538,-0.723076923076922,-0.707692307692307,
-0.692307692307692,-0.676923076923076,-0.661538461538461,-0.646153846153846,
-0.63076923076923,-0.615384615384615,-0.6,-0.584615384615384,-0.569230769230769,
-0.553846153846154,-0.538461538461538,-0.523076923076923,-0.507692307692308,
-0.492307692307692,-0.476923076923077,-0.461538461538462,-0.446153846153846,
-0.430769230769231,-0.415384615384615,-0.4,-0.384615384615385,-0.369230769230769,
-0.353846153846154,-0.338461538461538,-0.323076923076923,-0.307692307692308,
-0.292307692307692,-0.276923076923077,-0.261538461538462,-0.246153846153846,
-0.230769230769231,-0.215384615384615,-0.2,-0.184615384615385,-0.169230769230769,
-0.153846153846154,-0.138461538461538,-0.123076923076923,-0.107692307692308,
-0.0923076923076923,-0.0769230769230769,-0.0615384615384615,-0.0461538461538462,
-0.0307692307692308,-0.0153846153846154,0.),.UNSPECIFIED.)
CURVE()
GEOMETRIC_REPRESENTATION_ITEM()
RATIONAL_B_SPLINE_CURVE((1.,1.,1.,1.,1.,1.,1.,1.,1.,1.,1.,1.,1.,1.,1.,1.,
1.,1.,1.,1.,1.,1.,1.,1.,1.,1.,1.,1.,1.,1.,1.,1.,1.,1.,1.,1.,1.,1.,1.,1.,
1.,1.,1.,1.,1.,1.,1.,1.,1.,1.,1.,1.,1.,1.,1.,1.,1.,1.,1.,1.,1.,1.,1.,1.,
1.,1.,1.,1.,1.,1.))
REPRESENTATION_ITEM('')
);
#221=(
BOUNDED_CURVE()
B_SPLINE_CURVE(5,(#30947,#30948,#30949,#30950,#30951,#30952,#30953,#30954,
#30955,#30956,#30957,#30958,#30959,#30960,#30961,#30962,#30963,#30964,#30965,
#30966,#30967,#30968,#30969,#30970,#30971,#30972,#30973,#30974,#30975,#30976,
#30977,#30978,#30979,#30980,#30981,#30982,#30983,#30984,#30985,#30986,#30987,
#30988,#30989,#30990,#30991,#30992,#30993,#30994,#30995,#30996,#30997,#30998,
#30999,#31000,#31001,#31002,#31003,#31004,#31005,#31006,#31007,#31008,#31009,
#31010,#31011,#31012,#31013,#31014,#31015,#31016),.UNSPECIFIED.,.F.,.F.)
B_SPLINE_CURVE_WITH_KNOTS((6,1,1,1,1,1,1,1,1,1,1,1,1,1,1,1,1,1,1,1,1,1,
1,1,1,1,1,1,1,1,1,1,1,1,1,1,1,1,1,1,1,1,1,1,1,1,1,1,1,1,1,1,1,1,1,1,1,1,
1,1,1,1,1,1,1,6),(-1.,-0.984615384615383,-0.969230769230768,-0.953846153846152,
-0.938461538461537,-0.923076923076922,-0.907692307692306,-0.892307692307691,
-0.876923076923076,-0.86153846153846,-0.846153846153845,-0.83076923076923,
-0.815384615384614,-0.799999999999999,-0.784615384615384,-0.769230769230768,
-0.753846153846153,-0.738461538461538,-0.723076923076922,-0.707692307692307,
-0.692307692307692,-0.676923076923076,-0.661538461538461,-0.646153846153846,
-0.63076923076923,-0.615384615384615,-0.6,-0.584615384615384,-0.569230769230769,
-0.553846153846154,-0.538461538461538,-0.523076923076923,-0.507692307692308,
-0.492307692307692,-0.476923076923077,-0.461538461538462,-0.446153846153846,
-0.430769230769231,-0.415384615384615,-0.4,-0.384615384615385,-0.369230769230769,
-0.353846153846154,-0.338461538461538,-0.323076923076923,-0.307692307692308,
-0.292307692307692,-0.276923076923077,-0.261538461538462,-0.246153846153846,
-0.230769230769231,-0.215384615384615,-0.2,-0.184615384615385,-0.169230769230769,
-0.153846153846154,-0.138461538461538,-0.123076923076923,-0.107692307692308,
-0.0923076923076923,-0.0769230769230769,-0.0615384615384615,-0.0461538461538462,
-0.0307692307692308,-0.0153846153846154,0.),.UNSPECIFIED.)
CURVE()
GEOMETRIC_REPRESENTATION_ITEM()
RATIONAL_B_SPLINE_CURVE((1.,1.,1.,1.,1.,1.,1.,1.,1.,1.,1.,1.,1.,1.,1.,1.,
1.,1.,1.,1.,1.,1.,1.,1.,1.,1.,1.,1.,1.,1.,1.,1.,1.,1.,1.,1.,1.,1.,1.,1.,
1.,1.,1.,1.,1.,1.,1.,1.,1.,1.,1.,1.,1.,1.,1.,1.,1.,1.,1.,1.,1.,1.,1.,1.,
1.,1.,1.,1.,1.,1.))
REPRESENTATION_ITEM('')
);
#222=(
BOUNDED_CURVE()
B_SPLINE_CURVE(5,(#31163,#31164,#31165,#31166,#31167,#31168,#31169,#31170,
#31171,#31172,#31173,#31174,#31175,#31176,#31177,#31178,#31179,#31180,#31181,
#31182,#31183,#31184,#31185,#31186,#31187,#31188,#31189,#31190,#31191,#31192,
#31193,#31194,#31195,#31196,#31197,#31198,#31199,#31200,#31201,#31202,#31203,
#31204,#31205,#31206,#31207,#31208,#31209,#31210,#31211,#31212,#31213,#31214,
#31215,#31216,#31217,#31218,#31219,#31220,#31221,#31222,#31223,#31224,#31225,
#31226,#31227,#31228,#31229,#31230,#31231,#31232),.UNSPECIFIED.,.F.,.F.)
B_SPLINE_CURVE_WITH_KNOTS((6,1,1,1,1,1,1,1,1,1,1,1,1,1,1,1,1,1,1,1,1,1,
1,1,1,1,1,1,1,1,1,1,1,1,1,1,1,1,1,1,1,1,1,1,1,1,1,1,1,1,1,1,1,1,1,1,1,1,
1,1,1,1,1,1,1,6),(-1.,-0.984615384615383,-0.969230769230768,-0.953846153846152,
-0.938461538461537,-0.923076923076922,-0.907692307692306,-0.892307692307691,
-0.876923076923076,-0.86153846153846,-0.846153846153845,-0.83076923076923,
-0.815384615384614,-0.799999999999999,-0.784615384615384,-0.769230769230768,
-0.753846153846153,-0.738461538461538,-0.723076923076922,-0.707692307692307,
-0.692307692307692,-0.676923076923076,-0.661538461538461,-0.646153846153846,
-0.63076923076923,-0.615384615384615,-0.6,-0.584615384615384,-0.569230769230769,
-0.553846153846154,-0.538461538461538,-0.523076923076923,-0.507692307692308,
-0.492307692307692,-0.476923076923077,-0.461538461538462,-0.446153846153846,
-0.430769230769231,-0.415384615384615,-0.4,-0.384615384615385,-0.369230769230769,
-0.353846153846154,-0.338461538461538,-0.323076923076923,-0.307692307692308,
-0.292307692307692,-0.276923076923077,-0.261538461538462,-0.246153846153846,
-0.230769230769231,-0.215384615384615,-0.2,-0.184615384615385,-0.169230769230769,
-0.153846153846154,-0.138461538461538,-0.123076923076923,-0.107692307692308,
-0.0923076923076923,-0.0769230769230769,-0.0615384615384615,-0.0461538461538462,
-0.0307692307692308,-0.0153846153846154,0.),.UNSPECIFIED.)
CURVE()
GEOMETRIC_REPRESENTATION_ITEM()
RATIONAL_B_SPLINE_CURVE((1.,1.,1.,1.,1.,1.,1.,1.,1.,1.,1.,1.,1.,1.,1.,1.,
1.,1.,1.,1.,1.,1.,1.,1.,1.,1.,1.,1.,1.,1.,1.,1.,1.,1.,1.,1.,1.,1.,1.,1.,
1.,1.,1.,1.,1.,1.,1.,1.,1.,1.,1.,1.,1.,1.,1.,1.,1.,1.,1.,1.,1.,1.,1.,1.,
1.,1.,1.,1.,1.,1.))
REPRESENTATION_ITEM('')
);
#223=(
BOUNDED_CURVE()
B_SPLINE_CURVE(5,(#31379,#31380,#31381,#31382,#31383,#31384,#31385,#31386,
#31387,#31388,#31389,#31390,#31391,#31392,#31393,#31394,#31395,#31396,#31397,
#31398,#31399,#31400,#31401,#31402,#31403,#31404,#31405,#31406,#31407,#31408,
#31409,#31410,#31411,#31412,#31413,#31414,#31415,#31416,#31417,#31418,#31419,
#31420,#31421,#31422,#31423,#31424,#31425,#31426,#31427,#31428,#31429,#31430,
#31431,#31432,#31433,#31434,#31435,#31436,#31437,#31438,#31439,#31440,#31441,
#31442,#31443,#31444,#31445,#31446,#31447,#31448),.UNSPECIFIED.,.F.,.F.)
B_SPLINE_CURVE_WITH_KNOTS((6,1,1,1,1,1,1,1,1,1,1,1,1,1,1,1,1,1,1,1,1,1,
1,1,1,1,1,1,1,1,1,1,1,1,1,1,1,1,1,1,1,1,1,1,1,1,1,1,1,1,1,1,1,1,1,1,1,1,
1,1,1,1,1,1,1,6),(-1.,-0.984615384615383,-0.969230769230768,-0.953846153846152,
-0.938461538461537,-0.923076923076922,-0.907692307692306,-0.892307692307691,
-0.876923076923076,-0.86153846153846,-0.846153846153845,-0.83076923076923,
-0.815384615384614,-0.799999999999999,-0.784615384615384,-0.769230769230768,
-0.753846153846153,-0.738461538461538,-0.723076923076922,-0.707692307692307,
-0.692307692307692,-0.676923076923076,-0.661538461538461,-0.646153846153846,
-0.63076923076923,-0.615384615384615,-0.6,-0.584615384615384,-0.569230769230769,
-0.553846153846154,-0.538461538461538,-0.523076923076923,-0.507692307692308,
-0.492307692307692,-0.476923076923077,-0.461538461538462,-0.446153846153846,
-0.430769230769231,-0.415384615384615,-0.4,-0.384615384615385,-0.369230769230769,
-0.353846153846154,-0.338461538461538,-0.323076923076923,-0.307692307692308,
-0.292307692307692,-0.276923076923077,-0.261538461538462,-0.246153846153846,
-0.230769230769231,-0.215384615384615,-0.2,-0.184615384615385,-0.169230769230769,
-0.153846153846154,-0.138461538461538,-0.123076923076923,-0.107692307692308,
-0.0923076923076923,-0.0769230769230769,-0.0615384615384615,-0.0461538461538462,
-0.0307692307692308,-0.0153846153846154,0.),.UNSPECIFIED.)
CURVE()
GEOMETRIC_REPRESENTATION_ITEM()
RATIONAL_B_SPLINE_CURVE((1.,1.,1.,1.,1.,1.,1.,1.,1.,1.,1.,1.,1.,1.,1.,1.,
1.,1.,1.,1.,1.,1.,1.,1.,1.,1.,1.,1.,1.,1.,1.,1.,1.,1.,1.,1.,1.,1.,1.,1.,
1.,1.,1.,1.,1.,1.,1.,1.,1.,1.,1.,1.,1.,1.,1.,1.,1.,1.,1.,1.,1.,1.,1.,1.,
1.,1.,1.,1.,1.,1.))
REPRESENTATION_ITEM('')
);
#224=(
BOUNDED_CURVE()
B_SPLINE_CURVE(5,(#31595,#31596,#31597,#31598,#31599,#31600,#31601,#31602,
#31603,#31604,#31605,#31606,#31607,#31608,#31609,#31610,#31611,#31612,#31613,
#31614,#31615,#31616,#31617,#31618,#31619,#31620,#31621,#31622,#31623,#31624,
#31625,#31626,#31627,#31628,#31629,#31630,#31631,#31632,#31633,#31634,#31635,
#31636,#31637,#31638,#31639,#31640,#31641,#31642,#31643,#31644,#31645,#31646,
#31647,#31648,#31649,#31650,#31651,#31652,#31653,#31654,#31655,#31656,#31657,
#31658,#31659,#31660,#31661,#31662,#31663,#31664),.UNSPECIFIED.,.F.,.F.)
B_SPLINE_CURVE_WITH_KNOTS((6,1,1,1,1,1,1,1,1,1,1,1,1,1,1,1,1,1,1,1,1,1,
1,1,1,1,1,1,1,1,1,1,1,1,1,1,1,1,1,1,1,1,1,1,1,1,1,1,1,1,1,1,1,1,1,1,1,1,
1,1,1,1,1,1,1,6),(-1.,-0.984615384615383,-0.969230769230768,-0.953846153846152,
-0.938461538461537,-0.923076923076922,-0.907692307692306,-0.892307692307691,
-0.876923076923076,-0.86153846153846,-0.846153846153845,-0.83076923076923,
-0.815384615384614,-0.799999999999999,-0.784615384615384,-0.769230769230768,
-0.753846153846153,-0.738461538461538,-0.723076923076922,-0.707692307692307,
-0.692307692307692,-0.676923076923076,-0.661538461538461,-0.646153846153846,
-0.63076923076923,-0.615384615384615,-0.6,-0.584615384615384,-0.569230769230769,
-0.553846153846154,-0.538461538461538,-0.523076923076923,-0.507692307692308,
-0.492307692307692,-0.476923076923077,-0.461538461538462,-0.446153846153846,
-0.430769230769231,-0.415384615384615,-0.4,-0.384615384615385,-0.369230769230769,
-0.353846153846154,-0.338461538461538,-0.323076923076923,-0.307692307692308,
-0.292307692307692,-0.276923076923077,-0.261538461538462,-0.246153846153846,
-0.230769230769231,-0.215384615384615,-0.2,-0.184615384615385,-0.169230769230769,
-0.153846153846154,-0.138461538461538,-0.123076923076923,-0.107692307692308,
-0.0923076923076923,-0.0769230769230769,-0.0615384615384615,-0.0461538461538462,
-0.0307692307692308,-0.0153846153846154,0.),.UNSPECIFIED.)
CURVE()
GEOMETRIC_REPRESENTATION_ITEM()
RATIONAL_B_SPLINE_CURVE((1.,1.,1.,1.,1.,1.,1.,1.,1.,1.,1.,1.,1.,1.,1.,1.,
1.,1.,1.,1.,1.,1.,1.,1.,1.,1.,1.,1.,1.,1.,1.,1.,1.,1.,1.,1.,1.,1.,1.,1.,
1.,1.,1.,1.,1.,1.,1.,1.,1.,1.,1.,1.,1.,1.,1.,1.,1.,1.,1.,1.,1.,1.,1.,1.,
1.,1.,1.,1.,1.,1.))
REPRESENTATION_ITEM('')
);
#225=(
BOUNDED_CURVE()
B_SPLINE_CURVE(5,(#31811,#31812,#31813,#31814,#31815,#31816,#31817,#31818,
#31819,#31820,#31821,#31822,#31823,#31824,#31825,#31826,#31827,#31828,#31829,
#31830,#31831,#31832,#31833,#31834,#31835,#31836,#31837,#31838,#31839,#31840,
#31841,#31842,#31843,#31844,#31845,#31846,#31847,#31848,#31849,#31850,#31851,
#31852,#31853,#31854,#31855,#31856,#31857,#31858,#31859,#31860,#31861,#31862,
#31863,#31864,#31865,#31866,#31867,#31868,#31869,#31870,#31871,#31872,#31873,
#31874,#31875,#31876,#31877,#31878,#31879,#31880),.UNSPECIFIED.,.F.,.F.)
B_SPLINE_CURVE_WITH_KNOTS((6,1,1,1,1,1,1,1,1,1,1,1,1,1,1,1,1,1,1,1,1,1,
1,1,1,1,1,1,1,1,1,1,1,1,1,1,1,1,1,1,1,1,1,1,1,1,1,1,1,1,1,1,1,1,1,1,1,1,
1,1,1,1,1,1,1,6),(-1.,-0.984615384615383,-0.969230769230768,-0.953846153846152,
-0.938461538461537,-0.923076923076922,-0.907692307692306,-0.892307692307691,
-0.876923076923076,-0.86153846153846,-0.846153846153845,-0.83076923076923,
-0.815384615384614,-0.799999999999999,-0.784615384615384,-0.769230769230768,
-0.753846153846153,-0.738461538461538,-0.723076923076922,-0.707692307692307,
-0.692307692307692,-0.676923076923076,-0.661538461538461,-0.646153846153846,
-0.63076923076923,-0.615384615384615,-0.6,-0.584615384615384,-0.569230769230769,
-0.553846153846154,-0.538461538461538,-0.523076923076923,-0.507692307692308,
-0.492307692307692,-0.476923076923077,-0.461538461538462,-0.446153846153846,
-0.430769230769231,-0.415384615384615,-0.4,-0.384615384615385,-0.369230769230769,
-0.353846153846154,-0.338461538461538,-0.323076923076923,-0.307692307692308,
-0.292307692307692,-0.276923076923077,-0.261538461538462,-0.246153846153846,
-0.230769230769231,-0.215384615384615,-0.2,-0.184615384615385,-0.169230769230769,
-0.153846153846154,-0.138461538461538,-0.123076923076923,-0.107692307692308,
-0.0923076923076923,-0.0769230769230769,-0.0615384615384615,-0.0461538461538462,
-0.0307692307692308,-0.0153846153846154,0.),.UNSPECIFIED.)
CURVE()
GEOMETRIC_REPRESENTATION_ITEM()
RATIONAL_B_SPLINE_CURVE((1.,1.,1.,1.,1.,1.,1.,1.,1.,1.,1.,1.,1.,1.,1.,1.,
1.,1.,1.,1.,1.,1.,1.,1.,1.,1.,1.,1.,1.,1.,1.,1.,1.,1.,1.,1.,1.,1.,1.,1.,
1.,1.,1.,1.,1.,1.,1.,1.,1.,1.,1.,1.,1.,1.,1.,1.,1.,1.,1.,1.,1.,1.,1.,1.,
1.,1.,1.,1.,1.,1.))
REPRESENTATION_ITEM('')
);
#226=(
BOUNDED_CURVE()
B_SPLINE_CURVE(5,(#32027,#32028,#32029,#32030,#32031,#32032,#32033,#32034,
#32035,#32036,#32037,#32038,#32039,#32040,#32041,#32042,#32043,#32044,#32045,
#32046,#32047,#32048,#32049,#32050,#32051,#32052,#32053,#32054,#32055,#32056,
#32057,#32058,#32059,#32060,#32061,#32062,#32063,#32064,#32065,#32066,#32067,
#32068,#32069,#32070,#32071,#32072,#32073,#32074,#32075,#32076,#32077,#32078,
#32079,#32080,#32081,#32082,#32083,#32084,#32085,#32086,#32087,#32088,#32089,
#32090,#32091,#32092,#32093,#32094,#32095,#32096),.UNSPECIFIED.,.F.,.F.)
B_SPLINE_CURVE_WITH_KNOTS((6,1,1,1,1,1,1,1,1,1,1,1,1,1,1,1,1,1,1,1,1,1,
1,1,1,1,1,1,1,1,1,1,1,1,1,1,1,1,1,1,1,1,1,1,1,1,1,1,1,1,1,1,1,1,1,1,1,1,
1,1,1,1,1,1,1,6),(-1.,-0.984615384615383,-0.969230769230768,-0.953846153846152,
-0.938461538461537,-0.923076923076922,-0.907692307692306,-0.892307692307691,
-0.876923076923076,-0.86153846153846,-0.846153846153845,-0.83076923076923,
-0.815384615384614,-0.799999999999999,-0.784615384615384,-0.769230769230768,
-0.753846153846153,-0.738461538461538,-0.723076923076922,-0.707692307692307,
-0.692307692307692,-0.676923076923076,-0.661538461538461,-0.646153846153846,
-0.63076923076923,-0.615384615384615,-0.6,-0.584615384615384,-0.569230769230769,
-0.553846153846154,-0.538461538461538,-0.523076923076923,-0.507692307692308,
-0.492307692307692,-0.476923076923077,-0.461538461538462,-0.446153846153846,
-0.430769230769231,-0.415384615384615,-0.4,-0.384615384615385,-0.369230769230769,
-0.353846153846154,-0.338461538461538,-0.323076923076923,-0.307692307692308,
-0.292307692307692,-0.276923076923077,-0.261538461538462,-0.246153846153846,
-0.230769230769231,-0.215384615384615,-0.2,-0.184615384615385,-0.169230769230769,
-0.153846153846154,-0.138461538461538,-0.123076923076923,-0.107692307692308,
-0.0923076923076923,-0.0769230769230769,-0.0615384615384615,-0.0461538461538462,
-0.0307692307692308,-0.0153846153846154,0.),.UNSPECIFIED.)
CURVE()
GEOMETRIC_REPRESENTATION_ITEM()
RATIONAL_B_SPLINE_CURVE((1.,1.,1.,1.,1.,1.,1.,1.,1.,1.,1.,1.,1.,1.,1.,1.,
1.,1.,1.,1.,1.,1.,1.,1.,1.,1.,1.,1.,1.,1.,1.,1.,1.,1.,1.,1.,1.,1.,1.,1.,
1.,1.,1.,1.,1.,1.,1.,1.,1.,1.,1.,1.,1.,1.,1.,1.,1.,1.,1.,1.,1.,1.,1.,1.,
1.,1.,1.,1.,1.,1.))
REPRESENTATION_ITEM('')
);
#227=(
BOUNDED_CURVE()
B_SPLINE_CURVE(5,(#32243,#32244,#32245,#32246,#32247,#32248,#32249,#32250,
#32251,#32252,#32253,#32254,#32255,#32256,#32257,#32258,#32259,#32260,#32261,
#32262,#32263,#32264,#32265,#32266,#32267,#32268,#32269,#32270,#32271,#32272,
#32273,#32274,#32275,#32276,#32277,#32278,#32279,#32280,#32281,#32282,#32283,
#32284,#32285,#32286,#32287,#32288,#32289,#32290,#32291,#32292,#32293,#32294,
#32295,#32296,#32297,#32298,#32299,#32300,#32301,#32302,#32303,#32304,#32305,
#32306,#32307,#32308,#32309,#32310,#32311,#32312),.UNSPECIFIED.,.F.,.F.)
B_SPLINE_CURVE_WITH_KNOTS((6,1,1,1,1,1,1,1,1,1,1,1,1,1,1,1,1,1,1,1,1,1,
1,1,1,1,1,1,1,1,1,1,1,1,1,1,1,1,1,1,1,1,1,1,1,1,1,1,1,1,1,1,1,1,1,1,1,1,
1,1,1,1,1,1,1,6),(-1.,-0.984615384615383,-0.969230769230768,-0.953846153846152,
-0.938461538461537,-0.923076923076922,-0.907692307692306,-0.892307692307691,
-0.876923076923076,-0.86153846153846,-0.846153846153845,-0.83076923076923,
-0.815384615384614,-0.799999999999999,-0.784615384615384,-0.769230769230768,
-0.753846153846153,-0.738461538461538,-0.723076923076922,-0.707692307692307,
-0.692307692307692,-0.676923076923076,-0.661538461538461,-0.646153846153846,
-0.63076923076923,-0.615384615384615,-0.6,-0.584615384615384,-0.569230769230769,
-0.553846153846154,-0.538461538461538,-0.523076923076923,-0.507692307692308,
-0.492307692307692,-0.476923076923077,-0.461538461538462,-0.446153846153846,
-0.430769230769231,-0.415384615384615,-0.4,-0.384615384615385,-0.369230769230769,
-0.353846153846154,-0.338461538461538,-0.323076923076923,-0.307692307692308,
-0.292307692307692,-0.276923076923077,-0.261538461538462,-0.246153846153846,
-0.230769230769231,-0.215384615384615,-0.2,-0.184615384615385,-0.169230769230769,
-0.153846153846154,-0.138461538461538,-0.123076923076923,-0.107692307692308,
-0.0923076923076923,-0.0769230769230769,-0.0615384615384615,-0.0461538461538462,
-0.0307692307692308,-0.0153846153846154,0.),.UNSPECIFIED.)
CURVE()
GEOMETRIC_REPRESENTATION_ITEM()
RATIONAL_B_SPLINE_CURVE((1.,1.,1.,1.,1.,1.,1.,1.,1.,1.,1.,1.,1.,1.,1.,1.,
1.,1.,1.,1.,1.,1.,1.,1.,1.,1.,1.,1.,1.,1.,1.,1.,1.,1.,1.,1.,1.,1.,1.,1.,
1.,1.,1.,1.,1.,1.,1.,1.,1.,1.,1.,1.,1.,1.,1.,1.,1.,1.,1.,1.,1.,1.,1.,1.,
1.,1.,1.,1.,1.,1.))
REPRESENTATION_ITEM('')
);
#228=(
BOUNDED_CURVE()
B_SPLINE_CURVE(5,(#32459,#32460,#32461,#32462,#32463,#32464,#32465,#32466,
#32467,#32468,#32469,#32470,#32471,#32472,#32473,#32474,#32475,#32476,#32477,
#32478,#32479,#32480,#32481,#32482,#32483,#32484,#32485,#32486,#32487,#32488,
#32489,#32490,#32491,#32492,#32493,#32494,#32495,#32496,#32497,#32498,#32499,
#32500,#32501,#32502,#32503,#32504,#32505,#32506,#32507,#32508,#32509,#32510,
#32511,#32512,#32513,#32514,#32515,#32516,#32517,#32518,#32519,#32520,#32521,
#32522,#32523,#32524,#32525,#32526,#32527,#32528),.UNSPECIFIED.,.F.,.F.)
B_SPLINE_CURVE_WITH_KNOTS((6,1,1,1,1,1,1,1,1,1,1,1,1,1,1,1,1,1,1,1,1,1,
1,1,1,1,1,1,1,1,1,1,1,1,1,1,1,1,1,1,1,1,1,1,1,1,1,1,1,1,1,1,1,1,1,1,1,1,
1,1,1,1,1,1,1,6),(-1.,-0.984615384615383,-0.969230769230768,-0.953846153846152,
-0.938461538461537,-0.923076923076922,-0.907692307692306,-0.892307692307691,
-0.876923076923076,-0.86153846153846,-0.846153846153845,-0.83076923076923,
-0.815384615384614,-0.799999999999999,-0.784615384615384,-0.769230769230768,
-0.753846153846153,-0.738461538461538,-0.723076923076922,-0.707692307692307,
-0.692307692307692,-0.676923076923076,-0.661538461538461,-0.646153846153846,
-0.63076923076923,-0.615384615384615,-0.6,-0.584615384615384,-0.569230769230769,
-0.553846153846154,-0.538461538461538,-0.523076923076923,-0.507692307692308,
-0.492307692307692,-0.476923076923077,-0.461538461538462,-0.446153846153846,
-0.430769230769231,-0.415384615384615,-0.4,-0.384615384615385,-0.369230769230769,
-0.353846153846154,-0.338461538461538,-0.323076923076923,-0.307692307692308,
-0.292307692307692,-0.276923076923077,-0.261538461538462,-0.246153846153846,
-0.230769230769231,-0.215384615384615,-0.2,-0.184615384615385,-0.169230769230769,
-0.153846153846154,-0.138461538461538,-0.123076923076923,-0.107692307692308,
-0.0923076923076923,-0.0769230769230769,-0.0615384615384615,-0.0461538461538462,
-0.0307692307692308,-0.0153846153846154,0.),.UNSPECIFIED.)
CURVE()
GEOMETRIC_REPRESENTATION_ITEM()
RATIONAL_B_SPLINE_CURVE((1.,1.,1.,1.,1.,1.,1.,1.,1.,1.,1.,1.,1.,1.,1.,1.,
1.,1.,1.,1.,1.,1.,1.,1.,1.,1.,1.,1.,1.,1.,1.,1.,1.,1.,1.,1.,1.,1.,1.,1.,
1.,1.,1.,1.,1.,1.,1.,1.,1.,1.,1.,1.,1.,1.,1.,1.,1.,1.,1.,1.,1.,1.,1.,1.,
1.,1.,1.,1.,1.,1.))
REPRESENTATION_ITEM('')
);
#229=(
BOUNDED_CURVE()
B_SPLINE_CURVE(5,(#32675,#32676,#32677,#32678,#32679,#32680,#32681,#32682,
#32683,#32684,#32685,#32686,#32687,#32688,#32689,#32690,#32691,#32692,#32693,
#32694,#32695,#32696,#32697,#32698,#32699,#32700,#32701,#32702,#32703,#32704,
#32705,#32706,#32707,#32708,#32709,#32710,#32711,#32712,#32713,#32714,#32715,
#32716,#32717,#32718,#32719,#32720,#32721,#32722,#32723,#32724,#32725,#32726,
#32727,#32728,#32729,#32730,#32731,#32732,#32733,#32734,#32735,#32736,#32737,
#32738,#32739,#32740,#32741,#32742,#32743,#32744),.UNSPECIFIED.,.F.,.F.)
B_SPLINE_CURVE_WITH_KNOTS((6,1,1,1,1,1,1,1,1,1,1,1,1,1,1,1,1,1,1,1,1,1,
1,1,1,1,1,1,1,1,1,1,1,1,1,1,1,1,1,1,1,1,1,1,1,1,1,1,1,1,1,1,1,1,1,1,1,1,
1,1,1,1,1,1,1,6),(-1.,-0.984615384615383,-0.969230769230768,-0.953846153846152,
-0.938461538461537,-0.923076923076922,-0.907692307692306,-0.892307692307691,
-0.876923076923076,-0.86153846153846,-0.846153846153845,-0.83076923076923,
-0.815384615384614,-0.799999999999999,-0.784615384615384,-0.769230769230768,
-0.753846153846153,-0.738461538461538,-0.723076923076922,-0.707692307692307,
-0.692307692307692,-0.676923076923076,-0.661538461538461,-0.646153846153846,
-0.63076923076923,-0.615384615384615,-0.6,-0.584615384615384,-0.569230769230769,
-0.553846153846154,-0.538461538461538,-0.523076923076923,-0.507692307692308,
-0.492307692307692,-0.476923076923077,-0.461538461538462,-0.446153846153846,
-0.430769230769231,-0.415384615384615,-0.4,-0.384615384615385,-0.369230769230769,
-0.353846153846154,-0.338461538461538,-0.323076923076923,-0.307692307692308,
-0.292307692307692,-0.276923076923077,-0.261538461538462,-0.246153846153846,
-0.230769230769231,-0.215384615384615,-0.2,-0.184615384615385,-0.169230769230769,
-0.153846153846154,-0.138461538461538,-0.123076923076923,-0.107692307692308,
-0.0923076923076923,-0.0769230769230769,-0.0615384615384615,-0.0461538461538462,
-0.0307692307692308,-0.0153846153846154,0.),.UNSPECIFIED.)
CURVE()
GEOMETRIC_REPRESENTATION_ITEM()
RATIONAL_B_SPLINE_CURVE((1.,1.,1.,1.,1.,1.,1.,1.,1.,1.,1.,1.,1.,1.,1.,1.,
1.,1.,1.,1.,1.,1.,1.,1.,1.,1.,1.,1.,1.,1.,1.,1.,1.,1.,1.,1.,1.,1.,1.,1.,
1.,1.,1.,1.,1.,1.,1.,1.,1.,1.,1.,1.,1.,1.,1.,1.,1.,1.,1.,1.,1.,1.,1.,1.,
1.,1.,1.,1.,1.,1.))
REPRESENTATION_ITEM('')
);
#230=(
BOUNDED_CURVE()
B_SPLINE_CURVE(5,(#32891,#32892,#32893,#32894,#32895,#32896,#32897,#32898,
#32899,#32900,#32901,#32902,#32903,#32904,#32905,#32906,#32907,#32908,#32909,
#32910,#32911,#32912,#32913,#32914,#32915,#32916,#32917,#32918,#32919,#32920,
#32921,#32922,#32923,#32924,#32925,#32926,#32927,#32928,#32929,#32930,#32931,
#32932,#32933,#32934,#32935,#32936,#32937,#32938,#32939,#32940,#32941,#32942,
#32943,#32944,#32945,#32946,#32947,#32948,#32949,#32950,#32951,#32952,#32953,
#32954,#32955,#32956,#32957,#32958,#32959,#32960),.UNSPECIFIED.,.F.,.F.)
B_SPLINE_CURVE_WITH_KNOTS((6,1,1,1,1,1,1,1,1,1,1,1,1,1,1,1,1,1,1,1,1,1,
1,1,1,1,1,1,1,1,1,1,1,1,1,1,1,1,1,1,1,1,1,1,1,1,1,1,1,1,1,1,1,1,1,1,1,1,
1,1,1,1,1,1,1,6),(-1.,-0.984615384615383,-0.969230769230768,-0.953846153846152,
-0.938461538461537,-0.923076923076922,-0.907692307692306,-0.892307692307691,
-0.876923076923076,-0.86153846153846,-0.846153846153845,-0.83076923076923,
-0.815384615384614,-0.799999999999999,-0.784615384615384,-0.769230769230768,
-0.753846153846153,-0.738461538461538,-0.723076923076922,-0.707692307692307,
-0.692307692307692,-0.676923076923076,-0.661538461538461,-0.646153846153846,
-0.63076923076923,-0.615384615384615,-0.6,-0.584615384615384,-0.569230769230769,
-0.553846153846154,-0.538461538461538,-0.523076923076923,-0.507692307692308,
-0.492307692307692,-0.476923076923077,-0.461538461538462,-0.446153846153846,
-0.430769230769231,-0.415384615384615,-0.4,-0.384615384615385,-0.369230769230769,
-0.353846153846154,-0.338461538461538,-0.323076923076923,-0.307692307692308,
-0.292307692307692,-0.276923076923077,-0.261538461538462,-0.246153846153846,
-0.230769230769231,-0.215384615384615,-0.2,-0.184615384615385,-0.169230769230769,
-0.153846153846154,-0.138461538461538,-0.123076923076923,-0.107692307692308,
-0.0923076923076923,-0.0769230769230769,-0.0615384615384615,-0.0461538461538462,
-0.0307692307692308,-0.0153846153846154,0.),.UNSPECIFIED.)
CURVE()
GEOMETRIC_REPRESENTATION_ITEM()
RATIONAL_B_SPLINE_CURVE((1.,1.,1.,1.,1.,1.,1.,1.,1.,1.,1.,1.,1.,1.,1.,1.,
1.,1.,1.,1.,1.,1.,1.,1.,1.,1.,1.,1.,1.,1.,1.,1.,1.,1.,1.,1.,1.,1.,1.,1.,
1.,1.,1.,1.,1.,1.,1.,1.,1.,1.,1.,1.,1.,1.,1.,1.,1.,1.,1.,1.,1.,1.,1.,1.,
1.,1.,1.,1.,1.,1.))
REPRESENTATION_ITEM('')
);
#231=(
BOUNDED_CURVE()
B_SPLINE_CURVE(5,(#33107,#33108,#33109,#33110,#33111,#33112,#33113,#33114,
#33115,#33116,#33117,#33118,#33119,#33120,#33121,#33122,#33123,#33124,#33125,
#33126,#33127,#33128,#33129,#33130,#33131,#33132,#33133,#33134,#33135,#33136,
#33137,#33138,#33139,#33140,#33141,#33142,#33143,#33144,#33145,#33146,#33147,
#33148,#33149,#33150,#33151,#33152,#33153,#33154,#33155,#33156,#33157,#33158,
#33159,#33160,#33161,#33162,#33163,#33164,#33165,#33166,#33167,#33168,#33169,
#33170,#33171,#33172,#33173,#33174,#33175,#33176),.UNSPECIFIED.,.F.,.F.)
B_SPLINE_CURVE_WITH_KNOTS((6,1,1,1,1,1,1,1,1,1,1,1,1,1,1,1,1,1,1,1,1,1,
1,1,1,1,1,1,1,1,1,1,1,1,1,1,1,1,1,1,1,1,1,1,1,1,1,1,1,1,1,1,1,1,1,1,1,1,
1,1,1,1,1,1,1,6),(-1.,-0.984615384615383,-0.969230769230768,-0.953846153846152,
-0.938461538461537,-0.923076923076922,-0.907692307692306,-0.892307692307691,
-0.876923076923076,-0.86153846153846,-0.846153846153845,-0.83076923076923,
-0.815384615384614,-0.799999999999999,-0.784615384615384,-0.769230769230768,
-0.753846153846153,-0.738461538461538,-0.723076923076922,-0.707692307692307,
-0.692307692307692,-0.676923076923076,-0.661538461538461,-0.646153846153846,
-0.63076923076923,-0.615384615384615,-0.6,-0.584615384615384,-0.569230769230769,
-0.553846153846154,-0.538461538461538,-0.523076923076923,-0.507692307692308,
-0.492307692307692,-0.476923076923077,-0.461538461538462,-0.446153846153846,
-0.430769230769231,-0.415384615384615,-0.4,-0.384615384615385,-0.369230769230769,
-0.353846153846154,-0.338461538461538,-0.323076923076923,-0.307692307692308,
-0.292307692307692,-0.276923076923077,-0.261538461538462,-0.246153846153846,
-0.230769230769231,-0.215384615384615,-0.2,-0.184615384615385,-0.169230769230769,
-0.153846153846154,-0.138461538461538,-0.123076923076923,-0.107692307692308,
-0.0923076923076923,-0.0769230769230769,-0.0615384615384615,-0.0461538461538462,
-0.0307692307692308,-0.0153846153846154,0.),.UNSPECIFIED.)
CURVE()
GEOMETRIC_REPRESENTATION_ITEM()
RATIONAL_B_SPLINE_CURVE((1.,1.,1.,1.,1.,1.,1.,1.,1.,1.,1.,1.,1.,1.,1.,1.,
1.,1.,1.,1.,1.,1.,1.,1.,1.,1.,1.,1.,1.,1.,1.,1.,1.,1.,1.,1.,1.,1.,1.,1.,
1.,1.,1.,1.,1.,1.,1.,1.,1.,1.,1.,1.,1.,1.,1.,1.,1.,1.,1.,1.,1.,1.,1.,1.,
1.,1.,1.,1.,1.,1.))
REPRESENTATION_ITEM('')
);
#232=(
BOUNDED_CURVE()
B_SPLINE_CURVE(5,(#33323,#33324,#33325,#33326,#33327,#33328,#33329,#33330,
#33331,#33332,#33333,#33334,#33335,#33336,#33337,#33338,#33339,#33340,#33341,
#33342,#33343,#33344,#33345,#33346,#33347,#33348,#33349,#33350,#33351,#33352,
#33353,#33354,#33355,#33356,#33357,#33358,#33359,#33360,#33361,#33362,#33363,
#33364,#33365,#33366,#33367,#33368,#33369,#33370,#33371,#33372,#33373,#33374,
#33375,#33376,#33377,#33378,#33379,#33380,#33381,#33382,#33383,#33384,#33385,
#33386,#33387,#33388,#33389,#33390,#33391,#33392),.UNSPECIFIED.,.F.,.F.)
B_SPLINE_CURVE_WITH_KNOTS((6,1,1,1,1,1,1,1,1,1,1,1,1,1,1,1,1,1,1,1,1,1,
1,1,1,1,1,1,1,1,1,1,1,1,1,1,1,1,1,1,1,1,1,1,1,1,1,1,1,1,1,1,1,1,1,1,1,1,
1,1,1,1,1,1,1,6),(-1.,-0.984615384615383,-0.969230769230768,-0.953846153846152,
-0.938461538461537,-0.923076923076922,-0.907692307692306,-0.892307692307691,
-0.876923076923076,-0.86153846153846,-0.846153846153845,-0.83076923076923,
-0.815384615384614,-0.799999999999999,-0.784615384615384,-0.769230769230768,
-0.753846153846153,-0.738461538461538,-0.723076923076922,-0.707692307692307,
-0.692307692307692,-0.676923076923076,-0.661538461538461,-0.646153846153846,
-0.63076923076923,-0.615384615384615,-0.6,-0.584615384615384,-0.569230769230769,
-0.553846153846154,-0.538461538461538,-0.523076923076923,-0.507692307692308,
-0.492307692307692,-0.476923076923077,-0.461538461538462,-0.446153846153846,
-0.430769230769231,-0.415384615384615,-0.4,-0.384615384615385,-0.369230769230769,
-0.353846153846154,-0.338461538461538,-0.323076923076923,-0.307692307692308,
-0.292307692307692,-0.276923076923077,-0.261538461538462,-0.246153846153846,
-0.230769230769231,-0.215384615384615,-0.2,-0.184615384615385,-0.169230769230769,
-0.153846153846154,-0.138461538461538,-0.123076923076923,-0.107692307692308,
-0.0923076923076923,-0.0769230769230769,-0.0615384615384615,-0.0461538461538462,
-0.0307692307692308,-0.0153846153846154,0.),.UNSPECIFIED.)
CURVE()
GEOMETRIC_REPRESENTATION_ITEM()
RATIONAL_B_SPLINE_CURVE((1.,1.,1.,1.,1.,1.,1.,1.,1.,1.,1.,1.,1.,1.,1.,1.,
1.,1.,1.,1.,1.,1.,1.,1.,1.,1.,1.,1.,1.,1.,1.,1.,1.,1.,1.,1.,1.,1.,1.,1.,
1.,1.,1.,1.,1.,1.,1.,1.,1.,1.,1.,1.,1.,1.,1.,1.,1.,1.,1.,1.,1.,1.,1.,1.,
1.,1.,1.,1.,1.,1.))
REPRESENTATION_ITEM('')
);
#233=(
BOUNDED_CURVE()
B_SPLINE_CURVE(5,(#33539,#33540,#33541,#33542,#33543,#33544,#33545,#33546,
#33547,#33548,#33549,#33550,#33551,#33552,#33553,#33554,#33555,#33556,#33557,
#33558,#33559,#33560,#33561,#33562,#33563,#33564,#33565,#33566,#33567,#33568,
#33569,#33570,#33571,#33572,#33573,#33574,#33575,#33576,#33577,#33578,#33579,
#33580,#33581,#33582,#33583,#33584,#33585,#33586,#33587,#33588,#33589,#33590,
#33591,#33592,#33593,#33594,#33595,#33596,#33597,#33598,#33599,#33600,#33601,
#33602,#33603,#33604,#33605,#33606,#33607,#33608),.UNSPECIFIED.,.F.,.F.)
B_SPLINE_CURVE_WITH_KNOTS((6,1,1,1,1,1,1,1,1,1,1,1,1,1,1,1,1,1,1,1,1,1,
1,1,1,1,1,1,1,1,1,1,1,1,1,1,1,1,1,1,1,1,1,1,1,1,1,1,1,1,1,1,1,1,1,1,1,1,
1,1,1,1,1,1,1,6),(-1.,-0.984615384615383,-0.969230769230768,-0.953846153846152,
-0.938461538461537,-0.923076923076922,-0.907692307692306,-0.892307692307691,
-0.876923076923076,-0.86153846153846,-0.846153846153845,-0.83076923076923,
-0.815384615384614,-0.799999999999999,-0.784615384615384,-0.769230769230768,
-0.753846153846153,-0.738461538461538,-0.723076923076922,-0.707692307692307,
-0.692307692307692,-0.676923076923076,-0.661538461538461,-0.646153846153846,
-0.63076923076923,-0.615384615384615,-0.6,-0.584615384615384,-0.569230769230769,
-0.553846153846154,-0.538461538461538,-0.523076923076923,-0.507692307692308,
-0.492307692307692,-0.476923076923077,-0.461538461538462,-0.446153846153846,
-0.430769230769231,-0.415384615384615,-0.4,-0.384615384615385,-0.369230769230769,
-0.353846153846154,-0.338461538461538,-0.323076923076923,-0.307692307692308,
-0.292307692307692,-0.276923076923077,-0.261538461538462,-0.246153846153846,
-0.230769230769231,-0.215384615384615,-0.2,-0.184615384615385,-0.169230769230769,
-0.153846153846154,-0.138461538461538,-0.123076923076923,-0.107692307692308,
-0.0923076923076923,-0.0769230769230769,-0.0615384615384615,-0.0461538461538462,
-0.0307692307692308,-0.0153846153846154,0.),.UNSPECIFIED.)
CURVE()
GEOMETRIC_REPRESENTATION_ITEM()
RATIONAL_B_SPLINE_CURVE((1.,1.,1.,1.,1.,1.,1.,1.,1.,1.,1.,1.,1.,1.,1.,1.,
1.,1.,1.,1.,1.,1.,1.,1.,1.,1.,1.,1.,1.,1.,1.,1.,1.,1.,1.,1.,1.,1.,1.,1.,
1.,1.,1.,1.,1.,1.,1.,1.,1.,1.,1.,1.,1.,1.,1.,1.,1.,1.,1.,1.,1.,1.,1.,1.,
1.,1.,1.,1.,1.,1.))
REPRESENTATION_ITEM('')
);
#234=(
BOUNDED_CURVE()
B_SPLINE_CURVE(5,(#33755,#33756,#33757,#33758,#33759,#33760,#33761,#33762,
#33763,#33764,#33765,#33766,#33767,#33768,#33769,#33770,#33771,#33772,#33773,
#33774,#33775,#33776,#33777,#33778,#33779,#33780,#33781,#33782,#33783,#33784,
#33785,#33786,#33787,#33788,#33789,#33790,#33791,#33792,#33793,#33794,#33795,
#33796,#33797,#33798,#33799,#33800,#33801,#33802,#33803,#33804,#33805,#33806,
#33807,#33808,#33809,#33810,#33811,#33812,#33813,#33814,#33815,#33816,#33817,
#33818,#33819,#33820,#33821,#33822,#33823,#33824),.UNSPECIFIED.,.F.,.F.)
B_SPLINE_CURVE_WITH_KNOTS((6,1,1,1,1,1,1,1,1,1,1,1,1,1,1,1,1,1,1,1,1,1,
1,1,1,1,1,1,1,1,1,1,1,1,1,1,1,1,1,1,1,1,1,1,1,1,1,1,1,1,1,1,1,1,1,1,1,1,
1,1,1,1,1,1,1,6),(-1.,-0.984615384615383,-0.969230769230768,-0.953846153846152,
-0.938461538461537,-0.923076923076922,-0.907692307692306,-0.892307692307691,
-0.876923076923076,-0.86153846153846,-0.846153846153845,-0.83076923076923,
-0.815384615384614,-0.799999999999999,-0.784615384615384,-0.769230769230768,
-0.753846153846153,-0.738461538461538,-0.723076923076922,-0.707692307692307,
-0.692307692307692,-0.676923076923076,-0.661538461538461,-0.646153846153846,
-0.63076923076923,-0.615384615384615,-0.6,-0.584615384615384,-0.569230769230769,
-0.553846153846154,-0.538461538461538,-0.523076923076923,-0.507692307692308,
-0.492307692307692,-0.476923076923077,-0.461538461538462,-0.446153846153846,
-0.430769230769231,-0.415384615384615,-0.4,-0.384615384615385,-0.369230769230769,
-0.353846153846154,-0.338461538461538,-0.323076923076923,-0.307692307692308,
-0.292307692307692,-0.276923076923077,-0.261538461538462,-0.246153846153846,
-0.230769230769231,-0.215384615384615,-0.2,-0.184615384615385,-0.169230769230769,
-0.153846153846154,-0.138461538461538,-0.123076923076923,-0.107692307692308,
-0.0923076923076923,-0.0769230769230769,-0.0615384615384615,-0.0461538461538462,
-0.0307692307692308,-0.0153846153846154,0.),.UNSPECIFIED.)
CURVE()
GEOMETRIC_REPRESENTATION_ITEM()
RATIONAL_B_SPLINE_CURVE((1.,1.,1.,1.,1.,1.,1.,1.,1.,1.,1.,1.,1.,1.,1.,1.,
1.,1.,1.,1.,1.,1.,1.,1.,1.,1.,1.,1.,1.,1.,1.,1.,1.,1.,1.,1.,1.,1.,1.,1.,
1.,1.,1.,1.,1.,1.,1.,1.,1.,1.,1.,1.,1.,1.,1.,1.,1.,1.,1.,1.,1.,1.,1.,1.,
1.,1.,1.,1.,1.,1.))
REPRESENTATION_ITEM('')
);
#235=(
BOUNDED_CURVE()
B_SPLINE_CURVE(5,(#33971,#33972,#33973,#33974,#33975,#33976,#33977,#33978,
#33979,#33980,#33981,#33982,#33983,#33984,#33985,#33986,#33987,#33988,#33989,
#33990,#33991,#33992,#33993,#33994,#33995,#33996,#33997,#33998,#33999,#34000,
#34001,#34002,#34003,#34004,#34005,#34006,#34007,#34008,#34009,#34010,#34011,
#34012,#34013,#34014,#34015,#34016,#34017,#34018,#34019,#34020,#34021,#34022,
#34023,#34024,#34025,#34026,#34027,#34028,#34029,#34030,#34031,#34032,#34033,
#34034,#34035,#34036,#34037,#34038,#34039,#34040),.UNSPECIFIED.,.F.,.F.)
B_SPLINE_CURVE_WITH_KNOTS((6,1,1,1,1,1,1,1,1,1,1,1,1,1,1,1,1,1,1,1,1,1,
1,1,1,1,1,1,1,1,1,1,1,1,1,1,1,1,1,1,1,1,1,1,1,1,1,1,1,1,1,1,1,1,1,1,1,1,
1,1,1,1,1,1,1,6),(-1.,-0.984615384615383,-0.969230769230768,-0.953846153846152,
-0.938461538461537,-0.923076923076922,-0.907692307692306,-0.892307692307691,
-0.876923076923076,-0.86153846153846,-0.846153846153845,-0.83076923076923,
-0.815384615384614,-0.799999999999999,-0.784615384615384,-0.769230769230768,
-0.753846153846153,-0.738461538461538,-0.723076923076922,-0.707692307692307,
-0.692307692307692,-0.676923076923076,-0.661538461538461,-0.646153846153846,
-0.63076923076923,-0.615384615384615,-0.6,-0.584615384615384,-0.569230769230769,
-0.553846153846154,-0.538461538461538,-0.523076923076923,-0.507692307692308,
-0.492307692307692,-0.476923076923077,-0.461538461538462,-0.446153846153846,
-0.430769230769231,-0.415384615384615,-0.4,-0.384615384615385,-0.369230769230769,
-0.353846153846154,-0.338461538461538,-0.323076923076923,-0.307692307692308,
-0.292307692307692,-0.276923076923077,-0.261538461538462,-0.246153846153846,
-0.230769230769231,-0.215384615384615,-0.2,-0.184615384615385,-0.169230769230769,
-0.153846153846154,-0.138461538461538,-0.123076923076923,-0.107692307692308,
-0.0923076923076923,-0.0769230769230769,-0.0615384615384615,-0.0461538461538462,
-0.0307692307692308,-0.0153846153846154,0.),.UNSPECIFIED.)
CURVE()
GEOMETRIC_REPRESENTATION_ITEM()
RATIONAL_B_SPLINE_CURVE((1.,1.,1.,1.,1.,1.,1.,1.,1.,1.,1.,1.,1.,1.,1.,1.,
1.,1.,1.,1.,1.,1.,1.,1.,1.,1.,1.,1.,1.,1.,1.,1.,1.,1.,1.,1.,1.,1.,1.,1.,
1.,1.,1.,1.,1.,1.,1.,1.,1.,1.,1.,1.,1.,1.,1.,1.,1.,1.,1.,1.,1.,1.,1.,1.,
1.,1.,1.,1.,1.,1.))
REPRESENTATION_ITEM('')
);
#236=(
BOUNDED_CURVE()
B_SPLINE_CURVE(5,(#34187,#34188,#34189,#34190,#34191,#34192,#34193,#34194,
#34195,#34196,#34197,#34198,#34199,#34200,#34201,#34202,#34203,#34204,#34205,
#34206,#34207,#34208,#34209,#34210,#34211,#34212,#34213,#34214,#34215,#34216,
#34217,#34218,#34219,#34220,#34221,#34222,#34223,#34224,#34225,#34226,#34227,
#34228,#34229,#34230,#34231,#34232,#34233,#34234,#34235,#34236,#34237,#34238,
#34239,#34240,#34241,#34242,#34243,#34244,#34245,#34246,#34247,#34248,#34249,
#34250,#34251,#34252,#34253,#34254,#34255,#34256),.UNSPECIFIED.,.F.,.F.)
B_SPLINE_CURVE_WITH_KNOTS((6,1,1,1,1,1,1,1,1,1,1,1,1,1,1,1,1,1,1,1,1,1,
1,1,1,1,1,1,1,1,1,1,1,1,1,1,1,1,1,1,1,1,1,1,1,1,1,1,1,1,1,1,1,1,1,1,1,1,
1,1,1,1,1,1,1,6),(-1.,-0.984615384615383,-0.969230769230768,-0.953846153846152,
-0.938461538461537,-0.923076923076922,-0.907692307692306,-0.892307692307691,
-0.876923076923076,-0.86153846153846,-0.846153846153845,-0.83076923076923,
-0.815384615384614,-0.799999999999999,-0.784615384615384,-0.769230769230768,
-0.753846153846153,-0.738461538461538,-0.723076923076922,-0.707692307692307,
-0.692307692307692,-0.676923076923076,-0.661538461538461,-0.646153846153846,
-0.63076923076923,-0.615384615384615,-0.6,-0.584615384615384,-0.569230769230769,
-0.553846153846154,-0.538461538461538,-0.523076923076923,-0.507692307692308,
-0.492307692307692,-0.476923076923077,-0.461538461538462,-0.446153846153846,
-0.430769230769231,-0.415384615384615,-0.4,-0.384615384615385,-0.369230769230769,
-0.353846153846154,-0.338461538461538,-0.323076923076923,-0.307692307692308,
-0.292307692307692,-0.276923076923077,-0.261538461538462,-0.246153846153846,
-0.230769230769231,-0.215384615384615,-0.2,-0.184615384615385,-0.169230769230769,
-0.153846153846154,-0.138461538461538,-0.123076923076923,-0.107692307692308,
-0.0923076923076923,-0.0769230769230769,-0.0615384615384615,-0.0461538461538462,
-0.0307692307692308,-0.0153846153846154,0.),.UNSPECIFIED.)
CURVE()
GEOMETRIC_REPRESENTATION_ITEM()
RATIONAL_B_SPLINE_CURVE((1.,1.,1.,1.,1.,1.,1.,1.,1.,1.,1.,1.,1.,1.,1.,1.,
1.,1.,1.,1.,1.,1.,1.,1.,1.,1.,1.,1.,1.,1.,1.,1.,1.,1.,1.,1.,1.,1.,1.,1.,
1.,1.,1.,1.,1.,1.,1.,1.,1.,1.,1.,1.,1.,1.,1.,1.,1.,1.,1.,1.,1.,1.,1.,1.,
1.,1.,1.,1.,1.,1.))
REPRESENTATION_ITEM('')
);
#237=(
BOUNDED_CURVE()
B_SPLINE_CURVE(5,(#34403,#34404,#34405,#34406,#34407,#34408,#34409,#34410,
#34411,#34412,#34413,#34414,#34415,#34416,#34417,#34418,#34419,#34420,#34421,
#34422,#34423,#34424,#34425,#34426,#34427,#34428,#34429,#34430,#34431,#34432,
#34433,#34434,#34435,#34436,#34437,#34438,#34439,#34440,#34441,#34442,#34443,
#34444,#34445,#34446,#34447,#34448,#34449,#34450,#34451,#34452,#34453,#34454,
#34455,#34456,#34457,#34458,#34459,#34460,#34461,#34462,#34463,#34464,#34465,
#34466,#34467,#34468,#34469,#34470,#34471,#34472),.UNSPECIFIED.,.F.,.F.)
B_SPLINE_CURVE_WITH_KNOTS((6,1,1,1,1,1,1,1,1,1,1,1,1,1,1,1,1,1,1,1,1,1,
1,1,1,1,1,1,1,1,1,1,1,1,1,1,1,1,1,1,1,1,1,1,1,1,1,1,1,1,1,1,1,1,1,1,1,1,
1,1,1,1,1,1,1,6),(-1.,-0.984615384615383,-0.969230769230768,-0.953846153846152,
-0.938461538461537,-0.923076923076922,-0.907692307692306,-0.892307692307691,
-0.876923076923076,-0.86153846153846,-0.846153846153845,-0.83076923076923,
-0.815384615384614,-0.799999999999999,-0.784615384615384,-0.769230769230768,
-0.753846153846153,-0.738461538461538,-0.723076923076922,-0.707692307692307,
-0.692307692307692,-0.676923076923076,-0.661538461538461,-0.646153846153846,
-0.63076923076923,-0.615384615384615,-0.6,-0.584615384615384,-0.569230769230769,
-0.553846153846154,-0.538461538461538,-0.523076923076923,-0.507692307692308,
-0.492307692307692,-0.476923076923077,-0.461538461538462,-0.446153846153846,
-0.430769230769231,-0.415384615384615,-0.4,-0.384615384615385,-0.369230769230769,
-0.353846153846154,-0.338461538461538,-0.323076923076923,-0.307692307692308,
-0.292307692307692,-0.276923076923077,-0.261538461538462,-0.246153846153846,
-0.230769230769231,-0.215384615384615,-0.2,-0.184615384615385,-0.169230769230769,
-0.153846153846154,-0.138461538461538,-0.123076923076923,-0.107692307692308,
-0.0923076923076923,-0.0769230769230769,-0.0615384615384615,-0.0461538461538462,
-0.0307692307692308,-0.0153846153846154,0.),.UNSPECIFIED.)
CURVE()
GEOMETRIC_REPRESENTATION_ITEM()
RATIONAL_B_SPLINE_CURVE((1.,1.,1.,1.,1.,1.,1.,1.,1.,1.,1.,1.,1.,1.,1.,1.,
1.,1.,1.,1.,1.,1.,1.,1.,1.,1.,1.,1.,1.,1.,1.,1.,1.,1.,1.,1.,1.,1.,1.,1.,
1.,1.,1.,1.,1.,1.,1.,1.,1.,1.,1.,1.,1.,1.,1.,1.,1.,1.,1.,1.,1.,1.,1.,1.,
1.,1.,1.,1.,1.,1.))
REPRESENTATION_ITEM('')
);
#238=(
BOUNDED_CURVE()
B_SPLINE_CURVE(5,(#34619,#34620,#34621,#34622,#34623,#34624,#34625,#34626,
#34627,#34628,#34629,#34630,#34631,#34632,#34633,#34634,#34635,#34636,#34637,
#34638,#34639,#34640,#34641,#34642,#34643,#34644,#34645,#34646,#34647,#34648,
#34649,#34650,#34651,#34652,#34653,#34654,#34655,#34656,#34657,#34658,#34659,
#34660,#34661,#34662,#34663,#34664,#34665,#34666,#34667,#34668,#34669,#34670,
#34671,#34672,#34673,#34674,#34675,#34676,#34677,#34678,#34679,#34680,#34681,
#34682,#34683,#34684,#34685,#34686,#34687,#34688),.UNSPECIFIED.,.F.,.F.)
B_SPLINE_CURVE_WITH_KNOTS((6,1,1,1,1,1,1,1,1,1,1,1,1,1,1,1,1,1,1,1,1,1,
1,1,1,1,1,1,1,1,1,1,1,1,1,1,1,1,1,1,1,1,1,1,1,1,1,1,1,1,1,1,1,1,1,1,1,1,
1,1,1,1,1,1,1,6),(-1.,-0.984615384615383,-0.969230769230768,-0.953846153846152,
-0.938461538461537,-0.923076923076922,-0.907692307692306,-0.892307692307691,
-0.876923076923076,-0.86153846153846,-0.846153846153845,-0.83076923076923,
-0.815384615384614,-0.799999999999999,-0.784615384615384,-0.769230769230768,
-0.753846153846153,-0.738461538461538,-0.723076923076922,-0.707692307692307,
-0.692307692307692,-0.676923076923076,-0.661538461538461,-0.646153846153846,
-0.63076923076923,-0.615384615384615,-0.6,-0.584615384615384,-0.569230769230769,
-0.553846153846154,-0.538461538461538,-0.523076923076923,-0.507692307692308,
-0.492307692307692,-0.476923076923077,-0.461538461538462,-0.446153846153846,
-0.430769230769231,-0.415384615384615,-0.4,-0.384615384615385,-0.369230769230769,
-0.353846153846154,-0.338461538461538,-0.323076923076923,-0.307692307692308,
-0.292307692307692,-0.276923076923077,-0.261538461538462,-0.246153846153846,
-0.230769230769231,-0.215384615384615,-0.2,-0.184615384615385,-0.169230769230769,
-0.153846153846154,-0.138461538461538,-0.123076923076923,-0.107692307692308,
-0.0923076923076923,-0.0769230769230769,-0.0615384615384615,-0.0461538461538462,
-0.0307692307692308,-0.0153846153846154,0.),.UNSPECIFIED.)
CURVE()
GEOMETRIC_REPRESENTATION_ITEM()
RATIONAL_B_SPLINE_CURVE((1.,1.,1.,1.,1.,1.,1.,1.,1.,1.,1.,1.,1.,1.,1.,1.,
1.,1.,1.,1.,1.,1.,1.,1.,1.,1.,1.,1.,1.,1.,1.,1.,1.,1.,1.,1.,1.,1.,1.,1.,
1.,1.,1.,1.,1.,1.,1.,1.,1.,1.,1.,1.,1.,1.,1.,1.,1.,1.,1.,1.,1.,1.,1.,1.,
1.,1.,1.,1.,1.,1.))
REPRESENTATION_ITEM('')
);
#239=(
BOUNDED_CURVE()
B_SPLINE_CURVE(5,(#34835,#34836,#34837,#34838,#34839,#34840,#34841,#34842,
#34843,#34844,#34845,#34846,#34847,#34848,#34849,#34850,#34851,#34852,#34853,
#34854,#34855,#34856,#34857,#34858,#34859,#34860,#34861,#34862,#34863,#34864,
#34865,#34866,#34867,#34868,#34869,#34870,#34871,#34872,#34873,#34874,#34875,
#34876,#34877,#34878,#34879,#34880,#34881,#34882,#34883,#34884,#34885,#34886,
#34887,#34888,#34889,#34890,#34891,#34892,#34893,#34894,#34895,#34896,#34897,
#34898,#34899,#34900,#34901,#34902,#34903,#34904),.UNSPECIFIED.,.F.,.F.)
B_SPLINE_CURVE_WITH_KNOTS((6,1,1,1,1,1,1,1,1,1,1,1,1,1,1,1,1,1,1,1,1,1,
1,1,1,1,1,1,1,1,1,1,1,1,1,1,1,1,1,1,1,1,1,1,1,1,1,1,1,1,1,1,1,1,1,1,1,1,
1,1,1,1,1,1,1,6),(-1.,-0.984615384615383,-0.969230769230768,-0.953846153846152,
-0.938461538461537,-0.923076923076922,-0.907692307692306,-0.892307692307691,
-0.876923076923076,-0.86153846153846,-0.846153846153845,-0.83076923076923,
-0.815384615384614,-0.799999999999999,-0.784615384615384,-0.769230769230768,
-0.753846153846153,-0.738461538461538,-0.723076923076922,-0.707692307692307,
-0.692307692307692,-0.676923076923076,-0.661538461538461,-0.646153846153846,
-0.63076923076923,-0.615384615384615,-0.6,-0.584615384615384,-0.569230769230769,
-0.553846153846154,-0.538461538461538,-0.523076923076923,-0.507692307692308,
-0.492307692307692,-0.476923076923077,-0.461538461538462,-0.446153846153846,
-0.430769230769231,-0.415384615384615,-0.4,-0.384615384615385,-0.369230769230769,
-0.353846153846154,-0.338461538461538,-0.323076923076923,-0.307692307692308,
-0.292307692307692,-0.276923076923077,-0.261538461538462,-0.246153846153846,
-0.230769230769231,-0.215384615384615,-0.2,-0.184615384615385,-0.169230769230769,
-0.153846153846154,-0.138461538461538,-0.123076923076923,-0.107692307692308,
-0.0923076923076923,-0.0769230769230769,-0.0615384615384615,-0.0461538461538462,
-0.0307692307692308,-0.0153846153846154,0.),.UNSPECIFIED.)
CURVE()
GEOMETRIC_REPRESENTATION_ITEM()
RATIONAL_B_SPLINE_CURVE((1.,1.,1.,1.,1.,1.,1.,1.,1.,1.,1.,1.,1.,1.,1.,1.,
1.,1.,1.,1.,1.,1.,1.,1.,1.,1.,1.,1.,1.,1.,1.,1.,1.,1.,1.,1.,1.,1.,1.,1.,
1.,1.,1.,1.,1.,1.,1.,1.,1.,1.,1.,1.,1.,1.,1.,1.,1.,1.,1.,1.,1.,1.,1.,1.,
1.,1.,1.,1.,1.,1.))
REPRESENTATION_ITEM('')
);
#240=(
BOUNDED_CURVE()
B_SPLINE_CURVE(5,(#35051,#35052,#35053,#35054,#35055,#35056,#35057,#35058,
#35059,#35060,#35061,#35062,#35063,#35064,#35065,#35066,#35067,#35068,#35069,
#35070,#35071,#35072,#35073,#35074,#35075,#35076,#35077,#35078,#35079,#35080,
#35081,#35082,#35083,#35084,#35085,#35086,#35087,#35088,#35089,#35090,#35091,
#35092,#35093,#35094,#35095,#35096,#35097,#35098,#35099,#35100,#35101,#35102,
#35103,#35104,#35105,#35106,#35107,#35108,#35109,#35110,#35111,#35112,#35113,
#35114,#35115,#35116,#35117,#35118,#35119,#35120),.UNSPECIFIED.,.F.,.F.)
B_SPLINE_CURVE_WITH_KNOTS((6,1,1,1,1,1,1,1,1,1,1,1,1,1,1,1,1,1,1,1,1,1,
1,1,1,1,1,1,1,1,1,1,1,1,1,1,1,1,1,1,1,1,1,1,1,1,1,1,1,1,1,1,1,1,1,1,1,1,
1,1,1,1,1,1,1,6),(-1.,-0.984615384615383,-0.969230769230768,-0.953846153846152,
-0.938461538461537,-0.923076923076922,-0.907692307692306,-0.892307692307691,
-0.876923076923076,-0.86153846153846,-0.846153846153845,-0.83076923076923,
-0.815384615384614,-0.799999999999999,-0.784615384615384,-0.769230769230768,
-0.753846153846153,-0.738461538461538,-0.723076923076922,-0.707692307692307,
-0.692307692307692,-0.676923076923076,-0.661538461538461,-0.646153846153846,
-0.63076923076923,-0.615384615384615,-0.6,-0.584615384615384,-0.569230769230769,
-0.553846153846154,-0.538461538461538,-0.523076923076923,-0.507692307692308,
-0.492307692307692,-0.476923076923077,-0.461538461538462,-0.446153846153846,
-0.430769230769231,-0.415384615384615,-0.4,-0.384615384615385,-0.369230769230769,
-0.353846153846154,-0.338461538461538,-0.323076923076923,-0.307692307692308,
-0.292307692307692,-0.276923076923077,-0.261538461538462,-0.246153846153846,
-0.230769230769231,-0.215384615384615,-0.2,-0.184615384615385,-0.169230769230769,
-0.153846153846154,-0.138461538461538,-0.123076923076923,-0.107692307692308,
-0.0923076923076923,-0.0769230769230769,-0.0615384615384615,-0.0461538461538462,
-0.0307692307692308,-0.0153846153846154,0.),.UNSPECIFIED.)
CURVE()
GEOMETRIC_REPRESENTATION_ITEM()
RATIONAL_B_SPLINE_CURVE((1.,1.,1.,1.,1.,1.,1.,1.,1.,1.,1.,1.,1.,1.,1.,1.,
1.,1.,1.,1.,1.,1.,1.,1.,1.,1.,1.,1.,1.,1.,1.,1.,1.,1.,1.,1.,1.,1.,1.,1.,
1.,1.,1.,1.,1.,1.,1.,1.,1.,1.,1.,1.,1.,1.,1.,1.,1.,1.,1.,1.,1.,1.,1.,1.,
1.,1.,1.,1.,1.,1.))
REPRESENTATION_ITEM('')
);
#241=(
BOUNDED_CURVE()
B_SPLINE_CURVE(5,(#35267,#35268,#35269,#35270,#35271,#35272,#35273,#35274,
#35275,#35276,#35277,#35278,#35279,#35280,#35281,#35282,#35283,#35284,#35285,
#35286,#35287,#35288,#35289,#35290,#35291,#35292,#35293,#35294,#35295,#35296,
#35297,#35298,#35299,#35300,#35301,#35302,#35303,#35304,#35305,#35306,#35307,
#35308,#35309,#35310,#35311,#35312,#35313,#35314,#35315,#35316,#35317,#35318,
#35319,#35320,#35321,#35322,#35323,#35324,#35325,#35326,#35327,#35328,#35329,
#35330,#35331,#35332,#35333,#35334,#35335,#35336),.UNSPECIFIED.,.F.,.F.)
B_SPLINE_CURVE_WITH_KNOTS((6,1,1,1,1,1,1,1,1,1,1,1,1,1,1,1,1,1,1,1,1,1,
1,1,1,1,1,1,1,1,1,1,1,1,1,1,1,1,1,1,1,1,1,1,1,1,1,1,1,1,1,1,1,1,1,1,1,1,
1,1,1,1,1,1,1,6),(-1.,-0.984615384615383,-0.969230769230768,-0.953846153846152,
-0.938461538461537,-0.923076923076922,-0.907692307692306,-0.892307692307691,
-0.876923076923076,-0.86153846153846,-0.846153846153845,-0.83076923076923,
-0.815384615384614,-0.799999999999999,-0.784615384615384,-0.769230769230768,
-0.753846153846153,-0.738461538461538,-0.723076923076922,-0.707692307692307,
-0.692307692307692,-0.676923076923076,-0.661538461538461,-0.646153846153846,
-0.63076923076923,-0.615384615384615,-0.6,-0.584615384615384,-0.569230769230769,
-0.553846153846154,-0.538461538461538,-0.523076923076923,-0.507692307692308,
-0.492307692307692,-0.476923076923077,-0.461538461538462,-0.446153846153846,
-0.430769230769231,-0.415384615384615,-0.4,-0.384615384615385,-0.369230769230769,
-0.353846153846154,-0.338461538461538,-0.323076923076923,-0.307692307692308,
-0.292307692307692,-0.276923076923077,-0.261538461538462,-0.246153846153846,
-0.230769230769231,-0.215384615384615,-0.2,-0.184615384615385,-0.169230769230769,
-0.153846153846154,-0.138461538461538,-0.123076923076923,-0.107692307692308,
-0.0923076923076923,-0.0769230769230769,-0.0615384615384615,-0.0461538461538462,
-0.0307692307692308,-0.0153846153846154,0.),.UNSPECIFIED.)
CURVE()
GEOMETRIC_REPRESENTATION_ITEM()
RATIONAL_B_SPLINE_CURVE((1.,1.,1.,1.,1.,1.,1.,1.,1.,1.,1.,1.,1.,1.,1.,1.,
1.,1.,1.,1.,1.,1.,1.,1.,1.,1.,1.,1.,1.,1.,1.,1.,1.,1.,1.,1.,1.,1.,1.,1.,
1.,1.,1.,1.,1.,1.,1.,1.,1.,1.,1.,1.,1.,1.,1.,1.,1.,1.,1.,1.,1.,1.,1.,1.,
1.,1.,1.,1.,1.,1.))
REPRESENTATION_ITEM('')
);
#242=(
BOUNDED_CURVE()
B_SPLINE_CURVE(5,(#35483,#35484,#35485,#35486,#35487,#35488,#35489,#35490,
#35491,#35492,#35493,#35494,#35495,#35496,#35497,#35498,#35499,#35500,#35501,
#35502,#35503,#35504,#35505,#35506,#35507,#35508,#35509,#35510,#35511,#35512,
#35513,#35514,#35515,#35516,#35517,#35518,#35519,#35520,#35521,#35522,#35523,
#35524,#35525,#35526,#35527,#35528,#35529,#35530,#35531,#35532,#35533,#35534,
#35535,#35536,#35537,#35538,#35539,#35540,#35541,#35542,#35543,#35544,#35545,
#35546,#35547,#35548,#35549,#35550,#35551,#35552),.UNSPECIFIED.,.F.,.F.)
B_SPLINE_CURVE_WITH_KNOTS((6,1,1,1,1,1,1,1,1,1,1,1,1,1,1,1,1,1,1,1,1,1,
1,1,1,1,1,1,1,1,1,1,1,1,1,1,1,1,1,1,1,1,1,1,1,1,1,1,1,1,1,1,1,1,1,1,1,1,
1,1,1,1,1,1,1,6),(-1.,-0.984615384615383,-0.969230769230768,-0.953846153846152,
-0.938461538461537,-0.923076923076922,-0.907692307692306,-0.892307692307691,
-0.876923076923076,-0.86153846153846,-0.846153846153845,-0.83076923076923,
-0.815384615384614,-0.799999999999999,-0.784615384615384,-0.769230769230768,
-0.753846153846153,-0.738461538461538,-0.723076923076922,-0.707692307692307,
-0.692307692307692,-0.676923076923076,-0.661538461538461,-0.646153846153846,
-0.63076923076923,-0.615384615384615,-0.6,-0.584615384615384,-0.569230769230769,
-0.553846153846154,-0.538461538461538,-0.523076923076923,-0.507692307692308,
-0.492307692307692,-0.476923076923077,-0.461538461538462,-0.446153846153846,
-0.430769230769231,-0.415384615384615,-0.4,-0.384615384615385,-0.369230769230769,
-0.353846153846154,-0.338461538461538,-0.323076923076923,-0.307692307692308,
-0.292307692307692,-0.276923076923077,-0.261538461538462,-0.246153846153846,
-0.230769230769231,-0.215384615384615,-0.2,-0.184615384615385,-0.169230769230769,
-0.153846153846154,-0.138461538461538,-0.123076923076923,-0.107692307692308,
-0.0923076923076923,-0.0769230769230769,-0.0615384615384615,-0.0461538461538462,
-0.0307692307692308,-0.0153846153846154,0.),.UNSPECIFIED.)
CURVE()
GEOMETRIC_REPRESENTATION_ITEM()
RATIONAL_B_SPLINE_CURVE((1.,1.,1.,1.,1.,1.,1.,1.,1.,1.,1.,1.,1.,1.,1.,1.,
1.,1.,1.,1.,1.,1.,1.,1.,1.,1.,1.,1.,1.,1.,1.,1.,1.,1.,1.,1.,1.,1.,1.,1.,
1.,1.,1.,1.,1.,1.,1.,1.,1.,1.,1.,1.,1.,1.,1.,1.,1.,1.,1.,1.,1.,1.,1.,1.,
1.,1.,1.,1.,1.,1.))
REPRESENTATION_ITEM('')
);
#243=(
BOUNDED_CURVE()
B_SPLINE_CURVE(5,(#35699,#35700,#35701,#35702,#35703,#35704,#35705,#35706,
#35707,#35708,#35709,#35710,#35711,#35712,#35713,#35714,#35715,#35716,#35717,
#35718,#35719,#35720,#35721,#35722,#35723,#35724,#35725,#35726,#35727,#35728,
#35729,#35730,#35731,#35732,#35733,#35734,#35735,#35736,#35737,#35738,#35739,
#35740,#35741,#35742,#35743,#35744,#35745,#35746,#35747,#35748,#35749,#35750,
#35751,#35752,#35753,#35754,#35755,#35756,#35757,#35758,#35759,#35760,#35761,
#35762,#35763,#35764,#35765,#35766,#35767,#35768),.UNSPECIFIED.,.F.,.F.)
B_SPLINE_CURVE_WITH_KNOTS((6,1,1,1,1,1,1,1,1,1,1,1,1,1,1,1,1,1,1,1,1,1,
1,1,1,1,1,1,1,1,1,1,1,1,1,1,1,1,1,1,1,1,1,1,1,1,1,1,1,1,1,1,1,1,1,1,1,1,
1,1,1,1,1,1,1,6),(-1.,-0.984615384615383,-0.969230769230768,-0.953846153846152,
-0.938461538461537,-0.923076923076922,-0.907692307692306,-0.892307692307691,
-0.876923076923076,-0.86153846153846,-0.846153846153845,-0.83076923076923,
-0.815384615384614,-0.799999999999999,-0.784615384615384,-0.769230769230768,
-0.753846153846153,-0.738461538461538,-0.723076923076922,-0.707692307692307,
-0.692307692307692,-0.676923076923076,-0.661538461538461,-0.646153846153846,
-0.63076923076923,-0.615384615384615,-0.6,-0.584615384615384,-0.569230769230769,
-0.553846153846154,-0.538461538461538,-0.523076923076923,-0.507692307692308,
-0.492307692307692,-0.476923076923077,-0.461538461538462,-0.446153846153846,
-0.430769230769231,-0.415384615384615,-0.4,-0.384615384615385,-0.369230769230769,
-0.353846153846154,-0.338461538461538,-0.323076923076923,-0.307692307692308,
-0.292307692307692,-0.276923076923077,-0.261538461538462,-0.246153846153846,
-0.230769230769231,-0.215384615384615,-0.2,-0.184615384615385,-0.169230769230769,
-0.153846153846154,-0.138461538461538,-0.123076923076923,-0.107692307692308,
-0.0923076923076923,-0.0769230769230769,-0.0615384615384615,-0.0461538461538462,
-0.0307692307692308,-0.0153846153846154,0.),.UNSPECIFIED.)
CURVE()
GEOMETRIC_REPRESENTATION_ITEM()
RATIONAL_B_SPLINE_CURVE((1.,1.,1.,1.,1.,1.,1.,1.,1.,1.,1.,1.,1.,1.,1.,1.,
1.,1.,1.,1.,1.,1.,1.,1.,1.,1.,1.,1.,1.,1.,1.,1.,1.,1.,1.,1.,1.,1.,1.,1.,
1.,1.,1.,1.,1.,1.,1.,1.,1.,1.,1.,1.,1.,1.,1.,1.,1.,1.,1.,1.,1.,1.,1.,1.,
1.,1.,1.,1.,1.,1.))
REPRESENTATION_ITEM('')
);
#244=(
BOUNDED_CURVE()
B_SPLINE_CURVE(5,(#35915,#35916,#35917,#35918,#35919,#35920,#35921,#35922,
#35923,#35924,#35925,#35926,#35927,#35928,#35929,#35930,#35931,#35932,#35933,
#35934,#35935,#35936,#35937,#35938,#35939,#35940,#35941,#35942,#35943,#35944,
#35945,#35946,#35947,#35948,#35949,#35950,#35951,#35952,#35953,#35954,#35955,
#35956,#35957,#35958,#35959,#35960,#35961,#35962,#35963,#35964,#35965,#35966,
#35967,#35968,#35969,#35970,#35971,#35972,#35973,#35974,#35975,#35976,#35977,
#35978,#35979,#35980,#35981,#35982,#35983,#35984),.UNSPECIFIED.,.F.,.F.)
B_SPLINE_CURVE_WITH_KNOTS((6,1,1,1,1,1,1,1,1,1,1,1,1,1,1,1,1,1,1,1,1,1,
1,1,1,1,1,1,1,1,1,1,1,1,1,1,1,1,1,1,1,1,1,1,1,1,1,1,1,1,1,1,1,1,1,1,1,1,
1,1,1,1,1,1,1,6),(-1.,-0.984615384615383,-0.969230769230768,-0.953846153846152,
-0.938461538461537,-0.923076923076922,-0.907692307692306,-0.892307692307691,
-0.876923076923076,-0.86153846153846,-0.846153846153845,-0.83076923076923,
-0.815384615384614,-0.799999999999999,-0.784615384615384,-0.769230769230768,
-0.753846153846153,-0.738461538461538,-0.723076923076922,-0.707692307692307,
-0.692307692307692,-0.676923076923076,-0.661538461538461,-0.646153846153846,
-0.63076923076923,-0.615384615384615,-0.6,-0.584615384615384,-0.569230769230769,
-0.553846153846154,-0.538461538461538,-0.523076923076923,-0.507692307692308,
-0.492307692307692,-0.476923076923077,-0.461538461538462,-0.446153846153846,
-0.430769230769231,-0.415384615384615,-0.4,-0.384615384615385,-0.369230769230769,
-0.353846153846154,-0.338461538461538,-0.323076923076923,-0.307692307692308,
-0.292307692307692,-0.276923076923077,-0.261538461538462,-0.246153846153846,
-0.230769230769231,-0.215384615384615,-0.2,-0.184615384615385,-0.169230769230769,
-0.153846153846154,-0.138461538461538,-0.123076923076923,-0.107692307692308,
-0.0923076923076923,-0.0769230769230769,-0.0615384615384615,-0.0461538461538462,
-0.0307692307692308,-0.0153846153846154,0.),.UNSPECIFIED.)
CURVE()
GEOMETRIC_REPRESENTATION_ITEM()
RATIONAL_B_SPLINE_CURVE((1.,1.,1.,1.,1.,1.,1.,1.,1.,1.,1.,1.,1.,1.,1.,1.,
1.,1.,1.,1.,1.,1.,1.,1.,1.,1.,1.,1.,1.,1.,1.,1.,1.,1.,1.,1.,1.,1.,1.,1.,
1.,1.,1.,1.,1.,1.,1.,1.,1.,1.,1.,1.,1.,1.,1.,1.,1.,1.,1.,1.,1.,1.,1.,1.,
1.,1.,1.,1.,1.,1.))
REPRESENTATION_ITEM('')
);
#245=(
BOUNDED_CURVE()
B_SPLINE_CURVE(5,(#36131,#36132,#36133,#36134,#36135,#36136,#36137,#36138,
#36139,#36140,#36141,#36142,#36143,#36144,#36145,#36146,#36147,#36148,#36149,
#36150,#36151,#36152,#36153,#36154,#36155,#36156,#36157,#36158,#36159,#36160,
#36161,#36162,#36163,#36164,#36165,#36166,#36167,#36168,#36169,#36170,#36171,
#36172,#36173,#36174,#36175,#36176,#36177,#36178,#36179,#36180,#36181,#36182,
#36183,#36184,#36185,#36186,#36187,#36188,#36189,#36190,#36191,#36192,#36193,
#36194,#36195,#36196,#36197,#36198,#36199,#36200),.UNSPECIFIED.,.F.,.F.)
B_SPLINE_CURVE_WITH_KNOTS((6,1,1,1,1,1,1,1,1,1,1,1,1,1,1,1,1,1,1,1,1,1,
1,1,1,1,1,1,1,1,1,1,1,1,1,1,1,1,1,1,1,1,1,1,1,1,1,1,1,1,1,1,1,1,1,1,1,1,
1,1,1,1,1,1,1,6),(-1.,-0.984615384615383,-0.969230769230768,-0.953846153846152,
-0.938461538461537,-0.923076923076922,-0.907692307692306,-0.892307692307691,
-0.876923076923076,-0.86153846153846,-0.846153846153845,-0.83076923076923,
-0.815384615384614,-0.799999999999999,-0.784615384615384,-0.769230769230768,
-0.753846153846153,-0.738461538461538,-0.723076923076922,-0.707692307692307,
-0.692307692307692,-0.676923076923076,-0.661538461538461,-0.646153846153846,
-0.63076923076923,-0.615384615384615,-0.6,-0.584615384615384,-0.569230769230769,
-0.553846153846154,-0.538461538461538,-0.523076923076923,-0.507692307692308,
-0.492307692307692,-0.476923076923077,-0.461538461538462,-0.446153846153846,
-0.430769230769231,-0.415384615384615,-0.4,-0.384615384615385,-0.369230769230769,
-0.353846153846154,-0.338461538461538,-0.323076923076923,-0.307692307692308,
-0.292307692307692,-0.276923076923077,-0.261538461538462,-0.246153846153846,
-0.230769230769231,-0.215384615384615,-0.2,-0.184615384615385,-0.169230769230769,
-0.153846153846154,-0.138461538461538,-0.123076923076923,-0.107692307692308,
-0.0923076923076923,-0.0769230769230769,-0.0615384615384615,-0.0461538461538462,
-0.0307692307692308,-0.0153846153846154,0.),.UNSPECIFIED.)
CURVE()
GEOMETRIC_REPRESENTATION_ITEM()
RATIONAL_B_SPLINE_CURVE((1.,1.,1.,1.,1.,1.,1.,1.,1.,1.,1.,1.,1.,1.,1.,1.,
1.,1.,1.,1.,1.,1.,1.,1.,1.,1.,1.,1.,1.,1.,1.,1.,1.,1.,1.,1.,1.,1.,1.,1.,
1.,1.,1.,1.,1.,1.,1.,1.,1.,1.,1.,1.,1.,1.,1.,1.,1.,1.,1.,1.,1.,1.,1.,1.,
1.,1.,1.,1.,1.,1.))
REPRESENTATION_ITEM('')
);
#246=(
BOUNDED_CURVE()
B_SPLINE_CURVE(5,(#36347,#36348,#36349,#36350,#36351,#36352,#36353,#36354,
#36355,#36356,#36357,#36358,#36359,#36360,#36361,#36362,#36363,#36364,#36365,
#36366,#36367,#36368,#36369,#36370,#36371,#36372,#36373,#36374,#36375,#36376,
#36377,#36378,#36379,#36380,#36381,#36382,#36383,#36384,#36385,#36386,#36387,
#36388,#36389,#36390,#36391,#36392,#36393,#36394,#36395,#36396,#36397,#36398,
#36399,#36400,#36401,#36402,#36403,#36404,#36405,#36406,#36407,#36408,#36409,
#36410,#36411,#36412,#36413,#36414,#36415,#36416),.UNSPECIFIED.,.F.,.F.)
B_SPLINE_CURVE_WITH_KNOTS((6,1,1,1,1,1,1,1,1,1,1,1,1,1,1,1,1,1,1,1,1,1,
1,1,1,1,1,1,1,1,1,1,1,1,1,1,1,1,1,1,1,1,1,1,1,1,1,1,1,1,1,1,1,1,1,1,1,1,
1,1,1,1,1,1,1,6),(-1.,-0.984615384615383,-0.969230769230768,-0.953846153846152,
-0.938461538461537,-0.923076923076922,-0.907692307692306,-0.892307692307691,
-0.876923076923076,-0.86153846153846,-0.846153846153845,-0.83076923076923,
-0.815384615384614,-0.799999999999999,-0.784615384615384,-0.769230769230768,
-0.753846153846153,-0.738461538461538,-0.723076923076922,-0.707692307692307,
-0.692307692307692,-0.676923076923076,-0.661538461538461,-0.646153846153846,
-0.63076923076923,-0.615384615384615,-0.6,-0.584615384615384,-0.569230769230769,
-0.553846153846154,-0.538461538461538,-0.523076923076923,-0.507692307692308,
-0.492307692307692,-0.476923076923077,-0.461538461538462,-0.446153846153846,
-0.430769230769231,-0.415384615384615,-0.4,-0.384615384615385,-0.369230769230769,
-0.353846153846154,-0.338461538461538,-0.323076923076923,-0.307692307692308,
-0.292307692307692,-0.276923076923077,-0.261538461538462,-0.246153846153846,
-0.230769230769231,-0.215384615384615,-0.2,-0.184615384615385,-0.169230769230769,
-0.153846153846154,-0.138461538461538,-0.123076923076923,-0.107692307692308,
-0.0923076923076923,-0.0769230769230769,-0.0615384615384615,-0.0461538461538462,
-0.0307692307692308,-0.0153846153846154,0.),.UNSPECIFIED.)
CURVE()
GEOMETRIC_REPRESENTATION_ITEM()
RATIONAL_B_SPLINE_CURVE((1.,1.,1.,1.,1.,1.,1.,1.,1.,1.,1.,1.,1.,1.,1.,1.,
1.,1.,1.,1.,1.,1.,1.,1.,1.,1.,1.,1.,1.,1.,1.,1.,1.,1.,1.,1.,1.,1.,1.,1.,
1.,1.,1.,1.,1.,1.,1.,1.,1.,1.,1.,1.,1.,1.,1.,1.,1.,1.,1.,1.,1.,1.,1.,1.,
1.,1.,1.,1.,1.,1.))
REPRESENTATION_ITEM('')
);
#247=(
BOUNDED_CURVE()
B_SPLINE_CURVE(5,(#36563,#36564,#36565,#36566,#36567,#36568,#36569,#36570,
#36571,#36572,#36573,#36574,#36575,#36576,#36577,#36578,#36579,#36580,#36581,
#36582,#36583,#36584,#36585,#36586,#36587,#36588,#36589,#36590,#36591,#36592,
#36593,#36594,#36595,#36596,#36597,#36598,#36599,#36600,#36601,#36602,#36603,
#36604,#36605,#36606,#36607,#36608,#36609,#36610,#36611,#36612,#36613,#36614,
#36615,#36616,#36617,#36618,#36619,#36620,#36621,#36622,#36623,#36624,#36625,
#36626,#36627,#36628,#36629,#36630,#36631,#36632),.UNSPECIFIED.,.F.,.F.)
B_SPLINE_CURVE_WITH_KNOTS((6,1,1,1,1,1,1,1,1,1,1,1,1,1,1,1,1,1,1,1,1,1,
1,1,1,1,1,1,1,1,1,1,1,1,1,1,1,1,1,1,1,1,1,1,1,1,1,1,1,1,1,1,1,1,1,1,1,1,
1,1,1,1,1,1,1,6),(-1.,-0.984615384615383,-0.969230769230768,-0.953846153846152,
-0.938461538461537,-0.923076923076922,-0.907692307692306,-0.892307692307691,
-0.876923076923076,-0.86153846153846,-0.846153846153845,-0.83076923076923,
-0.815384615384614,-0.799999999999999,-0.784615384615384,-0.769230769230768,
-0.753846153846153,-0.738461538461538,-0.723076923076922,-0.707692307692307,
-0.692307692307692,-0.676923076923076,-0.661538461538461,-0.646153846153846,
-0.63076923076923,-0.615384615384615,-0.6,-0.584615384615384,-0.569230769230769,
-0.553846153846154,-0.538461538461538,-0.523076923076923,-0.507692307692308,
-0.492307692307692,-0.476923076923077,-0.461538461538462,-0.446153846153846,
-0.430769230769231,-0.415384615384615,-0.4,-0.384615384615385,-0.369230769230769,
-0.353846153846154,-0.338461538461538,-0.323076923076923,-0.307692307692308,
-0.292307692307692,-0.276923076923077,-0.261538461538462,-0.246153846153846,
-0.230769230769231,-0.215384615384615,-0.2,-0.184615384615385,-0.169230769230769,
-0.153846153846154,-0.138461538461538,-0.123076923076923,-0.107692307692308,
-0.0923076923076923,-0.0769230769230769,-0.0615384615384615,-0.0461538461538462,
-0.0307692307692308,-0.0153846153846154,0.),.UNSPECIFIED.)
CURVE()
GEOMETRIC_REPRESENTATION_ITEM()
RATIONAL_B_SPLINE_CURVE((1.,1.,1.,1.,1.,1.,1.,1.,1.,1.,1.,1.,1.,1.,1.,1.,
1.,1.,1.,1.,1.,1.,1.,1.,1.,1.,1.,1.,1.,1.,1.,1.,1.,1.,1.,1.,1.,1.,1.,1.,
1.,1.,1.,1.,1.,1.,1.,1.,1.,1.,1.,1.,1.,1.,1.,1.,1.,1.,1.,1.,1.,1.,1.,1.,
1.,1.,1.,1.,1.,1.))
REPRESENTATION_ITEM('')
);
#248=(
BOUNDED_CURVE()
B_SPLINE_CURVE(5,(#36779,#36780,#36781,#36782,#36783,#36784,#36785,#36786,
#36787,#36788,#36789,#36790,#36791,#36792,#36793,#36794,#36795,#36796,#36797,
#36798,#36799,#36800,#36801,#36802,#36803,#36804,#36805,#36806,#36807,#36808,
#36809,#36810,#36811,#36812,#36813,#36814,#36815,#36816,#36817,#36818,#36819,
#36820,#36821,#36822,#36823,#36824,#36825,#36826,#36827,#36828,#36829,#36830,
#36831,#36832,#36833,#36834,#36835,#36836,#36837,#36838,#36839,#36840,#36841,
#36842,#36843,#36844,#36845,#36846,#36847,#36848),.UNSPECIFIED.,.F.,.F.)
B_SPLINE_CURVE_WITH_KNOTS((6,1,1,1,1,1,1,1,1,1,1,1,1,1,1,1,1,1,1,1,1,1,
1,1,1,1,1,1,1,1,1,1,1,1,1,1,1,1,1,1,1,1,1,1,1,1,1,1,1,1,1,1,1,1,1,1,1,1,
1,1,1,1,1,1,1,6),(-1.,-0.984615384615383,-0.969230769230768,-0.953846153846152,
-0.938461538461537,-0.923076923076922,-0.907692307692306,-0.892307692307691,
-0.876923076923076,-0.86153846153846,-0.846153846153845,-0.83076923076923,
-0.815384615384614,-0.799999999999999,-0.784615384615384,-0.769230769230768,
-0.753846153846153,-0.738461538461538,-0.723076923076922,-0.707692307692307,
-0.692307692307692,-0.676923076923076,-0.661538461538461,-0.646153846153846,
-0.63076923076923,-0.615384615384615,-0.6,-0.584615384615384,-0.569230769230769,
-0.553846153846154,-0.538461538461538,-0.523076923076923,-0.507692307692308,
-0.492307692307692,-0.476923076923077,-0.461538461538462,-0.446153846153846,
-0.430769230769231,-0.415384615384615,-0.4,-0.384615384615385,-0.369230769230769,
-0.353846153846154,-0.338461538461538,-0.323076923076923,-0.307692307692308,
-0.292307692307692,-0.276923076923077,-0.261538461538462,-0.246153846153846,
-0.230769230769231,-0.215384615384615,-0.2,-0.184615384615385,-0.169230769230769,
-0.153846153846154,-0.138461538461538,-0.123076923076923,-0.107692307692308,
-0.0923076923076923,-0.0769230769230769,-0.0615384615384615,-0.0461538461538462,
-0.0307692307692308,-0.0153846153846154,0.),.UNSPECIFIED.)
CURVE()
GEOMETRIC_REPRESENTATION_ITEM()
RATIONAL_B_SPLINE_CURVE((1.,1.,1.,1.,1.,1.,1.,1.,1.,1.,1.,1.,1.,1.,1.,1.,
1.,1.,1.,1.,1.,1.,1.,1.,1.,1.,1.,1.,1.,1.,1.,1.,1.,1.,1.,1.,1.,1.,1.,1.,
1.,1.,1.,1.,1.,1.,1.,1.,1.,1.,1.,1.,1.,1.,1.,1.,1.,1.,1.,1.,1.,1.,1.,1.,
1.,1.,1.,1.,1.,1.))
REPRESENTATION_ITEM('')
);
#249=(
BOUNDED_CURVE()
B_SPLINE_CURVE(5,(#36995,#36996,#36997,#36998,#36999,#37000,#37001,#37002,
#37003,#37004,#37005,#37006,#37007,#37008,#37009,#37010,#37011,#37012,#37013,
#37014,#37015,#37016,#37017,#37018,#37019,#37020,#37021,#37022,#37023,#37024,
#37025,#37026,#37027,#37028,#37029,#37030,#37031,#37032,#37033,#37034,#37035,
#37036,#37037,#37038,#37039,#37040,#37041,#37042,#37043,#37044,#37045,#37046,
#37047,#37048,#37049,#37050,#37051,#37052,#37053,#37054,#37055,#37056,#37057,
#37058,#37059,#37060,#37061,#37062,#37063,#37064),.UNSPECIFIED.,.F.,.F.)
B_SPLINE_CURVE_WITH_KNOTS((6,1,1,1,1,1,1,1,1,1,1,1,1,1,1,1,1,1,1,1,1,1,
1,1,1,1,1,1,1,1,1,1,1,1,1,1,1,1,1,1,1,1,1,1,1,1,1,1,1,1,1,1,1,1,1,1,1,1,
1,1,1,1,1,1,1,6),(-1.,-0.984615384615383,-0.969230769230768,-0.953846153846152,
-0.938461538461537,-0.923076923076922,-0.907692307692306,-0.892307692307691,
-0.876923076923076,-0.86153846153846,-0.846153846153845,-0.83076923076923,
-0.815384615384614,-0.799999999999999,-0.784615384615384,-0.769230769230768,
-0.753846153846153,-0.738461538461538,-0.723076923076922,-0.707692307692307,
-0.692307692307692,-0.676923076923076,-0.661538461538461,-0.646153846153846,
-0.63076923076923,-0.615384615384615,-0.6,-0.584615384615384,-0.569230769230769,
-0.553846153846154,-0.538461538461538,-0.523076923076923,-0.507692307692308,
-0.492307692307692,-0.476923076923077,-0.461538461538462,-0.446153846153846,
-0.430769230769231,-0.415384615384615,-0.4,-0.384615384615385,-0.369230769230769,
-0.353846153846154,-0.338461538461538,-0.323076923076923,-0.307692307692308,
-0.292307692307692,-0.276923076923077,-0.261538461538462,-0.246153846153846,
-0.230769230769231,-0.215384615384615,-0.2,-0.184615384615385,-0.169230769230769,
-0.153846153846154,-0.138461538461538,-0.123076923076923,-0.107692307692308,
-0.0923076923076923,-0.0769230769230769,-0.0615384615384615,-0.0461538461538462,
-0.0307692307692308,-0.0153846153846154,0.),.UNSPECIFIED.)
CURVE()
GEOMETRIC_REPRESENTATION_ITEM()
RATIONAL_B_SPLINE_CURVE((1.,1.,1.,1.,1.,1.,1.,1.,1.,1.,1.,1.,1.,1.,1.,1.,
1.,1.,1.,1.,1.,1.,1.,1.,1.,1.,1.,1.,1.,1.,1.,1.,1.,1.,1.,1.,1.,1.,1.,1.,
1.,1.,1.,1.,1.,1.,1.,1.,1.,1.,1.,1.,1.,1.,1.,1.,1.,1.,1.,1.,1.,1.,1.,1.,
1.,1.,1.,1.,1.,1.))
REPRESENTATION_ITEM('')
);
#250=(
BOUNDED_CURVE()
B_SPLINE_CURVE(5,(#37211,#37212,#37213,#37214,#37215,#37216,#37217,#37218,
#37219,#37220,#37221,#37222,#37223,#37224,#37225,#37226,#37227,#37228,#37229,
#37230,#37231,#37232,#37233,#37234,#37235,#37236,#37237,#37238,#37239,#37240,
#37241,#37242,#37243,#37244,#37245,#37246,#37247,#37248,#37249,#37250,#37251,
#37252,#37253,#37254,#37255,#37256,#37257,#37258,#37259,#37260,#37261,#37262,
#37263,#37264,#37265,#37266,#37267,#37268,#37269,#37270,#37271,#37272,#37273,
#37274,#37275,#37276,#37277,#37278,#37279,#37280),.UNSPECIFIED.,.F.,.F.)
B_SPLINE_CURVE_WITH_KNOTS((6,1,1,1,1,1,1,1,1,1,1,1,1,1,1,1,1,1,1,1,1,1,
1,1,1,1,1,1,1,1,1,1,1,1,1,1,1,1,1,1,1,1,1,1,1,1,1,1,1,1,1,1,1,1,1,1,1,1,
1,1,1,1,1,1,1,6),(-1.,-0.984615384615383,-0.969230769230768,-0.953846153846152,
-0.938461538461537,-0.923076923076922,-0.907692307692306,-0.892307692307691,
-0.876923076923076,-0.86153846153846,-0.846153846153845,-0.83076923076923,
-0.815384615384614,-0.799999999999999,-0.784615384615384,-0.769230769230768,
-0.753846153846153,-0.738461538461538,-0.723076923076922,-0.707692307692307,
-0.692307692307692,-0.676923076923076,-0.661538461538461,-0.646153846153846,
-0.63076923076923,-0.615384615384615,-0.6,-0.584615384615384,-0.569230769230769,
-0.553846153846154,-0.538461538461538,-0.523076923076923,-0.507692307692308,
-0.492307692307692,-0.476923076923077,-0.461538461538462,-0.446153846153846,
-0.430769230769231,-0.415384615384615,-0.4,-0.384615384615385,-0.369230769230769,
-0.353846153846154,-0.338461538461538,-0.323076923076923,-0.307692307692308,
-0.292307692307692,-0.276923076923077,-0.261538461538462,-0.246153846153846,
-0.230769230769231,-0.215384615384615,-0.2,-0.184615384615385,-0.169230769230769,
-0.153846153846154,-0.138461538461538,-0.123076923076923,-0.107692307692308,
-0.0923076923076923,-0.0769230769230769,-0.0615384615384615,-0.0461538461538462,
-0.0307692307692308,-0.0153846153846154,0.),.UNSPECIFIED.)
CURVE()
GEOMETRIC_REPRESENTATION_ITEM()
RATIONAL_B_SPLINE_CURVE((1.,1.,1.,1.,1.,1.,1.,1.,1.,1.,1.,1.,1.,1.,1.,1.,
1.,1.,1.,1.,1.,1.,1.,1.,1.,1.,1.,1.,1.,1.,1.,1.,1.,1.,1.,1.,1.,1.,1.,1.,
1.,1.,1.,1.,1.,1.,1.,1.,1.,1.,1.,1.,1.,1.,1.,1.,1.,1.,1.,1.,1.,1.,1.,1.,
1.,1.,1.,1.,1.,1.))
REPRESENTATION_ITEM('')
);
#1157=SHAPE_REPRESENTATION_RELATIONSHIP('SRR','None',#73647,#1213);
#1213=ADVANCED_BREP_SHAPE_REPRESENTATION('',(#1353),#73343);
#1284=STYLED_ITEM('',(#74002),#1353);
#1353=MANIFOLD_SOLID_BREP('Body1',#16174);
#1555=FACE_BOUND('',#3552,.T.);
#1556=FACE_BOUND('',#3556,.T.);
#1557=FACE_BOUND('',#3637,.T.);
#1822=PLANE('',#17845);
#1823=PLANE('',#17846);
#1824=PLANE('',#17847);
#1825=PLANE('',#17848);
#1826=PLANE('',#17875);
#1827=PLANE('',#17876);
#1828=PLANE('',#17879);
#1829=PLANE('',#17882);
#1830=PLANE('',#17885);
#1831=PLANE('',#17888);
#1832=PLANE('',#17891);
#1833=PLANE('',#17894);
#1834=PLANE('',#17897);
#1835=PLANE('',#17900);
#1836=PLANE('',#17903);
#1837=PLANE('',#17906);
#1838=PLANE('',#17909);
#1839=PLANE('',#17912);
#1840=PLANE('',#17915);
#1841=PLANE('',#17918);
#1842=PLANE('',#17921);
#1843=PLANE('',#17924);
#1844=PLANE('',#17927);
#1845=PLANE('',#17930);
#1846=PLANE('',#17933);
#1847=PLANE('',#17934);
#2454=FACE_OUTER_BOUND('',#3548,.T.);
#2455=FACE_OUTER_BOUND('',#3549,.T.);
#2456=FACE_OUTER_BOUND('',#3550,.T.);
#2457=FACE_OUTER_BOUND('',#3551,.T.);
#2458=FACE_OUTER_BOUND('',#3553,.T.);
#2459=FACE_OUTER_BOUND('',#3554,.T.);
#2460=FACE_OUTER_BOUND('',#3555,.T.);
#2461=FACE_OUTER_BOUND('',#3557,.T.);
#2462=FACE_OUTER_BOUND('',#3558,.T.);
#2463=FACE_OUTER_BOUND('',#3559,.T.);
#2464=FACE_OUTER_BOUND('',#3560,.T.);
#2465=FACE_OUTER_BOUND('',#3561,.T.);
#2466=FACE_OUTER_BOUND('',#3562,.T.);
#2467=FACE_OUTER_BOUND('',#3563,.T.);
#2468=FACE_OUTER_BOUND('',#3564,.T.);
#2469=FACE_OUTER_BOUND('',#3565,.T.);
#2470=FACE_OUTER_BOUND('',#3566,.T.);
#2471=FACE_OUTER_BOUND('',#3567,.T.);
#2472=FACE_OUTER_BOUND('',#3568,.T.);
#2473=FACE_OUTER_BOUND('',#3569,.T.);
#2474=FACE_OUTER_BOUND('',#3570,.T.);
#2475=FACE_OUTER_BOUND('',#3571,.T.);
#2476=FACE_OUTER_BOUND('',#3572,.T.);
#2477=FACE_OUTER_BOUND('',#3573,.T.);
#2478=FACE_OUTER_BOUND('',#3574,.T.);
#2479=FACE_OUTER_BOUND('',#3575,.T.);
#2480=FACE_OUTER_BOUND('',#3576,.T.);
#2481=FACE_OUTER_BOUND('',#3577,.T.);
#2482=FACE_OUTER_BOUND('',#3578,.T.);
#2483=FACE_OUTER_BOUND('',#3579,.T.);
#2484=FACE_OUTER_BOUND('',#3580,.T.);
#2485=FACE_OUTER_BOUND('',#3581,.T.);
#2486=FACE_OUTER_BOUND('',#3582,.T.);
#2487=FACE_OUTER_BOUND('',#3583,.T.);
#2488=FACE_OUTER_BOUND('',#3584,.T.);
#2489=FACE_OUTER_BOUND('',#3585,.T.);
#2490=FACE_OUTER_BOUND('',#3586,.T.);
#2491=FACE_OUTER_BOUND('',#3587,.T.);
#2492=FACE_OUTER_BOUND('',#3588,.T.);
#2493=FACE_OUTER_BOUND('',#3589,.T.);
#2494=FACE_OUTER_BOUND('',#3590,.T.);
#2495=FACE_OUTER_BOUND('',#3591,.T.);
#2496=FACE_OUTER_BOUND('',#3592,.T.);
#2497=FACE_OUTER_BOUND('',#3593,.T.);
#2498=FACE_OUTER_BOUND('',#3594,.T.);
#2499=FACE_OUTER_BOUND('',#3595,.T.);
#2500=FACE_OUTER_BOUND('',#3596,.T.);
#2501=FACE_OUTER_BOUND('',#3597,.T.);
#2502=FACE_OUTER_BOUND('',#3598,.T.);
#2503=FACE_OUTER_BOUND('',#3599,.T.);
#2504=FACE_OUTER_BOUND('',#3600,.T.);
#2505=FACE_OUTER_BOUND('',#3601,.T.);
#2506=FACE_OUTER_BOUND('',#3602,.T.);
#2507=FACE_OUTER_BOUND('',#3603,.T.);
#2508=FACE_OUTER_BOUND('',#3604,.T.);
#2509=FACE_OUTER_BOUND('',#3605,.T.);
#2510=FACE_OUTER_BOUND('',#3606,.T.);
#2511=FACE_OUTER_BOUND('',#3607,.T.);
#2512=FACE_OUTER_BOUND('',#3608,.T.);
#2513=FACE_OUTER_BOUND('',#3609,.T.);
#2514=FACE_OUTER_BOUND('',#3610,.T.);
#2515=FACE_OUTER_BOUND('',#3611,.T.);
#2516=FACE_OUTER_BOUND('',#3612,.T.);
#2517=FACE_OUTER_BOUND('',#3613,.T.);
#2518=FACE_OUTER_BOUND('',#3614,.T.);
#2519=FACE_OUTER_BOUND('',#3615,.T.);
#2520=FACE_OUTER_BOUND('',#3616,.T.);
#2521=FACE_OUTER_BOUND('',#3617,.T.);
#2522=FACE_OUTER_BOUND('',#3618,.T.);
#2523=FACE_OUTER_BOUND('',#3619,.T.);
#2524=FACE_OUTER_BOUND('',#3620,.T.);
#2525=FACE_OUTER_BOUND('',#3621,.T.);
#2526=FACE_OUTER_BOUND('',#3622,.T.);
#2527=FACE_OUTER_BOUND('',#3623,.T.);
#2528=FACE_OUTER_BOUND('',#3624,.T.);
#2529=FACE_OUTER_BOUND('',#3625,.T.);
#2530=FACE_OUTER_BOUND('',#3626,.T.);
#2531=FACE_OUTER_BOUND('',#3627,.T.);
#2532=FACE_OUTER_BOUND('',#3628,.T.);
#2533=FACE_OUTER_BOUND('',#3629,.T.);
#2534=FACE_OUTER_BOUND('',#3630,.T.);
#2535=FACE_OUTER_BOUND('',#3631,.T.);
#2536=FACE_OUTER_BOUND('',#3632,.T.);
#2537=FACE_OUTER_BOUND('',#3633,.T.);
#2538=FACE_OUTER_BOUND('',#3634,.T.);
#2539=FACE_OUTER_BOUND('',#3635,.T.);
#2540=FACE_OUTER_BOUND('',#3636,.T.);
#2541=FACE_OUTER_BOUND('',#3638,.T.);
#3548=EDGE_LOOP('',(#12431,#12432,#12433,#12434));
#3549=EDGE_LOOP('',(#12435,#12436,#12437,#12438));
#3550=EDGE_LOOP('',(#12439,#12440,#12441,#12442));
#3551=EDGE_LOOP('',(#12443,#12444,#12445,#12446,#12447,#12448,#12449,#12450,
#12451,#12452,#12453,#12454,#12455,#12456,#12457,#12458,#12459,#12460,#12461,
#12462,#12463,#12464,#12465,#12466,#12467,#12468,#12469,#12470,#12471,#12472,
#12473,#12474,#12475,#12476,#12477,#12478,#12479,#12480,#12481,#12482,#12483,
#12484,#12485,#12486,#12487,#12488,#12489,#12490,#12491,#12492,#12493,#12494,
#12495,#12496,#12497,#12498,#12499,#12500,#12501,#12502,#12503,#12504,#12505,
#12506,#12507,#12508,#12509,#12510,#12511,#12512,#12513,#12514,#12515,#12516,
#12517,#12518,#12519,#12520,#12521,#12522));
#3552=EDGE_LOOP('',(#12523,#12524,#12525,#12526));
#3553=EDGE_LOOP('',(#12527,#12528,#12529,#12530));
#3554=EDGE_LOOP('',(#12531,#12532,#12533,#12534));
#3555=EDGE_LOOP('',(#12535));
#3556=EDGE_LOOP('',(#12536,#12537,#12538,#12539));
#3557=EDGE_LOOP('',(#12540,#12541,#12542,#12543));
#3558=EDGE_LOOP('',(#12544,#12545,#12546,#12547));
#3559=EDGE_LOOP('',(#12548,#12549,#12550,#12551));
#3560=EDGE_LOOP('',(#12552,#12553,#12554,#12555));
#3561=EDGE_LOOP('',(#12556,#12557,#12558,#12559));
#3562=EDGE_LOOP('',(#12560,#12561,#12562,#12563));
#3563=EDGE_LOOP('',(#12564,#12565,#12566,#12567));
#3564=EDGE_LOOP('',(#12568,#12569,#12570,#12571));
#3565=EDGE_LOOP('',(#12572,#12573,#12574,#12575));
#3566=EDGE_LOOP('',(#12576,#12577,#12578,#12579));
#3567=EDGE_LOOP('',(#12580,#12581,#12582,#12583));
#3568=EDGE_LOOP('',(#12584,#12585,#12586,#12587));
#3569=EDGE_LOOP('',(#12588,#12589,#12590,#12591));
#3570=EDGE_LOOP('',(#12592,#12593,#12594,#12595));
#3571=EDGE_LOOP('',(#12596,#12597,#12598,#12599));
#3572=EDGE_LOOP('',(#12600,#12601,#12602,#12603));
#3573=EDGE_LOOP('',(#12604,#12605,#12606,#12607));
#3574=EDGE_LOOP('',(#12608,#12609,#12610,#12611));
#3575=EDGE_LOOP('',(#12612,#12613,#12614,#12615));
#3576=EDGE_LOOP('',(#12616,#12617,#12618,#12619));
#3577=EDGE_LOOP('',(#12620,#12621,#12622,#12623));
#3578=EDGE_LOOP('',(#12624,#12625,#12626,#12627));
#3579=EDGE_LOOP('',(#12628,#12629,#12630,#12631));
#3580=EDGE_LOOP('',(#12632,#12633,#12634,#12635));
#3581=EDGE_LOOP('',(#12636,#12637,#12638,#12639));
#3582=EDGE_LOOP('',(#12640,#12641,#12642,#12643));
#3583=EDGE_LOOP('',(#12644,#12645,#12646,#12647));
#3584=EDGE_LOOP('',(#12648,#12649,#12650,#12651));
#3585=EDGE_LOOP('',(#12652,#12653,#12654,#12655));
#3586=EDGE_LOOP('',(#12656,#12657,#12658,#12659));
#3587=EDGE_LOOP('',(#12660,#12661,#12662,#12663));
#3588=EDGE_LOOP('',(#12664,#12665,#12666,#12667));
#3589=EDGE_LOOP('',(#12668,#12669,#12670,#12671));
#3590=EDGE_LOOP('',(#12672,#12673,#12674,#12675));
#3591=EDGE_LOOP('',(#12676,#12677,#12678,#12679));
#3592=EDGE_LOOP('',(#12680,#12681,#12682,#12683));
#3593=EDGE_LOOP('',(#12684,#12685,#12686,#12687));
#3594=EDGE_LOOP('',(#12688,#12689,#12690,#12691));
#3595=EDGE_LOOP('',(#12692,#12693,#12694,#12695));
#3596=EDGE_LOOP('',(#12696,#12697,#12698,#12699));
#3597=EDGE_LOOP('',(#12700,#12701,#12702,#12703));
#3598=EDGE_LOOP('',(#12704,#12705,#12706,#12707));
#3599=EDGE_LOOP('',(#12708,#12709,#12710,#12711));
#3600=EDGE_LOOP('',(#12712,#12713,#12714,#12715));
#3601=EDGE_LOOP('',(#12716,#12717,#12718,#12719));
#3602=EDGE_LOOP('',(#12720,#12721,#12722,#12723));
#3603=EDGE_LOOP('',(#12724,#12725,#12726,#12727));
#3604=EDGE_LOOP('',(#12728,#12729,#12730,#12731));
#3605=EDGE_LOOP('',(#12732,#12733,#12734,#12735));
#3606=EDGE_LOOP('',(#12736,#12737,#12738,#12739));
#3607=EDGE_LOOP('',(#12740,#12741,#12742,#12743));
#3608=EDGE_LOOP('',(#12744,#12745,#12746,#12747));
#3609=EDGE_LOOP('',(#12748,#12749,#12750,#12751));
#3610=EDGE_LOOP('',(#12752,#12753,#12754,#12755));
#3611=EDGE_LOOP('',(#12756,#12757,#12758,#12759));
#3612=EDGE_LOOP('',(#12760,#12761,#12762,#12763));
#3613=EDGE_LOOP('',(#12764,#12765,#12766,#12767));
#3614=EDGE_LOOP('',(#12768,#12769,#12770,#12771));
#3615=EDGE_LOOP('',(#12772,#12773,#12774,#12775));
#3616=EDGE_LOOP('',(#12776,#12777,#12778,#12779));
#3617=EDGE_LOOP('',(#12780,#12781,#12782,#12783));
#3618=EDGE_LOOP('',(#12784,#12785,#12786,#12787));
#3619=EDGE_LOOP('',(#12788,#12789,#12790,#12791));
#3620=EDGE_LOOP('',(#12792,#12793,#12794,#12795));
#3621=EDGE_LOOP('',(#12796,#12797,#12798,#12799));
#3622=EDGE_LOOP('',(#12800,#12801,#12802,#12803));
#3623=EDGE_LOOP('',(#12804,#12805,#12806,#12807));
#3624=EDGE_LOOP('',(#12808,#12809,#12810,#12811));
#3625=EDGE_LOOP('',(#12812,#12813,#12814,#12815));
#3626=EDGE_LOOP('',(#12816,#12817,#12818,#12819));
#3627=EDGE_LOOP('',(#12820,#12821,#12822,#12823));
#3628=EDGE_LOOP('',(#12824,#12825,#12826,#12827));
#3629=EDGE_LOOP('',(#12828,#12829,#12830,#12831));
#3630=EDGE_LOOP('',(#12832,#12833,#12834,#12835));
#3631=EDGE_LOOP('',(#12836,#12837,#12838,#12839));
#3632=EDGE_LOOP('',(#12840,#12841,#12842,#12843));
#3633=EDGE_LOOP('',(#12844,#12845,#12846,#12847));
#3634=EDGE_LOOP('',(#12848,#12849,#12850,#12851));
#3635=EDGE_LOOP('',(#12852,#12853,#12854,#12855));
#3636=EDGE_LOOP('',(#12856,#12857,#12858,#12859,#12860,#12861,#12862,#12863,
#12864,#12865,#12866,#12867,#12868,#12869,#12870,#12871,#12872,#12873,#12874,
#12875,#12876,#12877,#12878,#12879,#12880,#12881,#12882,#12883,#12884,#12885,
#12886,#12887,#12888,#12889,#12890,#12891,#12892,#12893,#12894,#12895,#12896,
#12897,#12898,#12899,#12900,#12901,#12902,#12903,#12904,#12905,#12906,#12907,
#12908,#12909,#12910,#12911,#12912,#12913,#12914,#12915,#12916,#12917,#12918,
#12919,#12920,#12921,#12922,#12923,#12924,#12925,#12926,#12927,#12928,#12929,
#12930,#12931,#12932,#12933,#12934,#12935));
#3637=EDGE_LOOP('',(#12936));
#3638=EDGE_LOOP('',(#12937,#12938,#12939,#12940));
#4508=LINE('',#25695,#5532);
#4509=LINE('',#25697,#5533);
#4510=LINE('',#25699,#5534);
#4511=LINE('',#25700,#5535);
#4512=LINE('',#25703,#5536);
#4513=LINE('',#25705,#5537);
#4514=LINE('',#25706,#5538);
#4515=LINE('',#25709,#5539);
#4516=LINE('',#25711,#5540);
#4517=LINE('',#25712,#5541);
#4518=LINE('',#25789,#5542);
#4519=LINE('',#25935,#5543);
#4520=LINE('',#26081,#5544);
#4521=LINE('',#26227,#5545);
#4522=LINE('',#26373,#5546);
#4523=LINE('',#26519,#5547);
#4524=LINE('',#26665,#5548);
#4525=LINE('',#26811,#5549);
#4526=LINE('',#26957,#5550);
#4527=LINE('',#27103,#5551);
#4528=LINE('',#27249,#5552);
#4529=LINE('',#27395,#5553);
#4530=LINE('',#27541,#5554);
#4531=LINE('',#27687,#5555);
#4532=LINE('',#27833,#5556);
#4533=LINE('',#27979,#5557);
#4534=LINE('',#28125,#5558);
#4535=LINE('',#28271,#5559);
#4536=LINE('',#28417,#5560);
#4537=LINE('',#28563,#5561);
#4538=LINE('',#28641,#5562);
#4539=LINE('',#28785,#5563);
#4540=LINE('',#28857,#5564);
#4541=LINE('',#28860,#5565);
#4542=LINE('',#28861,#5566);
#4543=LINE('',#29073,#5567);
#4544=LINE('',#29077,#5568);
#4545=LINE('',#29289,#5569);
#4546=LINE('',#29292,#5570);
#4547=LINE('',#29293,#5571);
#4548=LINE('',#29505,#5572);
#4549=LINE('',#29509,#5573);
#4550=LINE('',#29721,#5574);
#4551=LINE('',#29724,#5575);
#4552=LINE('',#29725,#5576);
#4553=LINE('',#29937,#5577);
#4554=LINE('',#29941,#5578);
#4555=LINE('',#30153,#5579);
#4556=LINE('',#30156,#5580);
#4557=LINE('',#30157,#5581);
#4558=LINE('',#30369,#5582);
#4559=LINE('',#30373,#5583);
#4560=LINE('',#30585,#5584);
#4561=LINE('',#30588,#5585);
#4562=LINE('',#30589,#5586);
#4563=LINE('',#30801,#5587);
#4564=LINE('',#30805,#5588);
#4565=LINE('',#31017,#5589);
#4566=LINE('',#31020,#5590);
#4567=LINE('',#31021,#5591);
#4568=LINE('',#31233,#5592);
#4569=LINE('',#31237,#5593);
#4570=LINE('',#31449,#5594);
#4571=LINE('',#31452,#5595);
#4572=LINE('',#31453,#5596);
#4573=LINE('',#31665,#5597);
#4574=LINE('',#31669,#5598);
#4575=LINE('',#31881,#5599);
#4576=LINE('',#31884,#5600);
#4577=LINE('',#31885,#5601);
#4578=LINE('',#32097,#5602);
#4579=LINE('',#32101,#5603);
#4580=LINE('',#32313,#5604);
#4581=LINE('',#32316,#5605);
#4582=LINE('',#32317,#5606);
#4583=LINE('',#32529,#5607);
#4584=LINE('',#32533,#5608);
#4585=LINE('',#32745,#5609);
#4586=LINE('',#32748,#5610);
#4587=LINE('',#32749,#5611);
#4588=LINE('',#32961,#5612);
#4589=LINE('',#32965,#5613);
#4590=LINE('',#33177,#5614);
#4591=LINE('',#33180,#5615);
#4592=LINE('',#33181,#5616);
#4593=LINE('',#33393,#5617);
#4594=LINE('',#33397,#5618);
#4595=LINE('',#33609,#5619);
#4596=LINE('',#33612,#5620);
#4597=LINE('',#33613,#5621);
#4598=LINE('',#33825,#5622);
#4599=LINE('',#33829,#5623);
#4600=LINE('',#34041,#5624);
#4601=LINE('',#34044,#5625);
#4602=LINE('',#34045,#5626);
#4603=LINE('',#34257,#5627);
#4604=LINE('',#34261,#5628);
#4605=LINE('',#34473,#5629);
#4606=LINE('',#34476,#5630);
#4607=LINE('',#34477,#5631);
#4608=LINE('',#34689,#5632);
#4609=LINE('',#34693,#5633);
#4610=LINE('',#34905,#5634);
#4611=LINE('',#34908,#5635);
#4612=LINE('',#34909,#5636);
#4613=LINE('',#35121,#5637);
#4614=LINE('',#35125,#5638);
#4615=LINE('',#35337,#5639);
#4616=LINE('',#35340,#5640);
#4617=LINE('',#35341,#5641);
#4618=LINE('',#35553,#5642);
#4619=LINE('',#35557,#5643);
#4620=LINE('',#35769,#5644);
#4621=LINE('',#35772,#5645);
#4622=LINE('',#35773,#5646);
#4623=LINE('',#35985,#5647);
#4624=LINE('',#35989,#5648);
#4625=LINE('',#36201,#5649);
#4626=LINE('',#36204,#5650);
#4627=LINE('',#36205,#5651);
#4628=LINE('',#36417,#5652);
#4629=LINE('',#36421,#5653);
#4630=LINE('',#36633,#5654);
#4631=LINE('',#36636,#5655);
#4632=LINE('',#36637,#5656);
#4633=LINE('',#36849,#5657);
#4634=LINE('',#36853,#5658);
#4635=LINE('',#37065,#5659);
#4636=LINE('',#37068,#5660);
#4637=LINE('',#37069,#5661);
#4638=LINE('',#37281,#5662);
#5532=VECTOR('',#20978,1.);
#5533=VECTOR('',#20979,1.);
#5534=VECTOR('',#20980,1.);
#5535=VECTOR('',#20981,1.);
#5536=VECTOR('',#20984,1.);
#5537=VECTOR('',#20985,1.);
#5538=VECTOR('',#20986,1.);
#5539=VECTOR('',#20989,1.);
#5540=VECTOR('',#20990,1.);
#5541=VECTOR('',#20991,1.);
#5542=VECTOR('',#20996,1.);
#5543=VECTOR('',#20999,1.);
#5544=VECTOR('',#21002,1.);
#5545=VECTOR('',#21005,1.);
#5546=VECTOR('',#21008,1.);
#5547=VECTOR('',#21011,1.);
#5548=VECTOR('',#21014,1.);
#5549=VECTOR('',#21017,1.);
#5550=VECTOR('',#21020,1.);
#5551=VECTOR('',#21023,1.);
#5552=VECTOR('',#21026,1.);
#5553=VECTOR('',#21029,1.);
#5554=VECTOR('',#21032,1.);
#5555=VECTOR('',#21035,1.);
#5556=VECTOR('',#21038,1.);
#5557=VECTOR('',#21041,1.);
#5558=VECTOR('',#21044,1.);
#5559=VECTOR('',#21047,1.);
#5560=VECTOR('',#21050,1.);
#5561=VECTOR('',#21053,1.);
#5562=VECTOR('',#21064,1.4);
#5563=VECTOR('',#21069,1.);
#5564=VECTOR('',#21070,1.);
#5565=VECTOR('',#21073,1.);
#5566=VECTOR('',#21074,1.);
#5567=VECTOR('',#21075,1.);
#5568=VECTOR('',#21080,1.);
#5569=VECTOR('',#21081,1.);
#5570=VECTOR('',#21084,1.);
#5571=VECTOR('',#21085,1.);
#5572=VECTOR('',#21086,1.);
#5573=VECTOR('',#21091,1.);
#5574=VECTOR('',#21092,1.);
#5575=VECTOR('',#21095,1.);
#5576=VECTOR('',#21096,1.);
#5577=VECTOR('',#21097,1.);
#5578=VECTOR('',#21102,1.);
#5579=VECTOR('',#21103,1.);
#5580=VECTOR('',#21106,1.);
#5581=VECTOR('',#21107,1.);
#5582=VECTOR('',#21108,1.);
#5583=VECTOR('',#21113,1.);
#5584=VECTOR('',#21114,1.);
#5585=VECTOR('',#21117,1.);
#5586=VECTOR('',#21118,1.);
#5587=VECTOR('',#21119,1.);
#5588=VECTOR('',#21124,1.);
#5589=VECTOR('',#21125,1.);
#5590=VECTOR('',#21128,1.);
#5591=VECTOR('',#21129,1.);
#5592=VECTOR('',#21130,1.);
#5593=VECTOR('',#21135,1.);
#5594=VECTOR('',#21136,1.);
#5595=VECTOR('',#21139,1.);
#5596=VECTOR('',#21140,1.);
#5597=VECTOR('',#21141,1.);
#5598=VECTOR('',#21146,1.);
#5599=VECTOR('',#21147,1.);
#5600=VECTOR('',#21150,1.);
#5601=VECTOR('',#21151,1.);
#5602=VECTOR('',#21152,1.);
#5603=VECTOR('',#21157,1.);
#5604=VECTOR('',#21158,1.);
#5605=VECTOR('',#21161,1.);
#5606=VECTOR('',#21162,1.);
#5607=VECTOR('',#21163,1.);
#5608=VECTOR('',#21168,1.);
#5609=VECTOR('',#21169,1.);
#5610=VECTOR('',#21172,1.);
#5611=VECTOR('',#21173,1.);
#5612=VECTOR('',#21174,1.);
#5613=VECTOR('',#21179,1.);
#5614=VECTOR('',#21180,1.);
#5615=VECTOR('',#21183,1.);
#5616=VECTOR('',#21184,1.);
#5617=VECTOR('',#21185,1.);
#5618=VECTOR('',#21190,1.);
#5619=VECTOR('',#21191,1.);
#5620=VECTOR('',#21194,1.);
#5621=VECTOR('',#21195,1.);
#5622=VECTOR('',#21196,1.);
#5623=VECTOR('',#21201,1.);
#5624=VECTOR('',#21202,1.);
#5625=VECTOR('',#21205,1.);
#5626=VECTOR('',#21206,1.);
#5627=VECTOR('',#21207,1.);
#5628=VECTOR('',#21212,1.);
#5629=VECTOR('',#21213,1.);
#5630=VECTOR('',#21216,1.);
#5631=VECTOR('',#21217,1.);
#5632=VECTOR('',#21218,1.);
#5633=VECTOR('',#21223,1.);
#5634=VECTOR('',#21224,1.);
#5635=VECTOR('',#21227,1.);
#5636=VECTOR('',#21228,1.);
#5637=VECTOR('',#21229,1.);
#5638=VECTOR('',#21234,1.);
#5639=VECTOR('',#21235,1.);
#5640=VECTOR('',#21238,1.);
#5641=VECTOR('',#21239,1.);
#5642=VECTOR('',#21240,1.);
#5643=VECTOR('',#21245,1.);
#5644=VECTOR('',#21246,1.);
#5645=VECTOR('',#21249,1.);
#5646=VECTOR('',#21250,1.);
#5647=VECTOR('',#21251,1.);
#5648=VECTOR('',#21256,1.);
#5649=VECTOR('',#21257,1.);
#5650=VECTOR('',#21260,1.);
#5651=VECTOR('',#21261,1.);
#5652=VECTOR('',#21262,1.);
#5653=VECTOR('',#21267,1.);
#5654=VECTOR('',#21268,1.);
#5655=VECTOR('',#21271,1.);
#5656=VECTOR('',#21272,1.);
#5657=VECTOR('',#21273,1.);
#5658=VECTOR('',#21278,1.);
#5659=VECTOR('',#21279,1.);
#5660=VECTOR('',#21282,1.);
#5661=VECTOR('',#21283,1.);
#5662=VECTOR('',#21284,1.);
#6574=CIRCLE('',#17849,1.75);
#6575=CIRCLE('',#17850,1.75);
#6576=CIRCLE('',#17851,1.75);
#6577=CIRCLE('',#17852,1.75);
#6578=CIRCLE('',#17853,1.75);
#6579=CIRCLE('',#17854,1.75);
#6580=CIRCLE('',#17855,1.75);
#6581=CIRCLE('',#17856,1.75);
#6582=CIRCLE('',#17857,1.75);
#6583=CIRCLE('',#17858,1.75);
#6584=CIRCLE('',#17859,1.75);
#6585=CIRCLE('',#17860,1.75);
#6586=CIRCLE('',#17861,1.75);
#6587=CIRCLE('',#17862,1.75);
#6588=CIRCLE('',#17863,1.75);
#6589=CIRCLE('',#17864,1.75);
#6590=CIRCLE('',#17865,1.75);
#6591=CIRCLE('',#17866,1.75);
#6592=CIRCLE('',#17867,1.75);
#6593=CIRCLE('',#17868,1.75);
#6594=CIRCLE('',#17869,0.6);
#6595=CIRCLE('',#17871,0.6);
#6596=CIRCLE('',#17873,1.4);
#6597=CIRCLE('',#17874,1.4);
#6598=CIRCLE('',#17878,1.75);
#6599=CIRCLE('',#17881,1.75);
#6600=CIRCLE('',#17884,1.75);
#6601=CIRCLE('',#17887,1.75);
#6602=CIRCLE('',#17890,1.75);
#6603=CIRCLE('',#17893,1.75);
#6604=CIRCLE('',#17896,1.75);
#6605=CIRCLE('',#17899,1.75);
#6606=CIRCLE('',#17902,1.75);
#6607=CIRCLE('',#17905,1.75);
#6608=CIRCLE('',#17908,1.75);
#6609=CIRCLE('',#17911,1.75);
#6610=CIRCLE('',#17914,1.75);
#6611=CIRCLE('',#17917,1.75);
#6612=CIRCLE('',#17920,1.75);
#6613=CIRCLE('',#17923,1.75);
#6614=CIRCLE('',#17926,1.75);
#6615=CIRCLE('',#17929,1.75);
#6616=CIRCLE('',#17932,1.75);
#6617=CIRCLE('',#17935,1.75);
#7481=VERTEX_POINT('',#25693);
#7482=VERTEX_POINT('',#25694);
#7483=VERTEX_POINT('',#25696);
#7484=VERTEX_POINT('',#25698);
#7485=VERTEX_POINT('',#25702);
#7486=VERTEX_POINT('',#25704);
#7487=VERTEX_POINT('',#25708);
#7488=VERTEX_POINT('',#25710);
#7489=VERTEX_POINT('',#25714);
#7490=VERTEX_POINT('',#25715);
#7491=VERTEX_POINT('',#25717);
#7492=VERTEX_POINT('',#25788);
#7493=VERTEX_POINT('',#25790);
#7494=VERTEX_POINT('',#25861);
#7495=VERTEX_POINT('',#25863);
#7496=VERTEX_POINT('',#25934);
#7497=VERTEX_POINT('',#25936);
#7498=VERTEX_POINT('',#26007);
#7499=VERTEX_POINT('',#26009);
#7500=VERTEX_POINT('',#26080);
#7501=VERTEX_POINT('',#26082);
#7502=VERTEX_POINT('',#26153);
#7503=VERTEX_POINT('',#26155);
#7504=VERTEX_POINT('',#26226);
#7505=VERTEX_POINT('',#26228);
#7506=VERTEX_POINT('',#26299);
#7507=VERTEX_POINT('',#26301);
#7508=VERTEX_POINT('',#26372);
#7509=VERTEX_POINT('',#26374);
#7510=VERTEX_POINT('',#26445);
#7511=VERTEX_POINT('',#26447);
#7512=VERTEX_POINT('',#26518);
#7513=VERTEX_POINT('',#26520);
#7514=VERTEX_POINT('',#26591);
#7515=VERTEX_POINT('',#26593);
#7516=VERTEX_POINT('',#26664);
#7517=VERTEX_POINT('',#26666);
#7518=VERTEX_POINT('',#26737);
#7519=VERTEX_POINT('',#26739);
#7520=VERTEX_POINT('',#26810);
#7521=VERTEX_POINT('',#26812);
#7522=VERTEX_POINT('',#26883);
#7523=VERTEX_POINT('',#26885);
#7524=VERTEX_POINT('',#26956);
#7525=VERTEX_POINT('',#26958);
#7526=VERTEX_POINT('',#27029);
#7527=VERTEX_POINT('',#27031);
#7528=VERTEX_POINT('',#27102);
#7529=VERTEX_POINT('',#27104);
#7530=VERTEX_POINT('',#27175);
#7531=VERTEX_POINT('',#27177);
#7532=VERTEX_POINT('',#27248);
#7533=VERTEX_POINT('',#27250);
#7534=VERTEX_POINT('',#27321);
#7535=VERTEX_POINT('',#27323);
#7536=VERTEX_POINT('',#27394);
#7537=VERTEX_POINT('',#27396);
#7538=VERTEX_POINT('',#27467);
#7539=VERTEX_POINT('',#27469);
#7540=VERTEX_POINT('',#27540);
#7541=VERTEX_POINT('',#27542);
#7542=VERTEX_POINT('',#27613);
#7543=VERTEX_POINT('',#27615);
#7544=VERTEX_POINT('',#27686);
#7545=VERTEX_POINT('',#27688);
#7546=VERTEX_POINT('',#27759);
#7547=VERTEX_POINT('',#27761);
#7548=VERTEX_POINT('',#27832);
#7549=VERTEX_POINT('',#27834);
#7550=VERTEX_POINT('',#27905);
#7551=VERTEX_POINT('',#27907);
#7552=VERTEX_POINT('',#27978);
#7553=VERTEX_POINT('',#27980);
#7554=VERTEX_POINT('',#28051);
#7555=VERTEX_POINT('',#28053);
#7556=VERTEX_POINT('',#28124);
#7557=VERTEX_POINT('',#28126);
#7558=VERTEX_POINT('',#28197);
#7559=VERTEX_POINT('',#28199);
#7560=VERTEX_POINT('',#28270);
#7561=VERTEX_POINT('',#28272);
#7562=VERTEX_POINT('',#28343);
#7563=VERTEX_POINT('',#28345);
#7564=VERTEX_POINT('',#28416);
#7565=VERTEX_POINT('',#28418);
#7566=VERTEX_POINT('',#28489);
#7567=VERTEX_POINT('',#28491);
#7568=VERTEX_POINT('',#28562);
#7569=VERTEX_POINT('',#28638);
#7570=VERTEX_POINT('',#28640);
#7571=VERTEX_POINT('',#28784);
#7572=VERTEX_POINT('',#28786);
#7573=VERTEX_POINT('',#28859);
#7574=VERTEX_POINT('',#29002);
#7575=VERTEX_POINT('',#29075);
#7576=VERTEX_POINT('',#29218);
#7577=VERTEX_POINT('',#29291);
#7578=VERTEX_POINT('',#29434);
#7579=VERTEX_POINT('',#29507);
#7580=VERTEX_POINT('',#29650);
#7581=VERTEX_POINT('',#29723);
#7582=VERTEX_POINT('',#29866);
#7583=VERTEX_POINT('',#29939);
#7584=VERTEX_POINT('',#30082);
#7585=VERTEX_POINT('',#30155);
#7586=VERTEX_POINT('',#30298);
#7587=VERTEX_POINT('',#30371);
#7588=VERTEX_POINT('',#30514);
#7589=VERTEX_POINT('',#30587);
#7590=VERTEX_POINT('',#30730);
#7591=VERTEX_POINT('',#30803);
#7592=VERTEX_POINT('',#30946);
#7593=VERTEX_POINT('',#31019);
#7594=VERTEX_POINT('',#31162);
#7595=VERTEX_POINT('',#31235);
#7596=VERTEX_POINT('',#31378);
#7597=VERTEX_POINT('',#31451);
#7598=VERTEX_POINT('',#31594);
#7599=VERTEX_POINT('',#31667);
#7600=VERTEX_POINT('',#31810);
#7601=VERTEX_POINT('',#31883);
#7602=VERTEX_POINT('',#32026);
#7603=VERTEX_POINT('',#32099);
#7604=VERTEX_POINT('',#32242);
#7605=VERTEX_POINT('',#32315);
#7606=VERTEX_POINT('',#32458);
#7607=VERTEX_POINT('',#32531);
#7608=VERTEX_POINT('',#32674);
#7609=VERTEX_POINT('',#32747);
#7610=VERTEX_POINT('',#32890);
#7611=VERTEX_POINT('',#32963);
#7612=VERTEX_POINT('',#33106);
#7613=VERTEX_POINT('',#33179);
#7614=VERTEX_POINT('',#33322);
#7615=VERTEX_POINT('',#33395);
#7616=VERTEX_POINT('',#33538);
#7617=VERTEX_POINT('',#33611);
#7618=VERTEX_POINT('',#33754);
#7619=VERTEX_POINT('',#33827);
#7620=VERTEX_POINT('',#33970);
#7621=VERTEX_POINT('',#34043);
#7622=VERTEX_POINT('',#34186);
#7623=VERTEX_POINT('',#34259);
#7624=VERTEX_POINT('',#34402);
#7625=VERTEX_POINT('',#34475);
#7626=VERTEX_POINT('',#34618);
#7627=VERTEX_POINT('',#34691);
#7628=VERTEX_POINT('',#34834);
#7629=VERTEX_POINT('',#34907);
#7630=VERTEX_POINT('',#35050);
#7631=VERTEX_POINT('',#35123);
#7632=VERTEX_POINT('',#35266);
#7633=VERTEX_POINT('',#35339);
#7634=VERTEX_POINT('',#35482);
#7635=VERTEX_POINT('',#35555);
#7636=VERTEX_POINT('',#35698);
#7637=VERTEX_POINT('',#35771);
#7638=VERTEX_POINT('',#35914);
#7639=VERTEX_POINT('',#35987);
#7640=VERTEX_POINT('',#36130);
#7641=VERTEX_POINT('',#36203);
#7642=VERTEX_POINT('',#36346);
#7643=VERTEX_POINT('',#36419);
#7644=VERTEX_POINT('',#36562);
#7645=VERTEX_POINT('',#36635);
#7646=VERTEX_POINT('',#36778);
#7647=VERTEX_POINT('',#36851);
#7648=VERTEX_POINT('',#36994);
#7649=VERTEX_POINT('',#37067);
#7650=VERTEX_POINT('',#37210);
#9269=EDGE_CURVE('',#7481,#7482,#4508,.T.);
#9270=EDGE_CURVE('',#7483,#7481,#4509,.T.);
#9271=EDGE_CURVE('',#7484,#7483,#4510,.T.);
#9272=EDGE_CURVE('',#7482,#7484,#4511,.T.);
#9273=EDGE_CURVE('',#7485,#7481,#4512,.T.);
#9274=EDGE_CURVE('',#7485,#7486,#4513,.T.);
#9275=EDGE_CURVE('',#7483,#7486,#4514,.T.);
#9276=EDGE_CURVE('',#7487,#7485,#4515,.T.);
#9277=EDGE_CURVE('',#7488,#7487,#4516,.T.);
#9278=EDGE_CURVE('',#7486,#7488,#4517,.T.);
#9279=EDGE_CURVE('',#7489,#7490,#6574,.T.);
#9280=EDGE_CURVE('',#7490,#7491,#171,.T.);
#9281=EDGE_CURVE('',#7491,#7492,#4518,.T.);
#9282=EDGE_CURVE('',#7492,#7493,#172,.T.);
#9283=EDGE_CURVE('',#7493,#7494,#6575,.T.);
#9284=EDGE_CURVE('',#7494,#7495,#173,.T.);
#9285=EDGE_CURVE('',#7495,#7496,#4519,.T.);
#9286=EDGE_CURVE('',#7496,#7497,#174,.T.);
#9287=EDGE_CURVE('',#7497,#7498,#6576,.T.);
#9288=EDGE_CURVE('',#7498,#7499,#175,.T.);
#9289=EDGE_CURVE('',#7499,#7500,#4520,.T.);
#9290=EDGE_CURVE('',#7500,#7501,#176,.T.);
#9291=EDGE_CURVE('',#7501,#7502,#6577,.T.);
#9292=EDGE_CURVE('',#7502,#7503,#177,.T.);
#9293=EDGE_CURVE('',#7503,#7504,#4521,.T.);
#9294=EDGE_CURVE('',#7504,#7505,#178,.T.);
#9295=EDGE_CURVE('',#7505,#7506,#6578,.T.);
#9296=EDGE_CURVE('',#7506,#7507,#179,.T.);
#9297=EDGE_CURVE('',#7507,#7508,#4522,.T.);
#9298=EDGE_CURVE('',#7508,#7509,#180,.T.);
#9299=EDGE_CURVE('',#7509,#7510,#6579,.T.);
#9300=EDGE_CURVE('',#7510,#7511,#181,.T.);
#9301=EDGE_CURVE('',#7511,#7512,#4523,.T.);
#9302=EDGE_CURVE('',#7512,#7513,#182,.T.);
#9303=EDGE_CURVE('',#7513,#7514,#6580,.T.);
#9304=EDGE_CURVE('',#7514,#7515,#183,.T.);
#9305=EDGE_CURVE('',#7515,#7516,#4524,.T.);
#9306=EDGE_CURVE('',#7516,#7517,#184,.T.);
#9307=EDGE_CURVE('',#7517,#7518,#6581,.T.);
#9308=EDGE_CURVE('',#7518,#7519,#185,.T.);
#9309=EDGE_CURVE('',#7519,#7520,#4525,.T.);
#9310=EDGE_CURVE('',#7520,#7521,#186,.T.);
#9311=EDGE_CURVE('',#7521,#7522,#6582,.T.);
#9312=EDGE_CURVE('',#7522,#7523,#187,.T.);
#9313=EDGE_CURVE('',#7523,#7524,#4526,.T.);
#9314=EDGE_CURVE('',#7524,#7525,#188,.T.);
#9315=EDGE_CURVE('',#7525,#7526,#6583,.T.);
#9316=EDGE_CURVE('',#7526,#7527,#189,.T.);
#9317=EDGE_CURVE('',#7527,#7528,#4527,.T.);
#9318=EDGE_CURVE('',#7528,#7529,#190,.T.);
#9319=EDGE_CURVE('',#7529,#7530,#6584,.T.);
#9320=EDGE_CURVE('',#7530,#7531,#191,.T.);
#9321=EDGE_CURVE('',#7531,#7532,#4528,.T.);
#9322=EDGE_CURVE('',#7532,#7533,#192,.T.);
#9323=EDGE_CURVE('',#7533,#7534,#6585,.T.);
#9324=EDGE_CURVE('',#7534,#7535,#193,.T.);
#9325=EDGE_CURVE('',#7535,#7536,#4529,.T.);
#9326=EDGE_CURVE('',#7536,#7537,#194,.T.);
#9327=EDGE_CURVE('',#7537,#7538,#6586,.T.);
#9328=EDGE_CURVE('',#7538,#7539,#195,.T.);
#9329=EDGE_CURVE('',#7539,#7540,#4530,.T.);
#9330=EDGE_CURVE('',#7540,#7541,#196,.T.);
#9331=EDGE_CURVE('',#7541,#7542,#6587,.T.);
#9332=EDGE_CURVE('',#7542,#7543,#197,.T.);
#9333=EDGE_CURVE('',#7543,#7544,#4531,.T.);
#9334=EDGE_CURVE('',#7544,#7545,#198,.T.);
#9335=EDGE_CURVE('',#7545,#7546,#6588,.T.);
#9336=EDGE_CURVE('',#7546,#7547,#199,.T.);
#9337=EDGE_CURVE('',#7547,#7548,#4532,.T.);
#9338=EDGE_CURVE('',#7548,#7549,#200,.T.);
#9339=EDGE_CURVE('',#7549,#7550,#6589,.T.);
#9340=EDGE_CURVE('',#7550,#7551,#201,.T.);
#9341=EDGE_CURVE('',#7551,#7552,#4533,.T.);
#9342=EDGE_CURVE('',#7552,#7553,#202,.T.);
#9343=EDGE_CURVE('',#7553,#7554,#6590,.T.);
#9344=EDGE_CURVE('',#7554,#7555,#203,.T.);
#9345=EDGE_CURVE('',#7555,#7556,#4534,.T.);
#9346=EDGE_CURVE('',#7556,#7557,#204,.T.);
#9347=EDGE_CURVE('',#7557,#7558,#6591,.T.);
#9348=EDGE_CURVE('',#7558,#7559,#205,.T.);
#9349=EDGE_CURVE('',#7559,#7560,#4535,.T.);
#9350=EDGE_CURVE('',#7560,#7561,#206,.T.);
#9351=EDGE_CURVE('',#7561,#7562,#6592,.T.);
#9352=EDGE_CURVE('',#7562,#7563,#207,.T.);
#9353=EDGE_CURVE('',#7563,#7564,#4536,.T.);
#9354=EDGE_CURVE('',#7564,#7565,#208,.T.);
#9355=EDGE_CURVE('',#7565,#7566,#6593,.T.);
#9356=EDGE_CURVE('',#7566,#7567,#209,.T.);
#9357=EDGE_CURVE('',#7567,#7568,#4537,.T.);
#9358=EDGE_CURVE('',#7568,#7489,#210,.T.);
#9359=EDGE_CURVE('',#7488,#7484,#6594,.T.);
#9360=EDGE_CURVE('',#7482,#7487,#6595,.T.);
#9361=EDGE_CURVE('',#7569,#7569,#6596,.T.);
#9362=EDGE_CURVE('',#7569,#7570,#4538,.T.);
#9363=EDGE_CURVE('',#7570,#7570,#6597,.T.);
#9364=EDGE_CURVE('',#7571,#7566,#4539,.T.);
#9365=EDGE_CURVE('',#7572,#7571,#211,.T.);
#9366=EDGE_CURVE('',#7567,#7572,#4540,.T.);
#9367=EDGE_CURVE('',#7573,#7572,#4541,.T.);
#9368=EDGE_CURVE('',#7568,#7573,#4542,.T.);
#9369=EDGE_CURVE('',#7574,#7573,#212,.T.);
#9370=EDGE_CURVE('',#7489,#7574,#4543,.T.);
#9371=EDGE_CURVE('',#7575,#7574,#6598,.T.);
#9372=EDGE_CURVE('',#7575,#7490,#4544,.T.);
#9373=EDGE_CURVE('',#7576,#7575,#213,.T.);
#9374=EDGE_CURVE('',#7491,#7576,#4545,.T.);
#9375=EDGE_CURVE('',#7577,#7576,#4546,.T.);
#9376=EDGE_CURVE('',#7492,#7577,#4547,.T.);
#9377=EDGE_CURVE('',#7578,#7577,#214,.T.);
#9378=EDGE_CURVE('',#7493,#7578,#4548,.T.);
#9379=EDGE_CURVE('',#7579,#7578,#6599,.T.);
#9380=EDGE_CURVE('',#7579,#7494,#4549,.T.);
#9381=EDGE_CURVE('',#7580,#7579,#215,.T.);
#9382=EDGE_CURVE('',#7495,#7580,#4550,.T.);
#9383=EDGE_CURVE('',#7581,#7580,#4551,.T.);
#9384=EDGE_CURVE('',#7496,#7581,#4552,.T.);
#9385=EDGE_CURVE('',#7582,#7581,#216,.T.);
#9386=EDGE_CURVE('',#7497,#7582,#4553,.T.);
#9387=EDGE_CURVE('',#7583,#7582,#6600,.T.);
#9388=EDGE_CURVE('',#7583,#7498,#4554,.T.);
#9389=EDGE_CURVE('',#7584,#7583,#217,.T.);
#9390=EDGE_CURVE('',#7499,#7584,#4555,.T.);
#9391=EDGE_CURVE('',#7585,#7584,#4556,.T.);
#9392=EDGE_CURVE('',#7500,#7585,#4557,.T.);
#9393=EDGE_CURVE('',#7586,#7585,#218,.T.);
#9394=EDGE_CURVE('',#7501,#7586,#4558,.T.);
#9395=EDGE_CURVE('',#7587,#7586,#6601,.T.);
#9396=EDGE_CURVE('',#7587,#7502,#4559,.T.);
#9397=EDGE_CURVE('',#7588,#7587,#219,.T.);
#9398=EDGE_CURVE('',#7503,#7588,#4560,.T.);
#9399=EDGE_CURVE('',#7589,#7588,#4561,.T.);
#9400=EDGE_CURVE('',#7504,#7589,#4562,.T.);
#9401=EDGE_CURVE('',#7590,#7589,#220,.T.);
#9402=EDGE_CURVE('',#7505,#7590,#4563,.T.);
#9403=EDGE_CURVE('',#7591,#7590,#6602,.T.);
#9404=EDGE_CURVE('',#7591,#7506,#4564,.T.);
#9405=EDGE_CURVE('',#7592,#7591,#221,.T.);
#9406=EDGE_CURVE('',#7507,#7592,#4565,.T.);
#9407=EDGE_CURVE('',#7593,#7592,#4566,.T.);
#9408=EDGE_CURVE('',#7508,#7593,#4567,.T.);
#9409=EDGE_CURVE('',#7594,#7593,#222,.T.);
#9410=EDGE_CURVE('',#7509,#7594,#4568,.T.);
#9411=EDGE_CURVE('',#7595,#7594,#6603,.T.);
#9412=EDGE_CURVE('',#7595,#7510,#4569,.T.);
#9413=EDGE_CURVE('',#7596,#7595,#223,.T.);
#9414=EDGE_CURVE('',#7511,#7596,#4570,.T.);
#9415=EDGE_CURVE('',#7597,#7596,#4571,.T.);
#9416=EDGE_CURVE('',#7512,#7597,#4572,.T.);
#9417=EDGE_CURVE('',#7598,#7597,#224,.T.);
#9418=EDGE_CURVE('',#7513,#7598,#4573,.T.);
#9419=EDGE_CURVE('',#7599,#7598,#6604,.T.);
#9420=EDGE_CURVE('',#7599,#7514,#4574,.T.);
#9421=EDGE_CURVE('',#7600,#7599,#225,.T.);
#9422=EDGE_CURVE('',#7515,#7600,#4575,.T.);
#9423=EDGE_CURVE('',#7601,#7600,#4576,.T.);
#9424=EDGE_CURVE('',#7516,#7601,#4577,.T.);
#9425=EDGE_CURVE('',#7602,#7601,#226,.T.);
#9426=EDGE_CURVE('',#7517,#7602,#4578,.T.);
#9427=EDGE_CURVE('',#7603,#7602,#6605,.T.);
#9428=EDGE_CURVE('',#7603,#7518,#4579,.T.);
#9429=EDGE_CURVE('',#7604,#7603,#227,.T.);
#9430=EDGE_CURVE('',#7519,#7604,#4580,.T.);
#9431=EDGE_CURVE('',#7605,#7604,#4581,.T.);
#9432=EDGE_CURVE('',#7520,#7605,#4582,.T.);
#9433=EDGE_CURVE('',#7606,#7605,#228,.T.);
#9434=EDGE_CURVE('',#7521,#7606,#4583,.T.);
#9435=EDGE_CURVE('',#7607,#7606,#6606,.T.);
#9436=EDGE_CURVE('',#7607,#7522,#4584,.T.);
#9437=EDGE_CURVE('',#7608,#7607,#229,.T.);
#9438=EDGE_CURVE('',#7523,#7608,#4585,.T.);
#9439=EDGE_CURVE('',#7609,#7608,#4586,.T.);
#9440=EDGE_CURVE('',#7524,#7609,#4587,.T.);
#9441=EDGE_CURVE('',#7610,#7609,#230,.T.);
#9442=EDGE_CURVE('',#7525,#7610,#4588,.T.);
#9443=EDGE_CURVE('',#7611,#7610,#6607,.T.);
#9444=EDGE_CURVE('',#7611,#7526,#4589,.T.);
#9445=EDGE_CURVE('',#7612,#7611,#231,.T.);
#9446=EDGE_CURVE('',#7527,#7612,#4590,.T.);
#9447=EDGE_CURVE('',#7613,#7612,#4591,.T.);
#9448=EDGE_CURVE('',#7528,#7613,#4592,.T.);
#9449=EDGE_CURVE('',#7614,#7613,#232,.T.);
#9450=EDGE_CURVE('',#7529,#7614,#4593,.T.);
#9451=EDGE_CURVE('',#7615,#7614,#6608,.T.);
#9452=EDGE_CURVE('',#7615,#7530,#4594,.T.);
#9453=EDGE_CURVE('',#7616,#7615,#233,.T.);
#9454=EDGE_CURVE('',#7531,#7616,#4595,.T.);
#9455=EDGE_CURVE('',#7617,#7616,#4596,.T.);
#9456=EDGE_CURVE('',#7532,#7617,#4597,.T.);
#9457=EDGE_CURVE('',#7618,#7617,#234,.T.);
#9458=EDGE_CURVE('',#7533,#7618,#4598,.T.);
#9459=EDGE_CURVE('',#7619,#7618,#6609,.T.);
#9460=EDGE_CURVE('',#7619,#7534,#4599,.T.);
#9461=EDGE_CURVE('',#7620,#7619,#235,.T.);
#9462=EDGE_CURVE('',#7535,#7620,#4600,.T.);
#9463=EDGE_CURVE('',#7621,#7620,#4601,.T.);
#9464=EDGE_CURVE('',#7536,#7621,#4602,.T.);
#9465=EDGE_CURVE('',#7622,#7621,#236,.T.);
#9466=EDGE_CURVE('',#7537,#7622,#4603,.T.);
#9467=EDGE_CURVE('',#7623,#7622,#6610,.T.);
#9468=EDGE_CURVE('',#7623,#7538,#4604,.T.);
#9469=EDGE_CURVE('',#7624,#7623,#237,.T.);
#9470=EDGE_CURVE('',#7539,#7624,#4605,.T.);
#9471=EDGE_CURVE('',#7625,#7624,#4606,.T.);
#9472=EDGE_CURVE('',#7540,#7625,#4607,.T.);
#9473=EDGE_CURVE('',#7626,#7625,#238,.T.);
#9474=EDGE_CURVE('',#7541,#7626,#4608,.T.);
#9475=EDGE_CURVE('',#7627,#7626,#6611,.T.);
#9476=EDGE_CURVE('',#7627,#7542,#4609,.T.);
#9477=EDGE_CURVE('',#7628,#7627,#239,.T.);
#9478=EDGE_CURVE('',#7543,#7628,#4610,.T.);
#9479=EDGE_CURVE('',#7629,#7628,#4611,.T.);
#9480=EDGE_CURVE('',#7544,#7629,#4612,.T.);
#9481=EDGE_CURVE('',#7630,#7629,#240,.T.);
#9482=EDGE_CURVE('',#7545,#7630,#4613,.T.);
#9483=EDGE_CURVE('',#7631,#7630,#6612,.T.);
#9484=EDGE_CURVE('',#7631,#7546,#4614,.T.);
#9485=EDGE_CURVE('',#7632,#7631,#241,.T.);
#9486=EDGE_CURVE('',#7547,#7632,#4615,.T.);
#9487=EDGE_CURVE('',#7633,#7632,#4616,.T.);
#9488=EDGE_CURVE('',#7548,#7633,#4617,.T.);
#9489=EDGE_CURVE('',#7634,#7633,#242,.T.);
#9490=EDGE_CURVE('',#7549,#7634,#4618,.T.);
#9491=EDGE_CURVE('',#7635,#7634,#6613,.T.);
#9492=EDGE_CURVE('',#7635,#7550,#4619,.T.);
#9493=EDGE_CURVE('',#7636,#7635,#243,.T.);
#9494=EDGE_CURVE('',#7551,#7636,#4620,.T.);
#9495=EDGE_CURVE('',#7637,#7636,#4621,.T.);
#9496=EDGE_CURVE('',#7552,#7637,#4622,.T.);
#9497=EDGE_CURVE('',#7638,#7637,#244,.T.);
#9498=EDGE_CURVE('',#7553,#7638,#4623,.T.);
#9499=EDGE_CURVE('',#7639,#7638,#6614,.T.);
#9500=EDGE_CURVE('',#7639,#7554,#4624,.T.);
#9501=EDGE_CURVE('',#7640,#7639,#245,.T.);
#9502=EDGE_CURVE('',#7555,#7640,#4625,.T.);
#9503=EDGE_CURVE('',#7641,#7640,#4626,.T.);
#9504=EDGE_CURVE('',#7556,#7641,#4627,.T.);
#9505=EDGE_CURVE('',#7642,#7641,#246,.T.);
#9506=EDGE_CURVE('',#7557,#7642,#4628,.T.);
#9507=EDGE_CURVE('',#7643,#7642,#6615,.T.);
#9508=EDGE_CURVE('',#7643,#7558,#4629,.T.);
#9509=EDGE_CURVE('',#7644,#7643,#247,.T.);
#9510=EDGE_CURVE('',#7559,#7644,#4630,.T.);
#9511=EDGE_CURVE('',#7645,#7644,#4631,.T.);
#9512=EDGE_CURVE('',#7560,#7645,#4632,.T.);
#9513=EDGE_CURVE('',#7646,#7645,#248,.T.);
#9514=EDGE_CURVE('',#7561,#7646,#4633,.T.);
#9515=EDGE_CURVE('',#7647,#7646,#6616,.T.);
#9516=EDGE_CURVE('',#7647,#7562,#4634,.T.);
#9517=EDGE_CURVE('',#7648,#7647,#249,.T.);
#9518=EDGE_CURVE('',#7563,#7648,#4635,.T.);
#9519=EDGE_CURVE('',#7649,#7648,#4636,.T.);
#9520=EDGE_CURVE('',#7564,#7649,#4637,.T.);
#9521=EDGE_CURVE('',#7650,#7649,#250,.T.);
#9522=EDGE_CURVE('',#7565,#7650,#4638,.T.);
#9523=EDGE_CURVE('',#7571,#7650,#6617,.T.);
#12431=ORIENTED_EDGE('',*,*,#9269,.F.);
#12432=ORIENTED_EDGE('',*,*,#9270,.F.);
#12433=ORIENTED_EDGE('',*,*,#9271,.F.);
#12434=ORIENTED_EDGE('',*,*,#9272,.F.);
#12435=ORIENTED_EDGE('',*,*,#9273,.F.);
#12436=ORIENTED_EDGE('',*,*,#9274,.T.);
#12437=ORIENTED_EDGE('',*,*,#9275,.F.);
#12438=ORIENTED_EDGE('',*,*,#9270,.T.);
#12439=ORIENTED_EDGE('',*,*,#9276,.F.);
#12440=ORIENTED_EDGE('',*,*,#9277,.F.);
#12441=ORIENTED_EDGE('',*,*,#9278,.F.);
#12442=ORIENTED_EDGE('',*,*,#9274,.F.);
#12443=ORIENTED_EDGE('',*,*,#9279,.T.);
#12444=ORIENTED_EDGE('',*,*,#9280,.T.);
#12445=ORIENTED_EDGE('',*,*,#9281,.T.);
#12446=ORIENTED_EDGE('',*,*,#9282,.T.);
#12447=ORIENTED_EDGE('',*,*,#9283,.T.);
#12448=ORIENTED_EDGE('',*,*,#9284,.T.);
#12449=ORIENTED_EDGE('',*,*,#9285,.T.);
#12450=ORIENTED_EDGE('',*,*,#9286,.T.);
#12451=ORIENTED_EDGE('',*,*,#9287,.T.);
#12452=ORIENTED_EDGE('',*,*,#9288,.T.);
#12453=ORIENTED_EDGE('',*,*,#9289,.T.);
#12454=ORIENTED_EDGE('',*,*,#9290,.T.);
#12455=ORIENTED_EDGE('',*,*,#9291,.T.);
#12456=ORIENTED_EDGE('',*,*,#9292,.T.);
#12457=ORIENTED_EDGE('',*,*,#9293,.T.);
#12458=ORIENTED_EDGE('',*,*,#9294,.T.);
#12459=ORIENTED_EDGE('',*,*,#9295,.T.);
#12460=ORIENTED_EDGE('',*,*,#9296,.T.);
#12461=ORIENTED_EDGE('',*,*,#9297,.T.);
#12462=ORIENTED_EDGE('',*,*,#9298,.T.);
#12463=ORIENTED_EDGE('',*,*,#9299,.T.);
#12464=ORIENTED_EDGE('',*,*,#9300,.T.);
#12465=ORIENTED_EDGE('',*,*,#9301,.T.);
#12466=ORIENTED_EDGE('',*,*,#9302,.T.);
#12467=ORIENTED_EDGE('',*,*,#9303,.T.);
#12468=ORIENTED_EDGE('',*,*,#9304,.T.);
#12469=ORIENTED_EDGE('',*,*,#9305,.T.);
#12470=ORIENTED_EDGE('',*,*,#9306,.T.);
#12471=ORIENTED_EDGE('',*,*,#9307,.T.);
#12472=ORIENTED_EDGE('',*,*,#9308,.T.);
#12473=ORIENTED_EDGE('',*,*,#9309,.T.);
#12474=ORIENTED_EDGE('',*,*,#9310,.T.);
#12475=ORIENTED_EDGE('',*,*,#9311,.T.);
#12476=ORIENTED_EDGE('',*,*,#9312,.T.);
#12477=ORIENTED_EDGE('',*,*,#9313,.T.);
#12478=ORIENTED_EDGE('',*,*,#9314,.T.);
#12479=ORIENTED_EDGE('',*,*,#9315,.T.);
#12480=ORIENTED_EDGE('',*,*,#9316,.T.);
#12481=ORIENTED_EDGE('',*,*,#9317,.T.);
#12482=ORIENTED_EDGE('',*,*,#9318,.T.);
#12483=ORIENTED_EDGE('',*,*,#9319,.T.);
#12484=ORIENTED_EDGE('',*,*,#9320,.T.);
#12485=ORIENTED_EDGE('',*,*,#9321,.T.);
#12486=ORIENTED_EDGE('',*,*,#9322,.T.);
#12487=ORIENTED_EDGE('',*,*,#9323,.T.);
#12488=ORIENTED_EDGE('',*,*,#9324,.T.);
#12489=ORIENTED_EDGE('',*,*,#9325,.T.);
#12490=ORIENTED_EDGE('',*,*,#9326,.T.);
#12491=ORIENTED_EDGE('',*,*,#9327,.T.);
#12492=ORIENTED_EDGE('',*,*,#9328,.T.);
#12493=ORIENTED_EDGE('',*,*,#9329,.T.);
#12494=ORIENTED_EDGE('',*,*,#9330,.T.);
#12495=ORIENTED_EDGE('',*,*,#9331,.T.);
#12496=ORIENTED_EDGE('',*,*,#9332,.T.);
#12497=ORIENTED_EDGE('',*,*,#9333,.T.);
#12498=ORIENTED_EDGE('',*,*,#9334,.T.);
#12499=ORIENTED_EDGE('',*,*,#9335,.T.);
#12500=ORIENTED_EDGE('',*,*,#9336,.T.);
#12501=ORIENTED_EDGE('',*,*,#9337,.T.);
#12502=ORIENTED_EDGE('',*,*,#9338,.T.);
#12503=ORIENTED_EDGE('',*,*,#9339,.T.);
#12504=ORIENTED_EDGE('',*,*,#9340,.T.);
#12505=ORIENTED_EDGE('',*,*,#9341,.T.);
#12506=ORIENTED_EDGE('',*,*,#9342,.T.);
#12507=ORIENTED_EDGE('',*,*,#9343,.T.);
#12508=ORIENTED_EDGE('',*,*,#9344,.T.);
#12509=ORIENTED_EDGE('',*,*,#9345,.T.);
#12510=ORIENTED_EDGE('',*,*,#9346,.T.);
#12511=ORIENTED_EDGE('',*,*,#9347,.T.);
#12512=ORIENTED_EDGE('',*,*,#9348,.T.);
#12513=ORIENTED_EDGE('',*,*,#9349,.T.);
#12514=ORIENTED_EDGE('',*,*,#9350,.T.);
#12515=ORIENTED_EDGE('',*,*,#9351,.T.);
#12516=ORIENTED_EDGE('',*,*,#9352,.T.);
#12517=ORIENTED_EDGE('',*,*,#9353,.T.);
#12518=ORIENTED_EDGE('',*,*,#9354,.T.);
#12519=ORIENTED_EDGE('',*,*,#9355,.T.);
#12520=ORIENTED_EDGE('',*,*,#9356,.T.);
#12521=ORIENTED_EDGE('',*,*,#9357,.T.);
#12522=ORIENTED_EDGE('',*,*,#9358,.T.);
#12523=ORIENTED_EDGE('',*,*,#9271,.T.);
#12524=ORIENTED_EDGE('',*,*,#9275,.T.);
#12525=ORIENTED_EDGE('',*,*,#9278,.T.);
#12526=ORIENTED_EDGE('',*,*,#9359,.T.);
#12527=ORIENTED_EDGE('',*,*,#9272,.T.);
#12528=ORIENTED_EDGE('',*,*,#9359,.F.);
#12529=ORIENTED_EDGE('',*,*,#9277,.T.);
#12530=ORIENTED_EDGE('',*,*,#9360,.F.);
#12531=ORIENTED_EDGE('',*,*,#9361,.F.);
#12532=ORIENTED_EDGE('',*,*,#9362,.T.);
#12533=ORIENTED_EDGE('',*,*,#9363,.F.);
#12534=ORIENTED_EDGE('',*,*,#9362,.F.);
#12535=ORIENTED_EDGE('',*,*,#9361,.T.);
#12536=ORIENTED_EDGE('',*,*,#9269,.T.);
#12537=ORIENTED_EDGE('',*,*,#9360,.T.);
#12538=ORIENTED_EDGE('',*,*,#9276,.T.);
#12539=ORIENTED_EDGE('',*,*,#9273,.T.);
#12540=ORIENTED_EDGE('',*,*,#9364,.F.);
#12541=ORIENTED_EDGE('',*,*,#9365,.F.);
#12542=ORIENTED_EDGE('',*,*,#9366,.F.);
#12543=ORIENTED_EDGE('',*,*,#9356,.F.);
#12544=ORIENTED_EDGE('',*,*,#9366,.T.);
#12545=ORIENTED_EDGE('',*,*,#9367,.F.);
#12546=ORIENTED_EDGE('',*,*,#9368,.F.);
#12547=ORIENTED_EDGE('',*,*,#9357,.F.);
#12548=ORIENTED_EDGE('',*,*,#9368,.T.);
#12549=ORIENTED_EDGE('',*,*,#9369,.F.);
#12550=ORIENTED_EDGE('',*,*,#9370,.F.);
#12551=ORIENTED_EDGE('',*,*,#9358,.F.);
#12552=ORIENTED_EDGE('',*,*,#9370,.T.);
#12553=ORIENTED_EDGE('',*,*,#9371,.F.);
#12554=ORIENTED_EDGE('',*,*,#9372,.T.);
#12555=ORIENTED_EDGE('',*,*,#9279,.F.);
#12556=ORIENTED_EDGE('',*,*,#9372,.F.);
#12557=ORIENTED_EDGE('',*,*,#9373,.F.);
#12558=ORIENTED_EDGE('',*,*,#9374,.F.);
#12559=ORIENTED_EDGE('',*,*,#9280,.F.);
#12560=ORIENTED_EDGE('',*,*,#9374,.T.);
#12561=ORIENTED_EDGE('',*,*,#9375,.F.);
#12562=ORIENTED_EDGE('',*,*,#9376,.F.);
#12563=ORIENTED_EDGE('',*,*,#9281,.F.);
#12564=ORIENTED_EDGE('',*,*,#9376,.T.);
#12565=ORIENTED_EDGE('',*,*,#9377,.F.);
#12566=ORIENTED_EDGE('',*,*,#9378,.F.);
#12567=ORIENTED_EDGE('',*,*,#9282,.F.);
#12568=ORIENTED_EDGE('',*,*,#9378,.T.);
#12569=ORIENTED_EDGE('',*,*,#9379,.F.);
#12570=ORIENTED_EDGE('',*,*,#9380,.T.);
#12571=ORIENTED_EDGE('',*,*,#9283,.F.);
#12572=ORIENTED_EDGE('',*,*,#9380,.F.);
#12573=ORIENTED_EDGE('',*,*,#9381,.F.);
#12574=ORIENTED_EDGE('',*,*,#9382,.F.);
#12575=ORIENTED_EDGE('',*,*,#9284,.F.);
#12576=ORIENTED_EDGE('',*,*,#9382,.T.);
#12577=ORIENTED_EDGE('',*,*,#9383,.F.);
#12578=ORIENTED_EDGE('',*,*,#9384,.F.);
#12579=ORIENTED_EDGE('',*,*,#9285,.F.);
#12580=ORIENTED_EDGE('',*,*,#9384,.T.);
#12581=ORIENTED_EDGE('',*,*,#9385,.F.);
#12582=ORIENTED_EDGE('',*,*,#9386,.F.);
#12583=ORIENTED_EDGE('',*,*,#9286,.F.);
#12584=ORIENTED_EDGE('',*,*,#9386,.T.);
#12585=ORIENTED_EDGE('',*,*,#9387,.F.);
#12586=ORIENTED_EDGE('',*,*,#9388,.T.);
#12587=ORIENTED_EDGE('',*,*,#9287,.F.);
#12588=ORIENTED_EDGE('',*,*,#9388,.F.);
#12589=ORIENTED_EDGE('',*,*,#9389,.F.);
#12590=ORIENTED_EDGE('',*,*,#9390,.F.);
#12591=ORIENTED_EDGE('',*,*,#9288,.F.);
#12592=ORIENTED_EDGE('',*,*,#9390,.T.);
#12593=ORIENTED_EDGE('',*,*,#9391,.F.);
#12594=ORIENTED_EDGE('',*,*,#9392,.F.);
#12595=ORIENTED_EDGE('',*,*,#9289,.F.);
#12596=ORIENTED_EDGE('',*,*,#9392,.T.);
#12597=ORIENTED_EDGE('',*,*,#9393,.F.);
#12598=ORIENTED_EDGE('',*,*,#9394,.F.);
#12599=ORIENTED_EDGE('',*,*,#9290,.F.);
#12600=ORIENTED_EDGE('',*,*,#9394,.T.);
#12601=ORIENTED_EDGE('',*,*,#9395,.F.);
#12602=ORIENTED_EDGE('',*,*,#9396,.T.);
#12603=ORIENTED_EDGE('',*,*,#9291,.F.);
#12604=ORIENTED_EDGE('',*,*,#9396,.F.);
#12605=ORIENTED_EDGE('',*,*,#9397,.F.);
#12606=ORIENTED_EDGE('',*,*,#9398,.F.);
#12607=ORIENTED_EDGE('',*,*,#9292,.F.);
#12608=ORIENTED_EDGE('',*,*,#9398,.T.);
#12609=ORIENTED_EDGE('',*,*,#9399,.F.);
#12610=ORIENTED_EDGE('',*,*,#9400,.F.);
#12611=ORIENTED_EDGE('',*,*,#9293,.F.);
#12612=ORIENTED_EDGE('',*,*,#9400,.T.);
#12613=ORIENTED_EDGE('',*,*,#9401,.F.);
#12614=ORIENTED_EDGE('',*,*,#9402,.F.);
#12615=ORIENTED_EDGE('',*,*,#9294,.F.);
#12616=ORIENTED_EDGE('',*,*,#9402,.T.);
#12617=ORIENTED_EDGE('',*,*,#9403,.F.);
#12618=ORIENTED_EDGE('',*,*,#9404,.T.);
#12619=ORIENTED_EDGE('',*,*,#9295,.F.);
#12620=ORIENTED_EDGE('',*,*,#9404,.F.);
#12621=ORIENTED_EDGE('',*,*,#9405,.F.);
#12622=ORIENTED_EDGE('',*,*,#9406,.F.);
#12623=ORIENTED_EDGE('',*,*,#9296,.F.);
#12624=ORIENTED_EDGE('',*,*,#9406,.T.);
#12625=ORIENTED_EDGE('',*,*,#9407,.F.);
#12626=ORIENTED_EDGE('',*,*,#9408,.F.);
#12627=ORIENTED_EDGE('',*,*,#9297,.F.);
#12628=ORIENTED_EDGE('',*,*,#9408,.T.);
#12629=ORIENTED_EDGE('',*,*,#9409,.F.);
#12630=ORIENTED_EDGE('',*,*,#9410,.F.);
#12631=ORIENTED_EDGE('',*,*,#9298,.F.);
#12632=ORIENTED_EDGE('',*,*,#9410,.T.);
#12633=ORIENTED_EDGE('',*,*,#9411,.F.);
#12634=ORIENTED_EDGE('',*,*,#9412,.T.);
#12635=ORIENTED_EDGE('',*,*,#9299,.F.);
#12636=ORIENTED_EDGE('',*,*,#9412,.F.);
#12637=ORIENTED_EDGE('',*,*,#9413,.F.);
#12638=ORIENTED_EDGE('',*,*,#9414,.F.);
#12639=ORIENTED_EDGE('',*,*,#9300,.F.);
#12640=ORIENTED_EDGE('',*,*,#9414,.T.);
#12641=ORIENTED_EDGE('',*,*,#9415,.F.);
#12642=ORIENTED_EDGE('',*,*,#9416,.F.);
#12643=ORIENTED_EDGE('',*,*,#9301,.F.);
#12644=ORIENTED_EDGE('',*,*,#9416,.T.);
#12645=ORIENTED_EDGE('',*,*,#9417,.F.);
#12646=ORIENTED_EDGE('',*,*,#9418,.F.);
#12647=ORIENTED_EDGE('',*,*,#9302,.F.);
#12648=ORIENTED_EDGE('',*,*,#9418,.T.);
#12649=ORIENTED_EDGE('',*,*,#9419,.F.);
#12650=ORIENTED_EDGE('',*,*,#9420,.T.);
#12651=ORIENTED_EDGE('',*,*,#9303,.F.);
#12652=ORIENTED_EDGE('',*,*,#9420,.F.);
#12653=ORIENTED_EDGE('',*,*,#9421,.F.);
#12654=ORIENTED_EDGE('',*,*,#9422,.F.);
#12655=ORIENTED_EDGE('',*,*,#9304,.F.);
#12656=ORIENTED_EDGE('',*,*,#9422,.T.);
#12657=ORIENTED_EDGE('',*,*,#9423,.F.);
#12658=ORIENTED_EDGE('',*,*,#9424,.F.);
#12659=ORIENTED_EDGE('',*,*,#9305,.F.);
#12660=ORIENTED_EDGE('',*,*,#9424,.T.);
#12661=ORIENTED_EDGE('',*,*,#9425,.F.);
#12662=ORIENTED_EDGE('',*,*,#9426,.F.);
#12663=ORIENTED_EDGE('',*,*,#9306,.F.);
#12664=ORIENTED_EDGE('',*,*,#9426,.T.);
#12665=ORIENTED_EDGE('',*,*,#9427,.F.);
#12666=ORIENTED_EDGE('',*,*,#9428,.T.);
#12667=ORIENTED_EDGE('',*,*,#9307,.F.);
#12668=ORIENTED_EDGE('',*,*,#9428,.F.);
#12669=ORIENTED_EDGE('',*,*,#9429,.F.);
#12670=ORIENTED_EDGE('',*,*,#9430,.F.);
#12671=ORIENTED_EDGE('',*,*,#9308,.F.);
#12672=ORIENTED_EDGE('',*,*,#9430,.T.);
#12673=ORIENTED_EDGE('',*,*,#9431,.F.);
#12674=ORIENTED_EDGE('',*,*,#9432,.F.);
#12675=ORIENTED_EDGE('',*,*,#9309,.F.);
#12676=ORIENTED_EDGE('',*,*,#9432,.T.);
#12677=ORIENTED_EDGE('',*,*,#9433,.F.);
#12678=ORIENTED_EDGE('',*,*,#9434,.F.);
#12679=ORIENTED_EDGE('',*,*,#9310,.F.);
#12680=ORIENTED_EDGE('',*,*,#9434,.T.);
#12681=ORIENTED_EDGE('',*,*,#9435,.F.);
#12682=ORIENTED_EDGE('',*,*,#9436,.T.);
#12683=ORIENTED_EDGE('',*,*,#9311,.F.);
#12684=ORIENTED_EDGE('',*,*,#9436,.F.);
#12685=ORIENTED_EDGE('',*,*,#9437,.F.);
#12686=ORIENTED_EDGE('',*,*,#9438,.F.);
#12687=ORIENTED_EDGE('',*,*,#9312,.F.);
#12688=ORIENTED_EDGE('',*,*,#9438,.T.);
#12689=ORIENTED_EDGE('',*,*,#9439,.F.);
#12690=ORIENTED_EDGE('',*,*,#9440,.F.);
#12691=ORIENTED_EDGE('',*,*,#9313,.F.);
#12692=ORIENTED_EDGE('',*,*,#9440,.T.);
#12693=ORIENTED_EDGE('',*,*,#9441,.F.);
#12694=ORIENTED_EDGE('',*,*,#9442,.F.);
#12695=ORIENTED_EDGE('',*,*,#9314,.F.);
#12696=ORIENTED_EDGE('',*,*,#9442,.T.);
#12697=ORIENTED_EDGE('',*,*,#9443,.F.);
#12698=ORIENTED_EDGE('',*,*,#9444,.T.);
#12699=ORIENTED_EDGE('',*,*,#9315,.F.);
#12700=ORIENTED_EDGE('',*,*,#9444,.F.);
#12701=ORIENTED_EDGE('',*,*,#9445,.F.);
#12702=ORIENTED_EDGE('',*,*,#9446,.F.);
#12703=ORIENTED_EDGE('',*,*,#9316,.F.);
#12704=ORIENTED_EDGE('',*,*,#9446,.T.);
#12705=ORIENTED_EDGE('',*,*,#9447,.F.);
#12706=ORIENTED_EDGE('',*,*,#9448,.F.);
#12707=ORIENTED_EDGE('',*,*,#9317,.F.);
#12708=ORIENTED_EDGE('',*,*,#9448,.T.);
#12709=ORIENTED_EDGE('',*,*,#9449,.F.);
#12710=ORIENTED_EDGE('',*,*,#9450,.F.);
#12711=ORIENTED_EDGE('',*,*,#9318,.F.);
#12712=ORIENTED_EDGE('',*,*,#9450,.T.);
#12713=ORIENTED_EDGE('',*,*,#9451,.F.);
#12714=ORIENTED_EDGE('',*,*,#9452,.T.);
#12715=ORIENTED_EDGE('',*,*,#9319,.F.);
#12716=ORIENTED_EDGE('',*,*,#9452,.F.);
#12717=ORIENTED_EDGE('',*,*,#9453,.F.);
#12718=ORIENTED_EDGE('',*,*,#9454,.F.);
#12719=ORIENTED_EDGE('',*,*,#9320,.F.);
#12720=ORIENTED_EDGE('',*,*,#9454,.T.);
#12721=ORIENTED_EDGE('',*,*,#9455,.F.);
#12722=ORIENTED_EDGE('',*,*,#9456,.F.);
#12723=ORIENTED_EDGE('',*,*,#9321,.F.);
#12724=ORIENTED_EDGE('',*,*,#9456,.T.);
#12725=ORIENTED_EDGE('',*,*,#9457,.F.);
#12726=ORIENTED_EDGE('',*,*,#9458,.F.);
#12727=ORIENTED_EDGE('',*,*,#9322,.F.);
#12728=ORIENTED_EDGE('',*,*,#9458,.T.);
#12729=ORIENTED_EDGE('',*,*,#9459,.F.);
#12730=ORIENTED_EDGE('',*,*,#9460,.T.);
#12731=ORIENTED_EDGE('',*,*,#9323,.F.);
#12732=ORIENTED_EDGE('',*,*,#9460,.F.);
#12733=ORIENTED_EDGE('',*,*,#9461,.F.);
#12734=ORIENTED_EDGE('',*,*,#9462,.F.);
#12735=ORIENTED_EDGE('',*,*,#9324,.F.);
#12736=ORIENTED_EDGE('',*,*,#9462,.T.);
#12737=ORIENTED_EDGE('',*,*,#9463,.F.);
#12738=ORIENTED_EDGE('',*,*,#9464,.F.);
#12739=ORIENTED_EDGE('',*,*,#9325,.F.);
#12740=ORIENTED_EDGE('',*,*,#9464,.T.);
#12741=ORIENTED_EDGE('',*,*,#9465,.F.);
#12742=ORIENTED_EDGE('',*,*,#9466,.F.);
#12743=ORIENTED_EDGE('',*,*,#9326,.F.);
#12744=ORIENTED_EDGE('',*,*,#9466,.T.);
#12745=ORIENTED_EDGE('',*,*,#9467,.F.);
#12746=ORIENTED_EDGE('',*,*,#9468,.T.);
#12747=ORIENTED_EDGE('',*,*,#9327,.F.);
#12748=ORIENTED_EDGE('',*,*,#9468,.F.);
#12749=ORIENTED_EDGE('',*,*,#9469,.F.);
#12750=ORIENTED_EDGE('',*,*,#9470,.F.);
#12751=ORIENTED_EDGE('',*,*,#9328,.F.);
#12752=ORIENTED_EDGE('',*,*,#9470,.T.);
#12753=ORIENTED_EDGE('',*,*,#9471,.F.);
#12754=ORIENTED_EDGE('',*,*,#9472,.F.);
#12755=ORIENTED_EDGE('',*,*,#9329,.F.);
#12756=ORIENTED_EDGE('',*,*,#9472,.T.);
#12757=ORIENTED_EDGE('',*,*,#9473,.F.);
#12758=ORIENTED_EDGE('',*,*,#9474,.F.);
#12759=ORIENTED_EDGE('',*,*,#9330,.F.);
#12760=ORIENTED_EDGE('',*,*,#9474,.T.);
#12761=ORIENTED_EDGE('',*,*,#9475,.F.);
#12762=ORIENTED_EDGE('',*,*,#9476,.T.);
#12763=ORIENTED_EDGE('',*,*,#9331,.F.);
#12764=ORIENTED_EDGE('',*,*,#9476,.F.);
#12765=ORIENTED_EDGE('',*,*,#9477,.F.);
#12766=ORIENTED_EDGE('',*,*,#9478,.F.);
#12767=ORIENTED_EDGE('',*,*,#9332,.F.);
#12768=ORIENTED_EDGE('',*,*,#9478,.T.);
#12769=ORIENTED_EDGE('',*,*,#9479,.F.);
#12770=ORIENTED_EDGE('',*,*,#9480,.F.);
#12771=ORIENTED_EDGE('',*,*,#9333,.F.);
#12772=ORIENTED_EDGE('',*,*,#9480,.T.);
#12773=ORIENTED_EDGE('',*,*,#9481,.F.);
#12774=ORIENTED_EDGE('',*,*,#9482,.F.);
#12775=ORIENTED_EDGE('',*,*,#9334,.F.);
#12776=ORIENTED_EDGE('',*,*,#9482,.T.);
#12777=ORIENTED_EDGE('',*,*,#9483,.F.);
#12778=ORIENTED_EDGE('',*,*,#9484,.T.);
#12779=ORIENTED_EDGE('',*,*,#9335,.F.);
#12780=ORIENTED_EDGE('',*,*,#9484,.F.);
#12781=ORIENTED_EDGE('',*,*,#9485,.F.);
#12782=ORIENTED_EDGE('',*,*,#9486,.F.);
#12783=ORIENTED_EDGE('',*,*,#9336,.F.);
#12784=ORIENTED_EDGE('',*,*,#9486,.T.);
#12785=ORIENTED_EDGE('',*,*,#9487,.F.);
#12786=ORIENTED_EDGE('',*,*,#9488,.F.);
#12787=ORIENTED_EDGE('',*,*,#9337,.F.);
#12788=ORIENTED_EDGE('',*,*,#9488,.T.);
#12789=ORIENTED_EDGE('',*,*,#9489,.F.);
#12790=ORIENTED_EDGE('',*,*,#9490,.F.);
#12791=ORIENTED_EDGE('',*,*,#9338,.F.);
#12792=ORIENTED_EDGE('',*,*,#9490,.T.);
#12793=ORIENTED_EDGE('',*,*,#9491,.F.);
#12794=ORIENTED_EDGE('',*,*,#9492,.T.);
#12795=ORIENTED_EDGE('',*,*,#9339,.F.);
#12796=ORIENTED_EDGE('',*,*,#9492,.F.);
#12797=ORIENTED_EDGE('',*,*,#9493,.F.);
#12798=ORIENTED_EDGE('',*,*,#9494,.F.);
#12799=ORIENTED_EDGE('',*,*,#9340,.F.);
#12800=ORIENTED_EDGE('',*,*,#9494,.T.);
#12801=ORIENTED_EDGE('',*,*,#9495,.F.);
#12802=ORIENTED_EDGE('',*,*,#9496,.F.);
#12803=ORIENTED_EDGE('',*,*,#9341,.F.);
#12804=ORIENTED_EDGE('',*,*,#9496,.T.);
#12805=ORIENTED_EDGE('',*,*,#9497,.F.);
#12806=ORIENTED_EDGE('',*,*,#9498,.F.);
#12807=ORIENTED_EDGE('',*,*,#9342,.F.);
#12808=ORIENTED_EDGE('',*,*,#9498,.T.);
#12809=ORIENTED_EDGE('',*,*,#9499,.F.);
#12810=ORIENTED_EDGE('',*,*,#9500,.T.);
#12811=ORIENTED_EDGE('',*,*,#9343,.F.);
#12812=ORIENTED_EDGE('',*,*,#9500,.F.);
#12813=ORIENTED_EDGE('',*,*,#9501,.F.);
#12814=ORIENTED_EDGE('',*,*,#9502,.F.);
#12815=ORIENTED_EDGE('',*,*,#9344,.F.);
#12816=ORIENTED_EDGE('',*,*,#9502,.T.);
#12817=ORIENTED_EDGE('',*,*,#9503,.F.);
#12818=ORIENTED_EDGE('',*,*,#9504,.F.);
#12819=ORIENTED_EDGE('',*,*,#9345,.F.);
#12820=ORIENTED_EDGE('',*,*,#9504,.T.);
#12821=ORIENTED_EDGE('',*,*,#9505,.F.);
#12822=ORIENTED_EDGE('',*,*,#9506,.F.);
#12823=ORIENTED_EDGE('',*,*,#9346,.F.);
#12824=ORIENTED_EDGE('',*,*,#9506,.T.);
#12825=ORIENTED_EDGE('',*,*,#9507,.F.);
#12826=ORIENTED_EDGE('',*,*,#9508,.T.);
#12827=ORIENTED_EDGE('',*,*,#9347,.F.);
#12828=ORIENTED_EDGE('',*,*,#9508,.F.);
#12829=ORIENTED_EDGE('',*,*,#9509,.F.);
#12830=ORIENTED_EDGE('',*,*,#9510,.F.);
#12831=ORIENTED_EDGE('',*,*,#9348,.F.);
#12832=ORIENTED_EDGE('',*,*,#9510,.T.);
#12833=ORIENTED_EDGE('',*,*,#9511,.F.);
#12834=ORIENTED_EDGE('',*,*,#9512,.F.);
#12835=ORIENTED_EDGE('',*,*,#9349,.F.);
#12836=ORIENTED_EDGE('',*,*,#9512,.T.);
#12837=ORIENTED_EDGE('',*,*,#9513,.F.);
#12838=ORIENTED_EDGE('',*,*,#9514,.F.);
#12839=ORIENTED_EDGE('',*,*,#9350,.F.);
#12840=ORIENTED_EDGE('',*,*,#9514,.T.);
#12841=ORIENTED_EDGE('',*,*,#9515,.F.);
#12842=ORIENTED_EDGE('',*,*,#9516,.T.);
#12843=ORIENTED_EDGE('',*,*,#9351,.F.);
#12844=ORIENTED_EDGE('',*,*,#9516,.F.);
#12845=ORIENTED_EDGE('',*,*,#9517,.F.);
#12846=ORIENTED_EDGE('',*,*,#9518,.F.);
#12847=ORIENTED_EDGE('',*,*,#9352,.F.);
#12848=ORIENTED_EDGE('',*,*,#9518,.T.);
#12849=ORIENTED_EDGE('',*,*,#9519,.F.);
#12850=ORIENTED_EDGE('',*,*,#9520,.F.);
#12851=ORIENTED_EDGE('',*,*,#9353,.F.);
#12852=ORIENTED_EDGE('',*,*,#9520,.T.);
#12853=ORIENTED_EDGE('',*,*,#9521,.F.);
#12854=ORIENTED_EDGE('',*,*,#9522,.F.);
#12855=ORIENTED_EDGE('',*,*,#9354,.F.);
#12856=ORIENTED_EDGE('',*,*,#9523,.T.);
#12857=ORIENTED_EDGE('',*,*,#9521,.T.);
#12858=ORIENTED_EDGE('',*,*,#9519,.T.);
#12859=ORIENTED_EDGE('',*,*,#9517,.T.);
#12860=ORIENTED_EDGE('',*,*,#9515,.T.);
#12861=ORIENTED_EDGE('',*,*,#9513,.T.);
#12862=ORIENTED_EDGE('',*,*,#9511,.T.);
#12863=ORIENTED_EDGE('',*,*,#9509,.T.);
#12864=ORIENTED_EDGE('',*,*,#9507,.T.);
#12865=ORIENTED_EDGE('',*,*,#9505,.T.);
#12866=ORIENTED_EDGE('',*,*,#9503,.T.);
#12867=ORIENTED_EDGE('',*,*,#9501,.T.);
#12868=ORIENTED_EDGE('',*,*,#9499,.T.);
#12869=ORIENTED_EDGE('',*,*,#9497,.T.);
#12870=ORIENTED_EDGE('',*,*,#9495,.T.);
#12871=ORIENTED_EDGE('',*,*,#9493,.T.);
#12872=ORIENTED_EDGE('',*,*,#9491,.T.);
#12873=ORIENTED_EDGE('',*,*,#9489,.T.);
#12874=ORIENTED_EDGE('',*,*,#9487,.T.);
#12875=ORIENTED_EDGE('',*,*,#9485,.T.);
#12876=ORIENTED_EDGE('',*,*,#9483,.T.);
#12877=ORIENTED_EDGE('',*,*,#9481,.T.);
#12878=ORIENTED_EDGE('',*,*,#9479,.T.);
#12879=ORIENTED_EDGE('',*,*,#9477,.T.);
#12880=ORIENTED_EDGE('',*,*,#9475,.T.);
#12881=ORIENTED_EDGE('',*,*,#9473,.T.);
#12882=ORIENTED_EDGE('',*,*,#9471,.T.);
#12883=ORIENTED_EDGE('',*,*,#9469,.T.);
#12884=ORIENTED_EDGE('',*,*,#9467,.T.);
#12885=ORIENTED_EDGE('',*,*,#9465,.T.);
#12886=ORIENTED_EDGE('',*,*,#9463,.T.);
#12887=ORIENTED_EDGE('',*,*,#9461,.T.);
#12888=ORIENTED_EDGE('',*,*,#9459,.T.);
#12889=ORIENTED_EDGE('',*,*,#9457,.T.);
#12890=ORIENTED_EDGE('',*,*,#9455,.T.);
#12891=ORIENTED_EDGE('',*,*,#9453,.T.);
#12892=ORIENTED_EDGE('',*,*,#9451,.T.);
#12893=ORIENTED_EDGE('',*,*,#9449,.T.);
#12894=ORIENTED_EDGE('',*,*,#9447,.T.);
#12895=ORIENTED_EDGE('',*,*,#9445,.T.);
#12896=ORIENTED_EDGE('',*,*,#9443,.T.);
#12897=ORIENTED_EDGE('',*,*,#9441,.T.);
#12898=ORIENTED_EDGE('',*,*,#9439,.T.);
#12899=ORIENTED_EDGE('',*,*,#9437,.T.);
#12900=ORIENTED_EDGE('',*,*,#9435,.T.);
#12901=ORIENTED_EDGE('',*,*,#9433,.T.);
#12902=ORIENTED_EDGE('',*,*,#9431,.T.);
#12903=ORIENTED_EDGE('',*,*,#9429,.T.);
#12904=ORIENTED_EDGE('',*,*,#9427,.T.);
#12905=ORIENTED_EDGE('',*,*,#9425,.T.);
#12906=ORIENTED_EDGE('',*,*,#9423,.T.);
#12907=ORIENTED_EDGE('',*,*,#9421,.T.);
#12908=ORIENTED_EDGE('',*,*,#9419,.T.);
#12909=ORIENTED_EDGE('',*,*,#9417,.T.);
#12910=ORIENTED_EDGE('',*,*,#9415,.T.);
#12911=ORIENTED_EDGE('',*,*,#9413,.T.);
#12912=ORIENTED_EDGE('',*,*,#9411,.T.);
#12913=ORIENTED_EDGE('',*,*,#9409,.T.);
#12914=ORIENTED_EDGE('',*,*,#9407,.T.);
#12915=ORIENTED_EDGE('',*,*,#9405,.T.);
#12916=ORIENTED_EDGE('',*,*,#9403,.T.);
#12917=ORIENTED_EDGE('',*,*,#9401,.T.);
#12918=ORIENTED_EDGE('',*,*,#9399,.T.);
#12919=ORIENTED_EDGE('',*,*,#9397,.T.);
#12920=ORIENTED_EDGE('',*,*,#9395,.T.);
#12921=ORIENTED_EDGE('',*,*,#9393,.T.);
#12922=ORIENTED_EDGE('',*,*,#9391,.T.);
#12923=ORIENTED_EDGE('',*,*,#9389,.T.);
#12924=ORIENTED_EDGE('',*,*,#9387,.T.);
#12925=ORIENTED_EDGE('',*,*,#9385,.T.);
#12926=ORIENTED_EDGE('',*,*,#9383,.T.);
#12927=ORIENTED_EDGE('',*,*,#9381,.T.);
#12928=ORIENTED_EDGE('',*,*,#9379,.T.);
#12929=ORIENTED_EDGE('',*,*,#9377,.T.);
#12930=ORIENTED_EDGE('',*,*,#9375,.T.);
#12931=ORIENTED_EDGE('',*,*,#9373,.T.);
#12932=ORIENTED_EDGE('',*,*,#9371,.T.);
#12933=ORIENTED_EDGE('',*,*,#9369,.T.);
#12934=ORIENTED_EDGE('',*,*,#9367,.T.);
#12935=ORIENTED_EDGE('',*,*,#9365,.T.);
#12936=ORIENTED_EDGE('',*,*,#9363,.T.);
#12937=ORIENTED_EDGE('',*,*,#9364,.T.);
#12938=ORIENTED_EDGE('',*,*,#9355,.F.);
#12939=ORIENTED_EDGE('',*,*,#9522,.T.);
#12940=ORIENTED_EDGE('',*,*,#9523,.F.);
#15090=CYLINDRICAL_SURFACE('',#17870,0.6);
#15091=CYLINDRICAL_SURFACE('',#17872,1.4);
#15092=CYLINDRICAL_SURFACE('',#17877,1.75);
#15093=CYLINDRICAL_SURFACE('',#17880,1.75);
#15094=CYLINDRICAL_SURFACE('',#17883,1.75);
#15095=CYLINDRICAL_SURFACE('',#17886,1.75);
#15096=CYLINDRICAL_SURFACE('',#17889,1.75);
#15097=CYLINDRICAL_SURFACE('',#17892,1.75);
#15098=CYLINDRICAL_SURFACE('',#17895,1.75);
#15099=CYLINDRICAL_SURFACE('',#17898,1.75);
#15100=CYLINDRICAL_SURFACE('',#17901,1.75);
#15101=CYLINDRICAL_SURFACE('',#17904,1.75);
#15102=CYLINDRICAL_SURFACE('',#17907,1.75);
#15103=CYLINDRICAL_SURFACE('',#17910,1.75);
#15104=CYLINDRICAL_SURFACE('',#17913,1.75);
#15105=CYLINDRICAL_SURFACE('',#17916,1.75);
#15106=CYLINDRICAL_SURFACE('',#17919,1.75);
#15107=CYLINDRICAL_SURFACE('',#17922,1.75);
#15108=CYLINDRICAL_SURFACE('',#17925,1.75);
#15109=CYLINDRICAL_SURFACE('',#17928,1.75);
#15110=CYLINDRICAL_SURFACE('',#17931,1.75);
#15111=CYLINDRICAL_SURFACE('',#17936,1.75);
#15661=ADVANCED_FACE('',(#2454),#1822,.F.);
#15662=ADVANCED_FACE('',(#2455),#1823,.F.);
#15663=ADVANCED_FACE('',(#2456),#1824,.F.);
#15664=ADVANCED_FACE('',(#2457,#1555),#1825,.F.);
#15665=ADVANCED_FACE('',(#2458),#15090,.F.);
#15666=ADVANCED_FACE('',(#2459),#15091,.T.);
#15667=ADVANCED_FACE('',(#2460,#1556),#1826,.T.);
#15668=ADVANCED_FACE('',(#2461),#11,.T.);
#15669=ADVANCED_FACE('',(#2462),#1827,.T.);
#15670=ADVANCED_FACE('',(#2463),#12,.T.);
#15671=ADVANCED_FACE('',(#2464),#15092,.T.);
#15672=ADVANCED_FACE('',(#2465),#13,.T.);
#15673=ADVANCED_FACE('',(#2466),#1828,.T.);
#15674=ADVANCED_FACE('',(#2467),#14,.T.);
#15675=ADVANCED_FACE('',(#2468),#15093,.T.);
#15676=ADVANCED_FACE('',(#2469),#15,.T.);
#15677=ADVANCED_FACE('',(#2470),#1829,.T.);
#15678=ADVANCED_FACE('',(#2471),#16,.T.);
#15679=ADVANCED_FACE('',(#2472),#15094,.T.);
#15680=ADVANCED_FACE('',(#2473),#17,.T.);
#15681=ADVANCED_FACE('',(#2474),#1830,.T.);
#15682=ADVANCED_FACE('',(#2475),#18,.T.);
#15683=ADVANCED_FACE('',(#2476),#15095,.T.);
#15684=ADVANCED_FACE('',(#2477),#19,.T.);
#15685=ADVANCED_FACE('',(#2478),#1831,.T.);
#15686=ADVANCED_FACE('',(#2479),#20,.T.);
#15687=ADVANCED_FACE('',(#2480),#15096,.T.);
#15688=ADVANCED_FACE('',(#2481),#21,.T.);
#15689=ADVANCED_FACE('',(#2482),#1832,.T.);
#15690=ADVANCED_FACE('',(#2483),#22,.T.);
#15691=ADVANCED_FACE('',(#2484),#15097,.T.);
#15692=ADVANCED_FACE('',(#2485),#23,.T.);
#15693=ADVANCED_FACE('',(#2486),#1833,.T.);
#15694=ADVANCED_FACE('',(#2487),#24,.T.);
#15695=ADVANCED_FACE('',(#2488),#15098,.T.);
#15696=ADVANCED_FACE('',(#2489),#25,.T.);
#15697=ADVANCED_FACE('',(#2490),#1834,.T.);
#15698=ADVANCED_FACE('',(#2491),#26,.T.);
#15699=ADVANCED_FACE('',(#2492),#15099,.T.);
#15700=ADVANCED_FACE('',(#2493),#27,.T.);
#15701=ADVANCED_FACE('',(#2494),#1835,.T.);
#15702=ADVANCED_FACE('',(#2495),#28,.T.);
#15703=ADVANCED_FACE('',(#2496),#15100,.T.);
#15704=ADVANCED_FACE('',(#2497),#29,.T.);
#15705=ADVANCED_FACE('',(#2498),#1836,.T.);
#15706=ADVANCED_FACE('',(#2499),#30,.T.);
#15707=ADVANCED_FACE('',(#2500),#15101,.T.);
#15708=ADVANCED_FACE('',(#2501),#31,.T.);
#15709=ADVANCED_FACE('',(#2502),#1837,.T.);
#15710=ADVANCED_FACE('',(#2503),#32,.T.);
#15711=ADVANCED_FACE('',(#2504),#15102,.T.);
#15712=ADVANCED_FACE('',(#2505),#33,.T.);
#15713=ADVANCED_FACE('',(#2506),#1838,.T.);
#15714=ADVANCED_FACE('',(#2507),#34,.T.);
#15715=ADVANCED_FACE('',(#2508),#15103,.T.);
#15716=ADVANCED_FACE('',(#2509),#35,.T.);
#15717=ADVANCED_FACE('',(#2510),#1839,.T.);
#15718=ADVANCED_FACE('',(#2511),#36,.T.);
#15719=ADVANCED_FACE('',(#2512),#15104,.T.);
#15720=ADVANCED_FACE('',(#2513),#37,.T.);
#15721=ADVANCED_FACE('',(#2514),#1840,.T.);
#15722=ADVANCED_FACE('',(#2515),#38,.T.);
#15723=ADVANCED_FACE('',(#2516),#15105,.T.);
#15724=ADVANCED_FACE('',(#2517),#39,.T.);
#15725=ADVANCED_FACE('',(#2518),#1841,.T.);
#15726=ADVANCED_FACE('',(#2519),#40,.T.);
#15727=ADVANCED_FACE('',(#2520),#15106,.T.);
#15728=ADVANCED_FACE('',(#2521),#41,.T.);
#15729=ADVANCED_FACE('',(#2522),#1842,.T.);
#15730=ADVANCED_FACE('',(#2523),#42,.T.);
#15731=ADVANCED_FACE('',(#2524),#15107,.T.);
#15732=ADVANCED_FACE('',(#2525),#43,.T.);
#15733=ADVANCED_FACE('',(#2526),#1843,.T.);
#15734=ADVANCED_FACE('',(#2527),#44,.T.);
#15735=ADVANCED_FACE('',(#2528),#15108,.T.);
#15736=ADVANCED_FACE('',(#2529),#45,.T.);
#15737=ADVANCED_FACE('',(#2530),#1844,.T.);
#15738=ADVANCED_FACE('',(#2531),#46,.T.);
#15739=ADVANCED_FACE('',(#2532),#15109,.T.);
#15740=ADVANCED_FACE('',(#2533),#47,.T.);
#15741=ADVANCED_FACE('',(#2534),#1845,.T.);
#15742=ADVANCED_FACE('',(#2535),#48,.T.);
#15743=ADVANCED_FACE('',(#2536),#15110,.T.);
#15744=ADVANCED_FACE('',(#2537),#49,.T.);
#15745=ADVANCED_FACE('',(#2538),#1846,.T.);
#15746=ADVANCED_FACE('',(#2539),#50,.T.);
#15747=ADVANCED_FACE('',(#2540,#1557),#1847,.T.);
#15748=ADVANCED_FACE('',(#2541),#15111,.T.);
#16174=CLOSED_SHELL('',(#15661,#15662,#15663,#15664,#15665,#15666,#15667,
#15668,#15669,#15670,#15671,#15672,#15673,#15674,#15675,#15676,#15677,#15678,
#15679,#15680,#15681,#15682,#15683,#15684,#15685,#15686,#15687,#15688,#15689,
#15690,#15691,#15692,#15693,#15694,#15695,#15696,#15697,#15698,#15699,#15700,
#15701,#15702,#15703,#15704,#15705,#15706,#15707,#15708,#15709,#15710,#15711,
#15712,#15713,#15714,#15715,#15716,#15717,#15718,#15719,#15720,#15721,#15722,
#15723,#15724,#15725,#15726,#15727,#15728,#15729,#15730,#15731,#15732,#15733,
#15734,#15735,#15736,#15737,#15738,#15739,#15740,#15741,#15742,#15743,#15744,
#15745,#15746,#15747,#15748));
#17844=AXIS2_PLACEMENT_3D('',#25691,#20974,#20975);
#17845=AXIS2_PLACEMENT_3D('',#25692,#20976,#20977);
#17846=AXIS2_PLACEMENT_3D('',#25701,#20982,#20983);
#17847=AXIS2_PLACEMENT_3D('',#25707,#20987,#20988);
#17848=AXIS2_PLACEMENT_3D('',#25713,#20992,#20993);
#17849=AXIS2_PLACEMENT_3D('',#25716,#20994,#20995);
#17850=AXIS2_PLACEMENT_3D('',#25862,#20997,#20998);
#17851=AXIS2_PLACEMENT_3D('',#26008,#21000,#21001);
#17852=AXIS2_PLACEMENT_3D('',#26154,#21003,#21004);
#17853=AXIS2_PLACEMENT_3D('',#26300,#21006,#21007);
#17854=AXIS2_PLACEMENT_3D('',#26446,#21009,#21010);
#17855=AXIS2_PLACEMENT_3D('',#26592,#21012,#21013);
#17856=AXIS2_PLACEMENT_3D('',#26738,#21015,#21016);
#17857=AXIS2_PLACEMENT_3D('',#26884,#21018,#21019);
#17858=AXIS2_PLACEMENT_3D('',#27030,#21021,#21022);
#17859=AXIS2_PLACEMENT_3D('',#27176,#21024,#21025);
#17860=AXIS2_PLACEMENT_3D('',#27322,#21027,#21028);
#17861=AXIS2_PLACEMENT_3D('',#27468,#21030,#21031);
#17862=AXIS2_PLACEMENT_3D('',#27614,#21033,#21034);
#17863=AXIS2_PLACEMENT_3D('',#27760,#21036,#21037);
#17864=AXIS2_PLACEMENT_3D('',#27906,#21039,#21040);
#17865=AXIS2_PLACEMENT_3D('',#28052,#21042,#21043);
#17866=AXIS2_PLACEMENT_3D('',#28198,#21045,#21046);
#17867=AXIS2_PLACEMENT_3D('',#28344,#21048,#21049);
#17868=AXIS2_PLACEMENT_3D('',#28490,#21051,#21052);
#17869=AXIS2_PLACEMENT_3D('',#28634,#21054,#21055);
#17870=AXIS2_PLACEMENT_3D('',#28635,#21056,#21057);
#17871=AXIS2_PLACEMENT_3D('',#28636,#21058,#21059);
#17872=AXIS2_PLACEMENT_3D('',#28637,#21060,#21061);
#17873=AXIS2_PLACEMENT_3D('',#28639,#21062,#21063);
#17874=AXIS2_PLACEMENT_3D('',#28642,#21065,#21066);
#17875=AXIS2_PLACEMENT_3D('',#28643,#21067,#21068);
#17876=AXIS2_PLACEMENT_3D('',#28858,#21071,#21072);
#17877=AXIS2_PLACEMENT_3D('',#29074,#21076,#21077);
#17878=AXIS2_PLACEMENT_3D('',#29076,#21078,#21079);
#17879=AXIS2_PLACEMENT_3D('',#29290,#21082,#21083);
#17880=AXIS2_PLACEMENT_3D('',#29506,#21087,#21088);
#17881=AXIS2_PLACEMENT_3D('',#29508,#21089,#21090);
#17882=AXIS2_PLACEMENT_3D('',#29722,#21093,#21094);
#17883=AXIS2_PLACEMENT_3D('',#29938,#21098,#21099);
#17884=AXIS2_PLACEMENT_3D('',#29940,#21100,#21101);
#17885=AXIS2_PLACEMENT_3D('',#30154,#21104,#21105);
#17886=AXIS2_PLACEMENT_3D('',#30370,#21109,#21110);
#17887=AXIS2_PLACEMENT_3D('',#30372,#21111,#21112);
#17888=AXIS2_PLACEMENT_3D('',#30586,#21115,#21116);
#17889=AXIS2_PLACEMENT_3D('',#30802,#21120,#21121);
#17890=AXIS2_PLACEMENT_3D('',#30804,#21122,#21123);
#17891=AXIS2_PLACEMENT_3D('',#31018,#21126,#21127);
#17892=AXIS2_PLACEMENT_3D('',#31234,#21131,#21132);
#17893=AXIS2_PLACEMENT_3D('',#31236,#21133,#21134);
#17894=AXIS2_PLACEMENT_3D('',#31450,#21137,#21138);
#17895=AXIS2_PLACEMENT_3D('',#31666,#21142,#21143);
#17896=AXIS2_PLACEMENT_3D('',#31668,#21144,#21145);
#17897=AXIS2_PLACEMENT_3D('',#31882,#21148,#21149);
#17898=AXIS2_PLACEMENT_3D('',#32098,#21153,#21154);
#17899=AXIS2_PLACEMENT_3D('',#32100,#21155,#21156);
#17900=AXIS2_PLACEMENT_3D('',#32314,#21159,#21160);
#17901=AXIS2_PLACEMENT_3D('',#32530,#21164,#21165);
#17902=AXIS2_PLACEMENT_3D('',#32532,#21166,#21167);
#17903=AXIS2_PLACEMENT_3D('',#32746,#21170,#21171);
#17904=AXIS2_PLACEMENT_3D('',#32962,#21175,#21176);
#17905=AXIS2_PLACEMENT_3D('',#32964,#21177,#21178);
#17906=AXIS2_PLACEMENT_3D('',#33178,#21181,#21182);
#17907=AXIS2_PLACEMENT_3D('',#33394,#21186,#21187);
#17908=AXIS2_PLACEMENT_3D('',#33396,#21188,#21189);
#17909=AXIS2_PLACEMENT_3D('',#33610,#21192,#21193);
#17910=AXIS2_PLACEMENT_3D('',#33826,#21197,#21198);
#17911=AXIS2_PLACEMENT_3D('',#33828,#21199,#21200);
#17912=AXIS2_PLACEMENT_3D('',#34042,#21203,#21204);
#17913=AXIS2_PLACEMENT_3D('',#34258,#21208,#21209);
#17914=AXIS2_PLACEMENT_3D('',#34260,#21210,#21211);
#17915=AXIS2_PLACEMENT_3D('',#34474,#21214,#21215);
#17916=AXIS2_PLACEMENT_3D('',#34690,#21219,#21220);
#17917=AXIS2_PLACEMENT_3D('',#34692,#21221,#21222);
#17918=AXIS2_PLACEMENT_3D('',#34906,#21225,#21226);
#17919=AXIS2_PLACEMENT_3D('',#35122,#21230,#21231);
#17920=AXIS2_PLACEMENT_3D('',#35124,#21232,#21233);
#17921=AXIS2_PLACEMENT_3D('',#35338,#21236,#21237);
#17922=AXIS2_PLACEMENT_3D('',#35554,#21241,#21242);
#17923=AXIS2_PLACEMENT_3D('',#35556,#21243,#21244);
#17924=AXIS2_PLACEMENT_3D('',#35770,#21247,#21248);
#17925=AXIS2_PLACEMENT_3D('',#35986,#21252,#21253);
#17926=AXIS2_PLACEMENT_3D('',#35988,#21254,#21255);
#17927=AXIS2_PLACEMENT_3D('',#36202,#21258,#21259);
#17928=AXIS2_PLACEMENT_3D('',#36418,#21263,#21264);
#17929=AXIS2_PLACEMENT_3D('',#36420,#21265,#21266);
#17930=AXIS2_PLACEMENT_3D('',#36634,#21269,#21270);
#17931=AXIS2_PLACEMENT_3D('',#36850,#21274,#21275);
#17932=AXIS2_PLACEMENT_3D('',#36852,#21276,#21277);
#17933=AXIS2_PLACEMENT_3D('',#37066,#21280,#21281);
#17934=AXIS2_PLACEMENT_3D('',#37282,#21285,#21286);
#17935=AXIS2_PLACEMENT_3D('',#37283,#21287,#21288);
#17936=AXIS2_PLACEMENT_3D('',#37284,#21289,#21290);
#20974=DIRECTION('axis',(0.,0.,1.));
#20975=DIRECTION('refdir',(1.,0.,0.));
#20976=DIRECTION('center_axis',(1.,0.,0.));
#20977=DIRECTION('ref_axis',(0.,0.,-1.));
#20978=DIRECTION('',(0.,0.,1.));
#20979=DIRECTION('',(0.,1.,0.));
#20980=DIRECTION('',(0.,0.,-1.));
#20981=DIRECTION('',(0.,-1.,0.));
#20982=DIRECTION('center_axis',(0.,0.,-1.));
#20983=DIRECTION('ref_axis',(-1.,0.,0.));
#20984=DIRECTION('',(1.,0.,0.));
#20985=DIRECTION('',(0.,-1.,0.));
#20986=DIRECTION('',(-1.,0.,0.));
#20987=DIRECTION('center_axis',(-1.,0.,0.));
#20988=DIRECTION('ref_axis',(0.,0.,1.));
#20989=DIRECTION('',(0.,0.,-1.));
#20990=DIRECTION('',(0.,1.,0.));
#20991=DIRECTION('',(0.,0.,1.));
#20992=DIRECTION('center_axis',(0.,1.,0.));
#20993=DIRECTION('ref_axis',(1.,0.,0.));
#20994=DIRECTION('center_axis',(0.,-1.,0.));
#20995=DIRECTION('ref_axis',(1.,0.,0.));
#20996=DIRECTION('',(-0.587785252292473,0.,0.809016994374947));
#20997=DIRECTION('center_axis',(0.,-1.,0.));
#20998=DIRECTION('ref_axis',(1.,0.,0.));
#20999=DIRECTION('',(-0.809016994374948,0.,0.587785252292473));
#21000=DIRECTION('center_axis',(0.,-1.,0.));
#21001=DIRECTION('ref_axis',(1.,0.,0.));
#21002=DIRECTION('',(-0.951056516295154,0.,0.309016994374947));
#21003=DIRECTION('center_axis',(0.,-1.,0.));
#21004=DIRECTION('ref_axis',(1.,0.,0.));
#21005=DIRECTION('',(-1.,0.,-1.83697019872103E-16));
#21006=DIRECTION('center_axis',(0.,-1.,0.));
#21007=DIRECTION('ref_axis',(1.,0.,0.));
#21008=DIRECTION('',(-0.951056516295154,0.,-0.309016994374948));
#21009=DIRECTION('center_axis',(0.,-1.,0.));
#21010=DIRECTION('ref_axis',(1.,0.,0.));
#21011=DIRECTION('',(-0.809016994374947,0.,-0.587785252292473));
#21012=DIRECTION('center_axis',(0.,-1.,0.));
#21013=DIRECTION('ref_axis',(1.,0.,0.));
#21014=DIRECTION('',(-0.587785252292473,0.,-0.809016994374948));
#21015=DIRECTION('center_axis',(0.,-1.,0.));
#21016=DIRECTION('ref_axis',(1.,0.,0.));
#21017=DIRECTION('',(-0.309016994374947,0.,-0.951056516295154));
#21018=DIRECTION('center_axis',(0.,-1.,0.));
#21019=DIRECTION('ref_axis',(1.,0.,0.));
#21020=DIRECTION('',(1.22464679914735E-16,0.,-1.));
#21021=DIRECTION('center_axis',(0.,-1.,0.));
#21022=DIRECTION('ref_axis',(1.,0.,0.));
#21023=DIRECTION('',(0.309016994374948,0.,-0.951056516295154));
#21024=DIRECTION('center_axis',(0.,-1.,0.));
#21025=DIRECTION('ref_axis',(1.,0.,0.));
#21026=DIRECTION('',(0.587785252292473,0.,-0.809016994374947));
#21027=DIRECTION('center_axis',(0.,-1.,0.));
#21028=DIRECTION('ref_axis',(1.,0.,0.));
#21029=DIRECTION('',(0.809016994374948,0.,-0.587785252292473));
#21030=DIRECTION('center_axis',(0.,-1.,0.));
#21031=DIRECTION('ref_axis',(1.,0.,0.));
#21032=DIRECTION('',(0.951056516295154,0.,-0.309016994374947));
#21033=DIRECTION('center_axis',(0.,-1.,0.));
#21034=DIRECTION('ref_axis',(1.,0.,0.));
#21035=DIRECTION('',(1.,0.,6.12323399573677E-17));
#21036=DIRECTION('center_axis',(0.,-1.,0.));
#21037=DIRECTION('ref_axis',(1.,0.,0.));
#21038=DIRECTION('',(0.951056516295154,0.,0.309016994374948));
#21039=DIRECTION('center_axis',(0.,-1.,0.));
#21040=DIRECTION('ref_axis',(1.,0.,0.));
#21041=DIRECTION('',(0.809016994374947,0.,0.587785252292473));
#21042=DIRECTION('center_axis',(0.,-1.,0.));
#21043=DIRECTION('ref_axis',(1.,0.,0.));
#21044=DIRECTION('',(0.587785252292473,0.,0.809016994374947));
#21045=DIRECTION('center_axis',(0.,-1.,0.));
#21046=DIRECTION('ref_axis',(1.,0.,0.));
#21047=DIRECTION('',(0.309016994374947,0.,0.951056516295154));
#21048=DIRECTION('center_axis',(0.,-1.,0.));
#21049=DIRECTION('ref_axis',(1.,0.,0.));
#21050=DIRECTION('',(0.,0.,1.));
#21051=DIRECTION('center_axis',(0.,-1.,0.));
#21052=DIRECTION('ref_axis',(1.,0.,0.));
#21053=DIRECTION('',(-0.309016994374948,0.,0.951056516295154));
#21054=DIRECTION('center_axis',(0.,1.,0.));
#21055=DIRECTION('ref_axis',(1.,0.,0.));
#21056=DIRECTION('center_axis',(0.,1.,0.));
#21057=DIRECTION('ref_axis',(6.12323399573677E-17,0.,1.));
#21058=DIRECTION('center_axis',(0.,-1.,0.));
#21059=DIRECTION('ref_axis',(1.,0.,0.));
#21060=DIRECTION('center_axis',(0.,1.,0.));
#21061=DIRECTION('ref_axis',(1.,0.,0.));
#21062=DIRECTION('center_axis',(0.,1.,0.));
#21063=DIRECTION('ref_axis',(1.,0.,0.));
#21064=DIRECTION('',(0.,-1.,0.));
#21065=DIRECTION('center_axis',(0.,-1.,0.));
#21066=DIRECTION('ref_axis',(1.,0.,0.));
#21067=DIRECTION('center_axis',(0.,1.,0.));
#21068=DIRECTION('ref_axis',(1.,0.,0.));
#21069=DIRECTION('',(0.,-1.,0.));
#21070=DIRECTION('',(0.,1.,0.));
#21071=DIRECTION('center_axis',(0.951056516295154,0.,0.309016994374948));
#21072=DIRECTION('ref_axis',(0.309016994374948,0.,-0.951056516295154));
#21073=DIRECTION('',(0.309016994374948,0.,-0.951056516295154));
#21074=DIRECTION('',(0.,1.,0.));
#21075=DIRECTION('',(0.,1.,0.));
#21076=DIRECTION('center_axis',(0.,1.,0.));
#21077=DIRECTION('ref_axis',(1.,0.,0.));
#21078=DIRECTION('center_axis',(0.,1.,0.));
#21079=DIRECTION('ref_axis',(1.,0.,0.));
#21080=DIRECTION('',(0.,-1.,0.));
#21081=DIRECTION('',(0.,1.,0.));
#21082=DIRECTION('center_axis',(0.809016994374947,0.,0.587785252292473));
#21083=DIRECTION('ref_axis',(0.587785252292473,0.,-0.809016994374947));
#21084=DIRECTION('',(0.587785252292473,0.,-0.809016994374947));
#21085=DIRECTION('',(0.,1.,0.));
#21086=DIRECTION('',(0.,1.,0.));
#21087=DIRECTION('center_axis',(0.,1.,0.));
#21088=DIRECTION('ref_axis',(1.,0.,0.));
#21089=DIRECTION('center_axis',(0.,1.,0.));
#21090=DIRECTION('ref_axis',(1.,0.,0.));
#21091=DIRECTION('',(0.,-1.,0.));
#21092=DIRECTION('',(0.,1.,0.));
#21093=DIRECTION('center_axis',(0.587785252292473,0.,0.809016994374948));
#21094=DIRECTION('ref_axis',(0.809016994374948,0.,-0.587785252292473));
#21095=DIRECTION('',(0.809016994374948,0.,-0.587785252292473));
#21096=DIRECTION('',(0.,1.,0.));
#21097=DIRECTION('',(0.,1.,0.));
#21098=DIRECTION('center_axis',(0.,1.,0.));
#21099=DIRECTION('ref_axis',(1.,0.,0.));
#21100=DIRECTION('center_axis',(0.,1.,0.));
#21101=DIRECTION('ref_axis',(1.,0.,0.));
#21102=DIRECTION('',(0.,-1.,0.));
#21103=DIRECTION('',(0.,1.,0.));
#21104=DIRECTION('center_axis',(0.309016994374947,0.,0.951056516295154));
#21105=DIRECTION('ref_axis',(0.951056516295154,0.,-0.309016994374947));
#21106=DIRECTION('',(0.951056516295154,0.,-0.309016994374947));
#21107=DIRECTION('',(0.,1.,0.));
#21108=DIRECTION('',(0.,1.,0.));
#21109=DIRECTION('center_axis',(0.,1.,0.));
#21110=DIRECTION('ref_axis',(1.,0.,0.));
#21111=DIRECTION('center_axis',(0.,1.,0.));
#21112=DIRECTION('ref_axis',(1.,0.,0.));
#21113=DIRECTION('',(0.,-1.,0.));
#21114=DIRECTION('',(0.,1.,0.));
#21115=DIRECTION('center_axis',(-1.83697019872103E-16,0.,1.));
#21116=DIRECTION('ref_axis',(1.,0.,1.83697019872103E-16));
#21117=DIRECTION('',(1.,0.,1.83697019872103E-16));
#21118=DIRECTION('',(0.,1.,0.));
#21119=DIRECTION('',(0.,1.,0.));
#21120=DIRECTION('center_axis',(0.,1.,0.));
#21121=DIRECTION('ref_axis',(1.,0.,0.));
#21122=DIRECTION('center_axis',(0.,1.,0.));
#21123=DIRECTION('ref_axis',(1.,0.,0.));
#21124=DIRECTION('',(0.,-1.,0.));
#21125=DIRECTION('',(0.,1.,0.));
#21126=DIRECTION('center_axis',(-0.309016994374948,0.,0.951056516295154));
#21127=DIRECTION('ref_axis',(0.951056516295154,0.,0.309016994374948));
#21128=DIRECTION('',(0.951056516295154,0.,0.309016994374948));
#21129=DIRECTION('',(0.,1.,0.));
#21130=DIRECTION('',(0.,1.,0.));
#21131=DIRECTION('center_axis',(0.,1.,0.));
#21132=DIRECTION('ref_axis',(1.,0.,0.));
#21133=DIRECTION('center_axis',(0.,1.,0.));
#21134=DIRECTION('ref_axis',(1.,0.,0.));
#21135=DIRECTION('',(0.,-1.,0.));
#21136=DIRECTION('',(0.,1.,0.));
#21137=DIRECTION('center_axis',(-0.587785252292473,0.,0.809016994374947));
#21138=DIRECTION('ref_axis',(0.809016994374947,0.,0.587785252292473));
#21139=DIRECTION('',(0.809016994374947,0.,0.587785252292473));
#21140=DIRECTION('',(0.,1.,0.));
#21141=DIRECTION('',(0.,1.,0.));
#21142=DIRECTION('center_axis',(0.,1.,0.));
#21143=DIRECTION('ref_axis',(1.,0.,0.));
#21144=DIRECTION('center_axis',(0.,1.,0.));
#21145=DIRECTION('ref_axis',(1.,0.,0.));
#21146=DIRECTION('',(0.,-1.,0.));
#21147=DIRECTION('',(0.,1.,0.));
#21148=DIRECTION('center_axis',(-0.809016994374948,0.,0.587785252292473));
#21149=DIRECTION('ref_axis',(0.587785252292473,0.,0.809016994374948));
#21150=DIRECTION('',(0.587785252292473,0.,0.809016994374948));
#21151=DIRECTION('',(0.,1.,0.));
#21152=DIRECTION('',(0.,1.,0.));
#21153=DIRECTION('center_axis',(0.,1.,0.));
#21154=DIRECTION('ref_axis',(1.,0.,0.));
#21155=DIRECTION('center_axis',(0.,1.,0.));
#21156=DIRECTION('ref_axis',(1.,0.,0.));
#21157=DIRECTION('',(0.,-1.,0.));
#21158=DIRECTION('',(0.,1.,0.));
#21159=DIRECTION('center_axis',(-0.951056516295154,0.,0.309016994374947));
#21160=DIRECTION('ref_axis',(0.309016994374947,0.,0.951056516295154));
#21161=DIRECTION('',(0.309016994374947,0.,0.951056516295154));
#21162=DIRECTION('',(0.,1.,0.));
#21163=DIRECTION('',(0.,1.,0.));
#21164=DIRECTION('center_axis',(0.,1.,0.));
#21165=DIRECTION('ref_axis',(1.,0.,0.));
#21166=DIRECTION('center_axis',(0.,1.,0.));
#21167=DIRECTION('ref_axis',(1.,0.,0.));
#21168=DIRECTION('',(0.,-1.,0.));
#21169=DIRECTION('',(0.,1.,0.));
#21170=DIRECTION('center_axis',(-1.,0.,-1.22464679914735E-16));
#21171=DIRECTION('ref_axis',(-1.22464679914735E-16,0.,1.));
#21172=DIRECTION('',(-1.22464679914735E-16,0.,1.));
#21173=DIRECTION('',(0.,1.,0.));
#21174=DIRECTION('',(0.,1.,0.));
#21175=DIRECTION('center_axis',(0.,1.,0.));
#21176=DIRECTION('ref_axis',(1.,0.,0.));
#21177=DIRECTION('center_axis',(0.,1.,0.));
#21178=DIRECTION('ref_axis',(1.,0.,0.));
#21179=DIRECTION('',(0.,-1.,0.));
#21180=DIRECTION('',(0.,1.,0.));
#21181=DIRECTION('center_axis',(-0.951056516295154,0.,-0.309016994374948));
#21182=DIRECTION('ref_axis',(-0.309016994374948,0.,0.951056516295154));
#21183=DIRECTION('',(-0.309016994374948,0.,0.951056516295154));
#21184=DIRECTION('',(0.,1.,0.));
#21185=DIRECTION('',(0.,1.,0.));
#21186=DIRECTION('center_axis',(0.,1.,0.));
#21187=DIRECTION('ref_axis',(1.,0.,0.));
#21188=DIRECTION('center_axis',(0.,1.,0.));
#21189=DIRECTION('ref_axis',(1.,0.,0.));
#21190=DIRECTION('',(0.,-1.,0.));
#21191=DIRECTION('',(0.,1.,0.));
#21192=DIRECTION('center_axis',(-0.809016994374947,0.,-0.587785252292473));
#21193=DIRECTION('ref_axis',(-0.587785252292473,0.,0.809016994374947));
#21194=DIRECTION('',(-0.587785252292473,0.,0.809016994374947));
#21195=DIRECTION('',(0.,1.,0.));
#21196=DIRECTION('',(0.,1.,0.));
#21197=DIRECTION('center_axis',(0.,1.,0.));
#21198=DIRECTION('ref_axis',(1.,0.,0.));
#21199=DIRECTION('center_axis',(0.,1.,0.));
#21200=DIRECTION('ref_axis',(1.,0.,0.));
#21201=DIRECTION('',(0.,-1.,0.));
#21202=DIRECTION('',(0.,1.,0.));
#21203=DIRECTION('center_axis',(-0.587785252292473,0.,-0.809016994374948));
#21204=DIRECTION('ref_axis',(-0.809016994374948,0.,0.587785252292473));
#21205=DIRECTION('',(-0.809016994374948,0.,0.587785252292473));
#21206=DIRECTION('',(0.,1.,0.));
#21207=DIRECTION('',(0.,1.,0.));
#21208=DIRECTION('center_axis',(0.,1.,0.));
#21209=DIRECTION('ref_axis',(1.,0.,0.));
#21210=DIRECTION('center_axis',(0.,1.,0.));
#21211=DIRECTION('ref_axis',(1.,0.,0.));
#21212=DIRECTION('',(0.,-1.,0.));
#21213=DIRECTION('',(0.,1.,0.));
#21214=DIRECTION('center_axis',(-0.309016994374947,0.,-0.951056516295154));
#21215=DIRECTION('ref_axis',(-0.951056516295154,0.,0.309016994374947));
#21216=DIRECTION('',(-0.951056516295154,0.,0.309016994374947));
#21217=DIRECTION('',(0.,1.,0.));
#21218=DIRECTION('',(0.,1.,0.));
#21219=DIRECTION('center_axis',(0.,1.,0.));
#21220=DIRECTION('ref_axis',(1.,0.,0.));
#21221=DIRECTION('center_axis',(0.,1.,0.));
#21222=DIRECTION('ref_axis',(1.,0.,0.));
#21223=DIRECTION('',(0.,-1.,0.));
#21224=DIRECTION('',(0.,1.,0.));
#21225=DIRECTION('center_axis',(6.12323399573677E-17,0.,-1.));
#21226=DIRECTION('ref_axis',(-1.,0.,-6.12323399573677E-17));
#21227=DIRECTION('',(-1.,0.,-6.12323399573677E-17));
#21228=DIRECTION('',(0.,1.,0.));
#21229=DIRECTION('',(0.,1.,0.));
#21230=DIRECTION('center_axis',(0.,1.,0.));
#21231=DIRECTION('ref_axis',(1.,0.,0.));
#21232=DIRECTION('center_axis',(0.,1.,0.));
#21233=DIRECTION('ref_axis',(1.,0.,0.));
#21234=DIRECTION('',(0.,-1.,0.));
#21235=DIRECTION('',(0.,1.,0.));
#21236=DIRECTION('center_axis',(0.309016994374948,0.,-0.951056516295154));
#21237=DIRECTION('ref_axis',(-0.951056516295154,0.,-0.309016994374948));
#21238=DIRECTION('',(-0.951056516295154,0.,-0.309016994374948));
#21239=DIRECTION('',(0.,1.,0.));
#21240=DIRECTION('',(0.,1.,0.));
#21241=DIRECTION('center_axis',(0.,1.,0.));
#21242=DIRECTION('ref_axis',(1.,0.,0.));
#21243=DIRECTION('center_axis',(0.,1.,0.));
#21244=DIRECTION('ref_axis',(1.,0.,0.));
#21245=DIRECTION('',(0.,-1.,0.));
#21246=DIRECTION('',(0.,1.,0.));
#21247=DIRECTION('center_axis',(0.587785252292473,0.,-0.809016994374947));
#21248=DIRECTION('ref_axis',(-0.809016994374947,0.,-0.587785252292473));
#21249=DIRECTION('',(-0.809016994374947,0.,-0.587785252292473));
#21250=DIRECTION('',(0.,1.,0.));
#21251=DIRECTION('',(0.,1.,0.));
#21252=DIRECTION('center_axis',(0.,1.,0.));
#21253=DIRECTION('ref_axis',(1.,0.,0.));
#21254=DIRECTION('center_axis',(0.,1.,0.));
#21255=DIRECTION('ref_axis',(1.,0.,0.));
#21256=DIRECTION('',(0.,-1.,0.));
#21257=DIRECTION('',(0.,1.,0.));
#21258=DIRECTION('center_axis',(0.809016994374947,0.,-0.587785252292473));
#21259=DIRECTION('ref_axis',(-0.587785252292473,0.,-0.809016994374947));
#21260=DIRECTION('',(-0.587785252292473,0.,-0.809016994374947));
#21261=DIRECTION('',(0.,1.,0.));
#21262=DIRECTION('',(0.,1.,0.));
#21263=DIRECTION('center_axis',(0.,1.,0.));
#21264=DIRECTION('ref_axis',(1.,0.,0.));
#21265=DIRECTION('center_axis',(0.,1.,0.));
#21266=DIRECTION('ref_axis',(1.,0.,0.));
#21267=DIRECTION('',(0.,-1.,0.));
#21268=DIRECTION('',(0.,1.,0.));
#21269=DIRECTION('center_axis',(0.951056516295154,0.,-0.309016994374947));
#21270=DIRECTION('ref_axis',(-0.309016994374947,0.,-0.951056516295154));
#21271=DIRECTION('',(-0.309016994374947,0.,-0.951056516295154));
#21272=DIRECTION('',(0.,1.,0.));
#21273=DIRECTION('',(0.,1.,0.));
#21274=DIRECTION('center_axis',(0.,1.,0.));
#21275=DIRECTION('ref_axis',(1.,0.,0.));
#21276=DIRECTION('center_axis',(0.,1.,0.));
#21277=DIRECTION('ref_axis',(1.,0.,0.));
#21278=DIRECTION('',(0.,-1.,0.));
#21279=DIRECTION('',(0.,1.,0.));
#21280=DIRECTION('center_axis',(1.,0.,0.));
#21281=DIRECTION('ref_axis',(0.,0.,-1.));
#21282=DIRECTION('',(0.,0.,-1.));
#21283=DIRECTION('',(0.,1.,0.));
#21284=DIRECTION('',(0.,1.,0.));
#21285=DIRECTION('center_axis',(0.,1.,0.));
#21286=DIRECTION('ref_axis',(1.,0.,0.));
#21287=DIRECTION('center_axis',(0.,1.,0.));
#21288=DIRECTION('ref_axis',(1.,0.,0.));
#21289=DIRECTION('center_axis',(0.,1.,0.));
#21290=DIRECTION('ref_axis',(1.,0.,0.));
#25691=CARTESIAN_POINT('',(0.,0.,0.));
#25692=CARTESIAN_POINT('Origin',(0.2,0.,0.));
#25693=CARTESIAN_POINT('',(0.2,2.2,-0.78));
#25694=CARTESIAN_POINT('',(0.2,2.2,-0.565685424949238));
#25695=CARTESIAN_POINT('',(0.2,2.2,0.));
#25696=CARTESIAN_POINT('',(0.2,-1.,-0.78));
#25697=CARTESIAN_POINT('',(0.2,0.,-0.78));
#25698=CARTESIAN_POINT('',(0.2,-1.,-0.565685424949238));
#25699=CARTESIAN_POINT('',(0.2,-1.,0.));
#25700=CARTESIAN_POINT('',(0.2,0.,-0.565685424949238));
#25701=CARTESIAN_POINT('Origin',(0.2,0.,-0.78));
#25702=CARTESIAN_POINT('',(-0.2,2.2,-0.78));
#25703=CARTESIAN_POINT('',(0.1,2.2,-0.78));
#25704=CARTESIAN_POINT('',(-0.2,-1.,-0.78));
#25705=CARTESIAN_POINT('',(-0.2,0.,-0.78));
#25706=CARTESIAN_POINT('',(0.1,-1.,-0.78));
#25707=CARTESIAN_POINT('Origin',(-0.2,0.,-0.78));
#25708=CARTESIAN_POINT('',(-0.2,2.2,-0.565685424949238));
#25709=CARTESIAN_POINT('',(-0.2,2.2,-0.39));
#25710=CARTESIAN_POINT('',(-0.2,-1.,-0.565685424949238));
#25711=CARTESIAN_POINT('',(-0.2,0.,-0.565685424949238));
#25712=CARTESIAN_POINT('',(-0.2,-1.,-0.39));
#25713=CARTESIAN_POINT('Origin',(0.,-1.,0.));
#25714=CARTESIAN_POINT('',(1.60662857109684,-1.,0.693717979106306));
#25715=CARTESIAN_POINT('',(1.5055822144029,-1.,0.892032620296856));
#25716=CARTESIAN_POINT('Origin',(0.,-1.,0.));
#25717=CARTESIAN_POINT('',(1.81978687191668,-1.,1.23627494547115));
#25718=CARTESIAN_POINT('Ctrl Pts',(1.5055822144029,-1.,0.892032620296856));
#25719=CARTESIAN_POINT('Ctrl Pts',(1.50980486806688,-1.,0.894452006964544));
#25720=CARTESIAN_POINT('Ctrl Pts',(1.51805569590094,-1.,0.899185047483511));
#25721=CARTESIAN_POINT('Ctrl Pts',(1.52984849887993,-1.,0.905967409625651));
#25722=CARTESIAN_POINT('Ctrl Pts',(1.54440491149498,-1.,0.914375919026456));
#25723=CARTESIAN_POINT('Ctrl Pts',(1.56065988578893,-1.,0.923832188944341));
#25724=CARTESIAN_POINT('Ctrl Pts',(1.57499388382243,-1.,0.932246680108685));
#25725=CARTESIAN_POINT('Ctrl Pts',(1.58744937487176,-1.,0.939646377893399));
#25726=CARTESIAN_POINT('Ctrl Pts',(1.59810042043673,-1.,0.946078063315257));
#25727=CARTESIAN_POINT('Ctrl Pts',(1.60706069896936,-1.,0.951613284356035));
#25728=CARTESIAN_POINT('Ctrl Pts',(1.61449324337085,-1.,0.956354422920671));
#25729=CARTESIAN_POINT('Ctrl Pts',(1.62061638140221,-1.,0.960438326101729));
#25730=CARTESIAN_POINT('Ctrl Pts',(1.62571930670187,-1.,0.964046107040536));
#25731=CARTESIAN_POINT('Ctrl Pts',(1.63013849959461,-1.,0.967387853230345));
#25732=CARTESIAN_POINT('Ctrl Pts',(1.63420665729798,-1.,0.970669715997509));
#25733=CARTESIAN_POINT('Ctrl Pts',(1.63820952658144,-1.,0.974066058287419));
#25734=CARTESIAN_POINT('Ctrl Pts',(1.64233990826687,-1.,0.977689794119417));
#25735=CARTESIAN_POINT('Ctrl Pts',(1.64665139190656,-1.,0.981562530939489));
#25736=CARTESIAN_POINT('Ctrl Pts',(1.65110016612638,-1.,0.985642622920821));
#25737=CARTESIAN_POINT('Ctrl Pts',(1.65559044289699,-1.,0.989855627854165));
#25738=CARTESIAN_POINT('Ctrl Pts',(1.66001553809947,-1.,0.994121836661306));
#25739=CARTESIAN_POINT('Ctrl Pts',(1.66430758030376,-1.,0.998389654952758));
#25740=CARTESIAN_POINT('Ctrl Pts',(1.66846059277303,-1.,1.00265091003727));
#25741=CARTESIAN_POINT('Ctrl Pts',(1.67250335383293,-1.,1.00692206696414));
#25742=CARTESIAN_POINT('Ctrl Pts',(1.67648246776464,-1.,1.01123236493511));
#25743=CARTESIAN_POINT('Ctrl Pts',(1.68044289894798,-1.,1.01561026162773));
#25744=CARTESIAN_POINT('Ctrl Pts',(1.68440578021706,-1.,1.02006795074201));
#25745=CARTESIAN_POINT('Ctrl Pts',(1.68836910178447,-1.,1.02460180535255));
#25746=CARTESIAN_POINT('Ctrl Pts',(1.69231840863458,-1.,1.02919977579147));
#25747=CARTESIAN_POINT('Ctrl Pts',(1.69623414782771,-1.,1.03384646003588));
#25748=CARTESIAN_POINT('Ctrl Pts',(1.70010052930962,-1.,1.03852922490789));
#25749=CARTESIAN_POINT('Ctrl Pts',(1.70391338707982,-1.,1.04324363334554));
#25750=CARTESIAN_POINT('Ctrl Pts',(1.70767646263649,-1.,1.04799085404995));
#25751=CARTESIAN_POINT('Ctrl Pts',(1.71139783543989,-1.,1.05277517202855));
#25752=CARTESIAN_POINT('Ctrl Pts',(1.7150865442702,-1.,1.05760163192479));
#25753=CARTESIAN_POINT('Ctrl Pts',(1.71874858456904,-1.,1.06247324680647));
#25754=CARTESIAN_POINT('Ctrl Pts',(1.72238500928453,-1.,1.06738966975462));
#25755=CARTESIAN_POINT('Ctrl Pts',(1.72599406198488,-1.,1.07234866990252));
#25756=CARTESIAN_POINT('Ctrl Pts',(1.72957248977424,-1.,1.0773470373727));
#25757=CARTESIAN_POINT('Ctrl Pts',(1.73311705663407,-1.,1.08238162784749));
#25758=CARTESIAN_POINT('Ctrl Pts',(1.73662628326091,-1.,1.08745056285427));
#25759=CARTESIAN_POINT('Ctrl Pts',(1.74010053962247,-1.,1.09255329056493));
#25760=CARTESIAN_POINT('Ctrl Pts',(1.74354119236208,-1.,1.09768999241226));
#25761=CARTESIAN_POINT('Ctrl Pts',(1.74695004214923,-1.,1.10286118991143));
#25762=CARTESIAN_POINT('Ctrl Pts',(1.7503286607592,-1.,1.10806728183007));
#25763=CARTESIAN_POINT('Ctrl Pts',(1.7536777209463,-1.,1.11330807582551));
#25764=CARTESIAN_POINT('Ctrl Pts',(1.75699720772105,-1.,1.11858293216763));
#25765=CARTESIAN_POINT('Ctrl Pts',(1.76028671825096,-1.,1.12389096855086));
#25766=CARTESIAN_POINT('Ctrl Pts',(1.7635457196617,-1.,1.12923123555075));
#25767=CARTESIAN_POINT('Ctrl Pts',(1.76677384551862,-1.,1.1346029180462));
#25768=CARTESIAN_POINT('Ctrl Pts',(1.76997111386769,-1.,1.14000548336975));
#25769=CARTESIAN_POINT('Ctrl Pts',(1.77313777896194,-1.,1.1454385822692));
#25770=CARTESIAN_POINT('Ctrl Pts',(1.7762742255701,-1.,1.15090197841515));
#25771=CARTESIAN_POINT('Ctrl Pts',(1.77938085564275,-1.,1.15639547194698));
#25772=CARTESIAN_POINT('Ctrl Pts',(1.78245795881009,-1.,1.16191881298499));
#25773=CARTESIAN_POINT('Ctrl Pts',(1.78550566040443,-1.,1.16747166312303));
#25774=CARTESIAN_POINT('Ctrl Pts',(1.78852398877616,-1.,1.17305363177328));
#25775=CARTESIAN_POINT('Ctrl Pts',(1.79151291552689,-1.,1.17866429440809));
#25776=CARTESIAN_POINT('Ctrl Pts',(1.79447240321515,-1.,1.18430321697432));
#25777=CARTESIAN_POINT('Ctrl Pts',(1.79740245923478,-1.,1.18996997934445));
#25778=CARTESIAN_POINT('Ctrl Pts',(1.80030314369879,-1.,1.19566418930242));
#25779=CARTESIAN_POINT('Ctrl Pts',(1.80317454838603,-1.,1.20138548938974));
#25780=CARTESIAN_POINT('Ctrl Pts',(1.80601678480707,-1.,1.20713356605475));
#25781=CARTESIAN_POINT('Ctrl Pts',(1.80882996917129,-1.,1.21290815708314));
#25782=CARTESIAN_POINT('Ctrl Pts',(1.81161420806656,-1.,1.21870906103557));
#25783=CARTESIAN_POINT('Ctrl Pts',(1.81436959210434,-1.,1.2245361330495));
#25784=CARTESIAN_POINT('Ctrl Pts',(1.8165508718364,-1.,1.2292186489137));
#25785=CARTESIAN_POINT('Ctrl Pts',(1.81817389921279,-1.,1.2327422452705));
#25786=CARTESIAN_POINT('Ctrl Pts',(1.81925017193666,-1.,1.23509651170476));
#25787=CARTESIAN_POINT('Ctrl Pts',(1.81978687191668,-1.,1.23627494547115));
#25788=CARTESIAN_POINT('',(1.73811241238545,-1.,1.34869019493419));
#25789=CARTESIAN_POINT('',(1.81978687191668,-1.,1.23627494547115));
#25790=CARTESIAN_POINT('',(1.31362392696032,-1.,1.15624053661742));
#25791=CARTESIAN_POINT('Ctrl Pts',(1.73811241238545,-1.,1.34869019493419));
#25792=CARTESIAN_POINT('Ctrl Pts',(1.73682580585691,-1.,1.34854391898045));
#25793=CARTESIAN_POINT('Ctrl Pts',(1.73425417885907,-1.,1.34824783112887));
#25794=CARTESIAN_POINT('Ctrl Pts',(1.7304014965394,-1.,1.34779309152035));
#25795=CARTESIAN_POINT('Ctrl Pts',(1.72527410680674,-1.,1.34716554819527));
#25796=CARTESIAN_POINT('Ctrl Pts',(1.7188807715049,-1.,1.34634568653227));
#25797=CARTESIAN_POINT('Ctrl Pts',(1.71250340686822,-1.,1.34549029589416));
#25798=CARTESIAN_POINT('Ctrl Pts',(1.70614212266738,-1.,1.34459924533831));
#25799=CARTESIAN_POINT('Ctrl Pts',(1.69979707754427,-1.,1.34367237124483));
#25800=CARTESIAN_POINT('Ctrl Pts',(1.6934684849687,-1.,1.34270948206319));
#25801=CARTESIAN_POINT('Ctrl Pts',(1.68715660868764,-1.,1.341710374848));
#25802=CARTESIAN_POINT('Ctrl Pts',(1.68086176030362,-1.,1.34067485185203));
#25803=CARTESIAN_POINT('Ctrl Pts',(1.67458429426086,-1.,1.3396027347034));
#25804=CARTESIAN_POINT('Ctrl Pts',(1.66832460783989,-1.,1.33849388654388));
#25805=CARTESIAN_POINT('Ctrl Pts',(1.66208312541983,-1.,1.33734820885262));
#25806=CARTESIAN_POINT('Ctrl Pts',(1.65586025952593,-1.,1.33616559745172));
#25807=CARTESIAN_POINT('Ctrl Pts',(1.6496563728683,-1.,1.33494590467993));
#25808=CARTESIAN_POINT('Ctrl Pts',(1.6434717485603,-1.,1.33368890676572));
#25809=CARTESIAN_POINT('Ctrl Pts',(1.63730653475089,-1.,1.33239425103724));
#25810=CARTESIAN_POINT('Ctrl Pts',(1.63116079730923,-1.,1.33106149345645));
#25811=CARTESIAN_POINT('Ctrl Pts',(1.62503464209797,-1.,1.3296901950568));
#25812=CARTESIAN_POINT('Ctrl Pts',(1.61892832270724,-1.,1.32828000610449));
#25813=CARTESIAN_POINT('Ctrl Pts',(1.6128423401575,-1.,1.32683074483356));
#25814=CARTESIAN_POINT('Ctrl Pts',(1.60677758290954,-1.,1.32534250785782));
#25815=CARTESIAN_POINT('Ctrl Pts',(1.60073511858687,-1.,1.32381550858256));
#25816=CARTESIAN_POINT('Ctrl Pts',(1.59471591079403,-1.,1.32224985747682));
#25817=CARTESIAN_POINT('Ctrl Pts',(1.58872057258245,-1.,1.32064537110892));
#25818=CARTESIAN_POINT('Ctrl Pts',(1.58274907898834,-1.,1.31900135021432));
#25819=CARTESIAN_POINT('Ctrl Pts',(1.5768005650559,-1.,1.31731642317187));
#25820=CARTESIAN_POINT('Ctrl Pts',(1.57087397835723,-1.,1.31558903860016));
#25821=CARTESIAN_POINT('Ctrl Pts',(1.56496872402353,-1.,1.31381795281002));
#25822=CARTESIAN_POINT('Ctrl Pts',(1.55908521254821,-1.,1.31200264341696));
#25823=CARTESIAN_POINT('Ctrl Pts',(1.55322568759481,-1.,1.31014393684222));
#25824=CARTESIAN_POINT('Ctrl Pts',(1.54739413957185,-1.,1.30824393907473));
#25825=CARTESIAN_POINT('Ctrl Pts',(1.54159462645432,-1.,1.30630475189556));
#25826=CARTESIAN_POINT('Ctrl Pts',(1.53582981268977,-1.,1.30432735639489));
#25827=CARTESIAN_POINT('Ctrl Pts',(1.53009970283891,-1.,1.30231064395568));
#25828=CARTESIAN_POINT('Ctrl Pts',(1.52439957861062,-1.,1.30024984366328));
#25829=CARTESIAN_POINT('Ctrl Pts',(1.51872184912724,-1.,1.29813791800747));
#25830=CARTESIAN_POINT('Ctrl Pts',(1.51305994241402,-1.,1.29596850710509));
#25831=CARTESIAN_POINT('Ctrl Pts',(1.50741159078365,-1.,1.29373841372842));
#25832=CARTESIAN_POINT('Ctrl Pts',(1.50178230149776,-1.,1.29145022885181));
#25833=CARTESIAN_POINT('Ctrl Pts',(1.49618896881754,-1.,1.28911506584254));
#25834=CARTESIAN_POINT('Ctrl Pts',(1.4906522831278,-1.,1.2867467611644));
#25835=CARTESIAN_POINT('Ctrl Pts',(1.4851881711891,-1.,1.28435533880201));
#25836=CARTESIAN_POINT('Ctrl Pts',(1.47980070347095,-1.,1.28194158939517));
#25837=CARTESIAN_POINT('Ctrl Pts',(1.4744717526707,-1.,1.2794891824849));
#25838=CARTESIAN_POINT('Ctrl Pts',(1.46916035917133,-1.,1.2769641483109));
#25839=CARTESIAN_POINT('Ctrl Pts',(1.46382431332476,-1.,1.27433119897822));
#25840=CARTESIAN_POINT('Ctrl Pts',(1.45843906294697,-1.,1.27156805265289));
#25841=CARTESIAN_POINT('Ctrl Pts',(1.45301422764247,-1.,1.2686778680489));
#25842=CARTESIAN_POINT('Ctrl Pts',(1.44761985001662,-1.,1.26570925118868));
#25843=CARTESIAN_POINT('Ctrl Pts',(1.44236470511303,-1.,1.26273903323859));
#25844=CARTESIAN_POINT('Ctrl Pts',(1.43734919180847,-1.,1.25983531012005));
#25845=CARTESIAN_POINT('Ctrl Pts',(1.43262645609691,-1.,1.25702687965755));
#25846=CARTESIAN_POINT('Ctrl Pts',(1.42815938799387,-1.,1.25426945222639));
#25847=CARTESIAN_POINT('Ctrl Pts',(1.42378102115575,-1.,1.2514145557001));
#25848=CARTESIAN_POINT('Ctrl Pts',(1.41923722596025,-1.,1.24824430986571));
#25849=CARTESIAN_POINT('Ctrl Pts',(1.41422913175179,-1.,1.24450600513056));
#25850=CARTESIAN_POINT('Ctrl Pts',(1.40845295531283,-1.,1.23994455029534));
#25851=CARTESIAN_POINT('Ctrl Pts',(1.40164708206106,-1.,1.23434087290423));
#25852=CARTESIAN_POINT('Ctrl Pts',(1.39361389568796,-1.,1.22752961899387));
#25853=CARTESIAN_POINT('Ctrl Pts',(1.38420564527715,-1.,1.21938737280852));
#25854=CARTESIAN_POINT('Ctrl Pts',(1.37331915607905,-1.,1.20982812925645));
#25855=CARTESIAN_POINT('Ctrl Pts',(1.36088705043885,-1.,1.1987959077932));
#25856=CARTESIAN_POINT('Ctrl Pts',(1.34687054001093,-1.,1.18625865667441));
#25857=CARTESIAN_POINT('Ctrl Pts',(1.33437539347008,-1.,1.17501305789857));
#25858=CARTESIAN_POINT('Ctrl Pts',(1.32428080721772,-1.,1.16589330093588));
#25859=CARTESIAN_POINT('Ctrl Pts',(1.31722977216397,-1.,1.15950888730809));
#25860=CARTESIAN_POINT('Ctrl Pts',(1.31362392696032,-1.,1.15624053661742));
#25861=CARTESIAN_POINT('',(1.15624053661742,-1.,1.31362392696033));
#25862=CARTESIAN_POINT('Origin',(0.,-1.,0.));
#25863=CARTESIAN_POINT('',(1.34869019493419,-1.,1.73811241238545));
#25864=CARTESIAN_POINT('Ctrl Pts',(1.15624053661742,-1.,1.31362392696033));
#25865=CARTESIAN_POINT('Ctrl Pts',(1.15950888730433,-1.,1.3172297721596));
#25866=CARTESIAN_POINT('Ctrl Pts',(1.16589330092532,-1.,1.32428080720544));
#25867=CARTESIAN_POINT('Ctrl Pts',(1.17501305787994,-1.,1.33437539344842));
#25868=CARTESIAN_POINT('Ctrl Pts',(1.18625865664915,-1.,1.34687053998157));
#25869=CARTESIAN_POINT('Ctrl Pts',(1.1987959077656,-1.,1.36088705040677));
#25870=CARTESIAN_POINT('Ctrl Pts',(1.20982812923113,-1.,1.37331915604962));
#25871=CARTESIAN_POINT('Ctrl Pts',(1.21938737278853,-1.,1.38420564525391));
#25872=CARTESIAN_POINT('Ctrl Pts',(1.22752961898063,-1.,1.39361389567257));
#25873=CARTESIAN_POINT('Ctrl Pts',(1.23434087289768,-1.,1.40164708205345));
#25874=CARTESIAN_POINT('Ctrl Pts',(1.23994455029421,-1.,1.40845295531151));
#25875=CARTESIAN_POINT('Ctrl Pts',(1.24450600513278,-1.,1.41422913175437));
#25876=CARTESIAN_POINT('Ctrl Pts',(1.24824430986911,-1.,1.41923722596421));
#25877=CARTESIAN_POINT('Ctrl Pts',(1.25141455570299,-1.,1.42378102115911));
#25878=CARTESIAN_POINT('Ctrl Pts',(1.25426945222783,-1.,1.42815938799555));
#25879=CARTESIAN_POINT('Ctrl Pts',(1.25702687965744,-1.,1.43262645609679));
#25880=CARTESIAN_POINT('Ctrl Pts',(1.25983531011894,-1.,1.43734919180719));
#25881=CARTESIAN_POINT('Ctrl Pts',(1.26273903323723,-1.,1.44236470511145));
#25882=CARTESIAN_POINT('Ctrl Pts',(1.26570925118767,-1.,1.44761985001544));
#25883=CARTESIAN_POINT('Ctrl Pts',(1.26867786804854,-1.,1.45301422764205));
#25884=CARTESIAN_POINT('Ctrl Pts',(1.27156805265312,-1.,1.45843906294725));
#25885=CARTESIAN_POINT('Ctrl Pts',(1.27433119897877,-1.,1.4638243133254));
#25886=CARTESIAN_POINT('Ctrl Pts',(1.27696414831144,-1.,1.46916035917197));
#25887=CARTESIAN_POINT('Ctrl Pts',(1.27948918248524,-1.,1.4744717526711));
#25888=CARTESIAN_POINT('Ctrl Pts',(1.28194158939522,-1.,1.47980070347102));
#25889=CARTESIAN_POINT('Ctrl Pts',(1.28435533880184,-1.,1.48518817118891));
#25890=CARTESIAN_POINT('Ctrl Pts',(1.28674676116415,-1.,1.4906522831275));
#25891=CARTESIAN_POINT('Ctrl Pts',(1.28911506584232,-1.,1.49618896881729));
#25892=CARTESIAN_POINT('Ctrl Pts',(1.29145022885171,-1.,1.50178230149764));
#25893=CARTESIAN_POINT('Ctrl Pts',(1.29373841372843,-1.,1.50741159078367));
#25894=CARTESIAN_POINT('Ctrl Pts',(1.29596850710518,-1.,1.51305994241412));
#25895=CARTESIAN_POINT('Ctrl Pts',(1.29813791800757,-1.,1.51872184912735));
#25896=CARTESIAN_POINT('Ctrl Pts',(1.30024984366334,-1.,1.5243995786107));
#25897=CARTESIAN_POINT('Ctrl Pts',(1.3023106439557,-1.,1.53009970283893));
#25898=CARTESIAN_POINT('Ctrl Pts',(1.30432735639487,-1.,1.53582981268976));
#25899=CARTESIAN_POINT('Ctrl Pts',(1.30630475189553,-1.,1.54159462645428));
#25900=CARTESIAN_POINT('Ctrl Pts',(1.30824393907471,-1.,1.54739413957183));
#25901=CARTESIAN_POINT('Ctrl Pts',(1.31014393684221,-1.,1.55322568759481));
#25902=CARTESIAN_POINT('Ctrl Pts',(1.31200264341696,-1.,1.55908521254822));
#25903=CARTESIAN_POINT('Ctrl Pts',(1.31381795281002,-1.,1.56496872402352));
#25904=CARTESIAN_POINT('Ctrl Pts',(1.31558903860015,-1.,1.57087397835721));
#25905=CARTESIAN_POINT('Ctrl Pts',(1.31731642317183,-1.,1.57680056505585));
#25906=CARTESIAN_POINT('Ctrl Pts',(1.31900135021428,-1.,1.58274907898829));
#25907=CARTESIAN_POINT('Ctrl Pts',(1.32064537110891,-1.,1.58872057258244));
#25908=CARTESIAN_POINT('Ctrl Pts',(1.32224985747686,-1.,1.59471591079408));
#25909=CARTESIAN_POINT('Ctrl Pts',(1.32381550858266,-1.,1.600735118587));
#25910=CARTESIAN_POINT('Ctrl Pts',(1.32534250785794,-1.,1.6067775829097));
#25911=CARTESIAN_POINT('Ctrl Pts',(1.32683074483365,-1.,1.61284234015762));
#25912=CARTESIAN_POINT('Ctrl Pts',(1.32828000610448,-1.,1.61892832270723));
#25913=CARTESIAN_POINT('Ctrl Pts',(1.32969019505665,-1.,1.62503464209777));
#25914=CARTESIAN_POINT('Ctrl Pts',(1.33106149345618,-1.,1.63116079730887));
#25915=CARTESIAN_POINT('Ctrl Pts',(1.33239425103694,-1.,1.6373065347505));
#25916=CARTESIAN_POINT('Ctrl Pts',(1.33368890676554,-1.,1.64347174856007));
#25917=CARTESIAN_POINT('Ctrl Pts',(1.33494590468003,-1.,1.64965637286843));
#25918=CARTESIAN_POINT('Ctrl Pts',(1.33616559745217,-1.,1.65586025952651));
#25919=CARTESIAN_POINT('Ctrl Pts',(1.33734820885331,-1.,1.66208312542073));
#25920=CARTESIAN_POINT('Ctrl Pts',(1.33849388654458,-1.,1.66832460784078));
#25921=CARTESIAN_POINT('Ctrl Pts',(1.33960273470372,-1.,1.67458429426126));
#25922=CARTESIAN_POINT('Ctrl Pts',(1.3406748518516,-1.,1.68086176030308));
#25923=CARTESIAN_POINT('Ctrl Pts',(1.34171037484673,-1.,1.68715660868602));
#25924=CARTESIAN_POINT('Ctrl Pts',(1.34270948206139,-1.,1.6934684849664));
#25925=CARTESIAN_POINT('Ctrl Pts',(1.34367237124322,-1.,1.69979707754221));
#25926=CARTESIAN_POINT('Ctrl Pts',(1.34459924533783,-1.,1.70614212266676));
#25927=CARTESIAN_POINT('Ctrl Pts',(1.34549029589563,-1.,1.71250340687011));
#25928=CARTESIAN_POINT('Ctrl Pts',(1.34634568653586,-1.,1.7188807715095));
#25929=CARTESIAN_POINT('Ctrl Pts',(1.34716554820013,-1.,1.72527410681298));
#25930=CARTESIAN_POINT('Ctrl Pts',(1.3477930915247,-1.,1.73040149654497));
#25931=CARTESIAN_POINT('Ctrl Pts',(1.34824783113158,-1.,1.73425417886255));
#25932=CARTESIAN_POINT('Ctrl Pts',(1.34854391898145,-1.,1.73682580585819));
#25933=CARTESIAN_POINT('Ctrl Pts',(1.34869019493419,-1.,1.73811241238545));
#25934=CARTESIAN_POINT('',(1.23627494547115,-1.,1.81978687191668));
#25935=CARTESIAN_POINT('',(1.34869019493419,-1.,1.73811241238545));
#25936=CARTESIAN_POINT('',(0.892032620296855,-1.,1.5055822144029));
#25937=CARTESIAN_POINT('Ctrl Pts',(1.23627494547115,-1.,1.81978687191668));
#25938=CARTESIAN_POINT('Ctrl Pts',(1.23509651170384,-1.,1.81925017193531));
#25939=CARTESIAN_POINT('Ctrl Pts',(1.23274224526804,-1.,1.81817389920914));
#25940=CARTESIAN_POINT('Ctrl Pts',(1.22921864890975,-1.,1.81655087183054));
#25941=CARTESIAN_POINT('Ctrl Pts',(1.22453613304507,-1.,1.81436959209778));
#25942=CARTESIAN_POINT('Ctrl Pts',(1.2187090610323,-1.,1.81161420806172));
#25943=CARTESIAN_POINT('Ctrl Pts',(1.2129081570818,-1.,1.80882996916931));
#25944=CARTESIAN_POINT('Ctrl Pts',(1.20713356605519,-1.,1.80601678480772));
#25945=CARTESIAN_POINT('Ctrl Pts',(1.2013854893912,-1.,1.8031745483882));
#25946=CARTESIAN_POINT('Ctrl Pts',(1.19566418930405,-1.,1.80030314370121));
#25947=CARTESIAN_POINT('Ctrl Pts',(1.1899699793456,-1.,1.79740245923649));
#25948=CARTESIAN_POINT('Ctrl Pts',(1.18430321697471,-1.,1.79447240321572));
#25949=CARTESIAN_POINT('Ctrl Pts',(1.17866429440781,-1.,1.79151291552646));
#25950=CARTESIAN_POINT('Ctrl Pts',(1.17305363177265,-1.,1.78852398877523));
#25951=CARTESIAN_POINT('Ctrl Pts',(1.16747166312239,-1.,1.78550566040349));
#25952=CARTESIAN_POINT('Ctrl Pts',(1.16191881298458,-1.,1.78245795880949));
#25953=CARTESIAN_POINT('Ctrl Pts',(1.15639547194689,-1.,1.77938085564261));
#25954=CARTESIAN_POINT('Ctrl Pts',(1.15090197841531,-1.,1.77627422557034));
#25955=CARTESIAN_POINT('Ctrl Pts',(1.14543858226948,-1.,1.77313777896234));
#25956=CARTESIAN_POINT('Ctrl Pts',(1.14000548337,-1.,1.76997111386806));
#25957=CARTESIAN_POINT('Ctrl Pts',(1.13460291804634,-1.,1.76677384551883));
#25958=CARTESIAN_POINT('Ctrl Pts',(1.12923123555076,-1.,1.76354571966171));
#25959=CARTESIAN_POINT('Ctrl Pts',(1.12389096855078,-1.,1.76028671825084));
#25960=CARTESIAN_POINT('Ctrl Pts',(1.11858293216752,-1.,1.75699720772089));
#25961=CARTESIAN_POINT('Ctrl Pts',(1.11330807582542,-1.,1.75367772094617));
#25962=CARTESIAN_POINT('Ctrl Pts',(1.10806728183003,-1.,1.75032866075914));
#25963=CARTESIAN_POINT('Ctrl Pts',(1.10286118991144,-1.,1.74695004214924));
#25964=CARTESIAN_POINT('Ctrl Pts',(1.09768999241229,-1.,1.74354119236212));
#25965=CARTESIAN_POINT('Ctrl Pts',(1.09255329056496,-1.,1.74010053962252));
#25966=CARTESIAN_POINT('Ctrl Pts',(1.08745056285429,-1.,1.73662628326093));
#25967=CARTESIAN_POINT('Ctrl Pts',(1.08238162784749,-1.,1.73311705663407));
#25968=CARTESIAN_POINT('Ctrl Pts',(1.0773470373727,-1.,1.72957248977424));
#25969=CARTESIAN_POINT('Ctrl Pts',(1.07234866990252,-1.,1.72599406198489));
#25970=CARTESIAN_POINT('Ctrl Pts',(1.06738966975463,-1.,1.72238500928456));
#25971=CARTESIAN_POINT('Ctrl Pts',(1.06247324680649,-1.,1.71874858456908));
#25972=CARTESIAN_POINT('Ctrl Pts',(1.05760163192481,-1.,1.71508654427022));
#25973=CARTESIAN_POINT('Ctrl Pts',(1.05277517202853,-1.,1.71139783543986));
#25974=CARTESIAN_POINT('Ctrl Pts',(1.0479908540499,-1.,1.70767646263641));
#25975=CARTESIAN_POINT('Ctrl Pts',(1.04324363334546,-1.,1.70391338707969));
#25976=CARTESIAN_POINT('Ctrl Pts',(1.03852922490782,-1.,1.70010052930951));
#25977=CARTESIAN_POINT('Ctrl Pts',(1.03384646003587,-1.,1.69623414782769));
#25978=CARTESIAN_POINT('Ctrl Pts',(1.02919977579155,-1.,1.69231840863471));
#25979=CARTESIAN_POINT('Ctrl Pts',(1.02460180535272,-1.,1.68836910178475));
#25980=CARTESIAN_POINT('Ctrl Pts',(1.02006795074222,-1.,1.68440578021739));
#25981=CARTESIAN_POINT('Ctrl Pts',(1.01561026162786,-1.,1.6804428989482));
#25982=CARTESIAN_POINT('Ctrl Pts',(1.01123236493507,-1.,1.67648246776457));
#25983=CARTESIAN_POINT('Ctrl Pts',(1.00692206696387,-1.,1.67250335383248));
#25984=CARTESIAN_POINT('Ctrl Pts',(1.00265091003682,-1.,1.66846059277231));
#25985=CARTESIAN_POINT('Ctrl Pts',(0.998389654952317,-1.,1.66430758030304));
#25986=CARTESIAN_POINT('Ctrl Pts',(0.994121836661115,-1.,1.66001553809916));
#25987=CARTESIAN_POINT('Ctrl Pts',(0.98985562785445,-1.,1.65559044289746));
#25988=CARTESIAN_POINT('Ctrl Pts',(0.985642622921626,-1.,1.6511001661277));
#25989=CARTESIAN_POINT('Ctrl Pts',(0.981562530940574,-1.,1.64665139190834));
#25990=CARTESIAN_POINT('Ctrl Pts',(0.977689794120296,-1.,1.64233990826831));
#25991=CARTESIAN_POINT('Ctrl Pts',(0.974066058287501,-1.,1.63820952658157));
#25992=CARTESIAN_POINT('Ctrl Pts',(0.970669715996356,-1.,1.63420665729609));
#25993=CARTESIAN_POINT('Ctrl Pts',(0.967387853228041,-1.,1.63013849959083));
#25994=CARTESIAN_POINT('Ctrl Pts',(0.964046107037821,-1.,1.6257193066974));
#25995=CARTESIAN_POINT('Ctrl Pts',(0.960438326099958,-1.,1.62061638139929));
#25996=CARTESIAN_POINT('Ctrl Pts',(0.956354422921572,-1.,1.61449324337233));
#25997=CARTESIAN_POINT('Ctrl Pts',(0.951613284361247,-1.,1.60706069897794));
#25998=CARTESIAN_POINT('Ctrl Pts',(0.946078063325795,-1.,1.59810042045408));
#25999=CARTESIAN_POINT('Ctrl Pts',(0.939646377909319,-1.,1.58744937489796));
#26000=CARTESIAN_POINT('Ctrl Pts',(0.932246680128848,-1.,1.57499388385561));
#26001=CARTESIAN_POINT('Ctrl Pts',(0.923832188966322,-1.,1.56065988582509));
#26002=CARTESIAN_POINT('Ctrl Pts',(0.914375919046579,-1.,1.54440491152808));
#26003=CARTESIAN_POINT('Ctrl Pts',(0.905967409640498,-1.,1.52984849890434));
#26004=CARTESIAN_POINT('Ctrl Pts',(0.89918504749193,-1.,1.51805569591479));
#26005=CARTESIAN_POINT('Ctrl Pts',(0.894452006967538,-1.,1.50980486807181));
#26006=CARTESIAN_POINT('Ctrl Pts',(0.892032620296855,-1.,1.5055822144029));
#26007=CARTESIAN_POINT('',(0.693717979106305,-1.,1.60662857109684));
#26008=CARTESIAN_POINT('Origin',(0.,-1.,0.));
#26009=CARTESIAN_POINT('',(0.7455743247944,-1.,2.0698113262342));
#26010=CARTESIAN_POINT('Ctrl Pts',(0.693717979106305,-1.,1.60662857109684));
#26011=CARTESIAN_POINT('Ctrl Pts',(0.69571209787897,-1.,1.61106790957619));
#26012=CARTESIAN_POINT('Ctrl Pts',(0.699605146398836,-1.,1.61974673471117));
#26013=CARTESIAN_POINT('Ctrl Pts',(0.705159151977294,-1.,1.6321654166204));
#26014=CARTESIAN_POINT('Ctrl Pts',(0.711993139340447,-1.,1.64752408828442));
#26015=CARTESIAN_POINT('Ctrl Pts',(0.719585433787949,-1.,1.66472880551777));
#26016=CARTESIAN_POINT('Ctrl Pts',(0.726235967982445,-1.,1.67996158451922));
#26017=CARTESIAN_POINT('Ctrl Pts',(0.731963238685357,-1.,1.69326921972915));
#26018=CARTESIAN_POINT('Ctrl Pts',(0.736799665716932,-1.,1.70473309004249));
#26019=CARTESIAN_POINT('Ctrl Pts',(0.74079516202821,-1.,1.71447789751001));
#26020=CARTESIAN_POINT('Ctrl Pts',(0.744021445433093,-1.,1.72268229916769));
#26021=CARTESIAN_POINT('Ctrl Pts',(0.746574710097752,-1.,1.72958533647714));
#26022=CARTESIAN_POINT('Ctrl Pts',(0.74858246295687,-1.,1.7355035168033));
#26023=CARTESIAN_POINT('Ctrl Pts',(0.750193435981249,-1.,1.74080458267114));
#26024=CARTESIAN_POINT('Ctrl Pts',(0.751555614164482,-1.,1.74585086852502));
#26025=CARTESIAN_POINT('Ctrl Pts',(0.752797683531314,-1.,1.75095139468794));
#26026=CARTESIAN_POINT('Ctrl Pts',(0.754009254027828,-1.,1.75631083600019));
#26027=CARTESIAN_POINT('Ctrl Pts',(0.755220979974461,-1.,1.76197817240128));
#26028=CARTESIAN_POINT('Ctrl Pts',(0.75642189602781,-1.,1.76789396002998));
#26029=CARTESIAN_POINT('Ctrl Pts',(0.757578264077028,-1.,1.77394167108292));
#26030=CARTESIAN_POINT('Ctrl Pts',(0.758650626677518,-1.,1.77999411220945));
#26031=CARTESIAN_POINT('Ctrl Pts',(0.759614401110189,-1.,1.78596964884604));
#26032=CARTESIAN_POINT('Ctrl Pts',(0.760469555880749,-1.,1.7918581561088));
#26033=CARTESIAN_POINT('Ctrl Pts',(0.761229695230558,-1.,1.79768986997783));
#26034=CARTESIAN_POINT('Ctrl Pts',(0.761915336443547,-1.,1.80351583877342));
#26035=CARTESIAN_POINT('Ctrl Pts',(0.762546129463938,-1.,1.80938551463965));
#26036=CARTESIAN_POINT('Ctrl Pts',(0.763132003836634,-1.,1.8153211840553));
#26037=CARTESIAN_POINT('Ctrl Pts',(0.763673465462726,-1.,1.82131873145266));
#26038=CARTESIAN_POINT('Ctrl Pts',(0.764165902605995,-1.,1.82735991200065));
#26039=CARTESIAN_POINT('Ctrl Pts',(0.764602549687853,-1.,1.83342077227142));
#26040=CARTESIAN_POINT('Ctrl Pts',(0.764978057881737,-1.,1.83948181064835));
#26041=CARTESIAN_POINT('Ctrl Pts',(0.765291664862029,-1.,1.84553698875924));
#26042=CARTESIAN_POINT('Ctrl Pts',(0.765545710619062,-1.,1.85158945130063));
#26043=CARTESIAN_POINT('Ctrl Pts',(0.765744212909318,-1.,1.85764741390394));
#26044=CARTESIAN_POINT('Ctrl Pts',(0.765891519092547,-1.,1.86372027063312));
#26045=CARTESIAN_POINT('Ctrl Pts',(0.765990708546091,-1.,1.86981398314341));
#26046=CARTESIAN_POINT('Ctrl Pts',(0.766042837036744,-1.,1.87592888967883));
#26047=CARTESIAN_POINT('Ctrl Pts',(0.766047794851864,-1.,1.88206215302561));
#26048=CARTESIAN_POINT('Ctrl Pts',(0.766004837062091,-1.,1.88820926433409));
#26049=CARTESIAN_POINT('Ctrl Pts',(0.765913193856978,-1.,1.89436577771388));
#26050=CARTESIAN_POINT('Ctrl Pts',(0.765772772593386,-1.,1.90052930393596));
#26051=CARTESIAN_POINT('Ctrl Pts',(0.765584196937919,-1.,1.90669961402356));
#26052=CARTESIAN_POINT('Ctrl Pts',(0.765348465884722,-1.,1.91287765805169));
#26053=CARTESIAN_POINT('Ctrl Pts',(0.765066729667088,-1.,1.91906491634196));
#26054=CARTESIAN_POINT('Ctrl Pts',(0.764740025488211,-1.,1.92526263537048));
#26055=CARTESIAN_POINT('Ctrl Pts',(0.76436901067394,-1.,1.93147105496382));
#26056=CARTESIAN_POINT('Ctrl Pts',(0.763954049121458,-1.,1.93768964875886));
#26057=CARTESIAN_POINT('Ctrl Pts',(0.763495333538629,-1.,1.9439174661764));
#26058=CARTESIAN_POINT('Ctrl Pts',(0.762992990878769,-1.,1.95015342590024));
#26059=CARTESIAN_POINT('Ctrl Pts',(0.762447203806178,-1.,1.95639665309869));
#26060=CARTESIAN_POINT('Ctrl Pts',(0.761858300014423,-1.,1.96264672744186));
#26061=CARTESIAN_POINT('Ctrl Pts',(0.76122669048382,-1.,1.96890351582499));
#26062=CARTESIAN_POINT('Ctrl Pts',(0.760552825409757,-1.,1.97516705321494));
#26063=CARTESIAN_POINT('Ctrl Pts',(0.75983714745219,-1.,1.98143741418172));
#26064=CARTESIAN_POINT('Ctrl Pts',(0.759080037802488,-1.,1.98771456680874));
#26065=CARTESIAN_POINT('Ctrl Pts',(0.758281796766761,-1.,1.99399831098817));
#26066=CARTESIAN_POINT('Ctrl Pts',(0.757442676862724,-1.,2.00028834739178));
#26067=CARTESIAN_POINT('Ctrl Pts',(0.75656290464667,-1.,2.0065843158773));
#26068=CARTESIAN_POINT('Ctrl Pts',(0.755642704957865,-1.,2.01288584328084));
#26069=CARTESIAN_POINT('Ctrl Pts',(0.754682330722816,-1.,2.01919259405809));
#26070=CARTESIAN_POINT('Ctrl Pts',(0.753682061112768,-1.,2.02550428623313));
#26071=CARTESIAN_POINT('Ctrl Pts',(0.75264218048721,-1.,2.03182068456221));
#26072=CARTESIAN_POINT('Ctrl Pts',(0.751562963361115,-1.,2.03814160092099));
#26073=CARTESIAN_POINT('Ctrl Pts',(0.750444657875575,-1.,2.04446689147979));
#26074=CARTESIAN_POINT('Ctrl Pts',(0.749287468665046,-1.,2.05079645592154));
#26075=CARTESIAN_POINT('Ctrl Pts',(0.748091554183802,-1.,2.05713023031007));
#26076=CARTESIAN_POINT('Ctrl Pts',(0.747103932787919,-1.,2.06220058927826));
#26077=CARTESIAN_POINT('Ctrl Pts',(0.7463458715442,-1.,2.06600523016815));
#26078=CARTESIAN_POINT('Ctrl Pts',(0.745832791378367,-1.,2.06854248895728));
#26079=CARTESIAN_POINT('Ctrl Pts',(0.7455743247944,-1.,2.0698113262342));
#26080=CARTESIAN_POINT('',(0.61342227326009,-1.,2.11275013067528));
#26081=CARTESIAN_POINT('',(0.7455743247944,-1.,2.0698113262342));
#26082=CARTESIAN_POINT('',(0.383122945602004,-1.,1.7075470150345));
#26083=CARTESIAN_POINT('Ctrl Pts',(0.61342227326009,-1.,2.11275013067528));
#26084=CARTESIAN_POINT('Ctrl Pts',(0.6124673655618,-1.,2.11187554259986));
#26085=CARTESIAN_POINT('Ctrl Pts',(0.610560911689898,-1.,2.11012443807238));
#26086=CARTESIAN_POINT('Ctrl Pts',(0.607711315454876,-1.,2.1074919961518));
#26087=CARTESIAN_POINT('Ctrl Pts',(0.60393203073603,-1.,2.10397049886949));
#26088=CARTESIAN_POINT('Ctrl Pts',(0.599241616420533,-1.,2.0995493086477));
#26089=CARTESIAN_POINT('Ctrl Pts',(0.594585006052162,-1.,2.0951087622027));
#26090=CARTESIAN_POINT('Ctrl Pts',(0.589962365403406,-1.,2.09064881812129));
#26091=CARTESIAN_POINT('Ctrl Pts',(0.585373918991617,-1.,2.08616943727951));
#26092=CARTESIAN_POINT('Ctrl Pts',(0.580819952108063,-1.,2.08167059018418));
#26093=CARTESIAN_POINT('Ctrl Pts',(0.576300797416844,-1.,2.07715226767559));
#26094=CARTESIAN_POINT('Ctrl Pts',(0.571816823242602,-1.,2.07261449292824));
#26095=CARTESIAN_POINT('Ctrl Pts',(0.567368421181087,-1.,2.06805732997334));
#26096=CARTESIAN_POINT('Ctrl Pts',(0.562955993082261,-1.,2.06348090160589));
#26097=CARTESIAN_POINT('Ctrl Pts',(0.558579940185151,-1.,2.05888537756462));
#26098=CARTESIAN_POINT('Ctrl Pts',(0.554240657463906,-1.,2.05427091604413));
#26099=CARTESIAN_POINT('Ctrl Pts',(0.549938525150295,-1.,2.04963761077958));
#26100=CARTESIAN_POINT('Ctrl Pts',(0.54567390381743,-1.,2.04498544714588));
#26101=CARTESIAN_POINT('Ctrl Pts',(0.541447120615659,-1.,2.04031422690527));
#26102=CARTESIAN_POINT('Ctrl Pts',(0.537258489833262,-1.,2.03562362954037));
#26103=CARTESIAN_POINT('Ctrl Pts',(0.533108355132976,-1.,2.03091336214426));
#26104=CARTESIAN_POINT('Ctrl Pts',(0.528997127241914,-1.,2.0261832908329));
#26105=CARTESIAN_POINT('Ctrl Pts',(0.524925318333476,-1.,2.02143356304698));
#26106=CARTESIAN_POINT('Ctrl Pts',(0.52089359039937,-1.,2.01666477917286));
#26107=CARTESIAN_POINT('Ctrl Pts',(0.516902681728687,-1.,2.01187773939242));
#26108=CARTESIAN_POINT('Ctrl Pts',(0.512953306961792,-1.,2.00707309946949));
#26109=CARTESIAN_POINT('Ctrl Pts',(0.509046069886157,-1.,2.00225107134734));
#26110=CARTESIAN_POINT('Ctrl Pts',(0.505181361323026,-1.,1.99741107463572));
#26111=CARTESIAN_POINT('Ctrl Pts',(0.501359287727146,-1.,1.99255149126155));
#26112=CARTESIAN_POINT('Ctrl Pts',(0.497579909545574,-1.,1.98767044752932));
#26113=CARTESIAN_POINT('Ctrl Pts',(0.493843476541494,-1.,1.98276658761821));
#26114=CARTESIAN_POINT('Ctrl Pts',(0.490150627860952,-1.,1.97783973019229));
#26115=CARTESIAN_POINT('Ctrl Pts',(0.486502692907658,-1.,1.97289186263272));
#26116=CARTESIAN_POINT('Ctrl Pts',(0.48290166212069,-1.,1.96792703422362));
#26117=CARTESIAN_POINT('Ctrl Pts',(0.479349583074855,-1.,1.96294933055943));
#26118=CARTESIAN_POINT('Ctrl Pts',(0.475848034683176,-1.,1.95796111148177));
#26119=CARTESIAN_POINT('Ctrl Pts',(0.472397672264072,-1.,1.95296148278133));
#26120=CARTESIAN_POINT('Ctrl Pts',(0.468997482913135,-1.,1.94794381136514));
#26121=CARTESIAN_POINT('Ctrl Pts',(0.46564546202603,-1.,1.9428979419619));
#26122=CARTESIAN_POINT('Ctrl Pts',(0.462340031009056,-1.,1.93781486640821));
#26123=CARTESIAN_POINT('Ctrl Pts',(0.459081234547926,-1.,1.93269066517934));
#26124=CARTESIAN_POINT('Ctrl Pts',(0.45587200517437,-1.,1.92753067150476));
#26125=CARTESIAN_POINT('Ctrl Pts',(0.452719478359432,-1.,1.92235380648502));
#26126=CARTESIAN_POINT('Ctrl Pts',(0.449632260106662,-1.,1.91718342555755));
#26127=CARTESIAN_POINT('Ctrl Pts',(0.446617343485711,-1.,1.9120369998112));
#26128=CARTESIAN_POINT('Ctrl Pts',(0.44367755684915,-1.,1.90691756144898));
#26129=CARTESIAN_POINT('Ctrl Pts',(0.440807833704038,-1.,1.90180124389086));
#26130=CARTESIAN_POINT('Ctrl Pts',(0.437995003948244,-1.,1.89663648956466));
#26131=CARTESIAN_POINT('Ctrl Pts',(0.435225660963383,-1.,1.89136993975504));
#26132=CARTESIAN_POINT('Ctrl Pts',(0.432493038548748,-1.,1.88596913666793));
#26133=CARTESIAN_POINT('Ctrl Pts',(0.429803062482344,-1.,1.88044229001832));
#26134=CARTESIAN_POINT('Ctrl Pts',(0.427183828519102,-1.,1.87486989291484));
#26135=CARTESIAN_POINT('Ctrl Pts',(0.424678177291358,-1.,1.86937803944323));
#26136=CARTESIAN_POINT('Ctrl Pts',(0.422327307418275,-1.,1.86408083334028));
#26137=CARTESIAN_POINT('Ctrl Pts',(0.420157287975619,-1.,1.85903281096686));
#26138=CARTESIAN_POINT('Ctrl Pts',(0.418164129143534,-1.,1.85417632856234));
#26139=CARTESIAN_POINT('Ctrl Pts',(0.416300022038864,-1.,1.84929312929882));
#26140=CARTESIAN_POINT('Ctrl Pts',(0.41448743825434,-1.,1.8440575707371));
#26141=CARTESIAN_POINT('Ctrl Pts',(0.412633125322161,-1.,1.83808953475839));
#26142=CARTESIAN_POINT('Ctrl Pts',(0.410641256301674,-1.,1.83100408895216));
#26143=CARTESIAN_POINT('Ctrl Pts',(0.408428948108533,-1.,1.8224702267854));
#26144=CARTESIAN_POINT('Ctrl Pts',(0.405933518411838,-1.,1.81223801813988));
#26145=CARTESIAN_POINT('Ctrl Pts',(0.403107976170441,-1.,1.80012077176221));
#26146=CARTESIAN_POINT('Ctrl Pts',(0.39991940378308,-1.,1.78598826347533));
#26147=CARTESIAN_POINT('Ctrl Pts',(0.39634619612042,-1.,1.7697556004756));
#26148=CARTESIAN_POINT('Ctrl Pts',(0.392375812294307,-1.,1.75137405313962));
#26149=CARTESIAN_POINT('Ctrl Pts',(0.388877023509191,-1.,1.7349317097561));
#26150=CARTESIAN_POINT('Ctrl Pts',(0.38607079032701,-1.,1.72162022246158));
#26151=CARTESIAN_POINT('Ctrl Pts',(0.384119047315541,-1.,1.71231062891958));
#26152=CARTESIAN_POINT('Ctrl Pts',(0.383122945602004,-1.,1.7075470150345));
#26153=CARTESIAN_POINT('',(0.163289472382896,-1.,1.74236521665491));
#26154=CARTESIAN_POINT('Origin',(0.,-1.,0.));
#26155=CARTESIAN_POINT('',(0.0694764450219578,-1.,2.19890268624765));
#26156=CARTESIAN_POINT('Ctrl Pts',(0.163289472382896,-1.,1.74236521665491));
#26157=CARTESIAN_POINT('Ctrl Pts',(0.163814161002002,-1.,1.7472034950333));
#26158=CARTESIAN_POINT('Ctrl Pts',(0.164834765707158,-1.,1.75666056638427));
#26159=CARTESIAN_POINT('Ctrl Pts',(0.1662793551464,-1.,1.77018771684844));
#26160=CARTESIAN_POINT('Ctrl Pts',(0.168032772805197,-1.,1.7869064998507));
#26161=CARTESIAN_POINT('Ctrl Pts',(0.169936923904608,-1.,1.80561530629706));
#26162=CARTESIAN_POINT('Ctrl Pts',(0.171554770204119,-1.,1.82215766811545));
#26163=CARTESIAN_POINT('Ctrl Pts',(0.1728894428919,-1.,1.83658380527692));
#26164=CARTESIAN_POINT('Ctrl Pts',(0.173946627587731,-1.,1.8489811319852));
#26165=CARTESIAN_POINT('Ctrl Pts',(0.17473525927603,-1.,1.85948367088837));
#26166=CARTESIAN_POINT('Ctrl Pts',(0.175268337590757,-1.,1.86828349694799));
#26167=CARTESIAN_POINT('Ctrl Pts',(0.175563480746485,-1.,1.87563767773588));
#26168=CARTESIAN_POINT('Ctrl Pts',(0.175644148889698,-1.,1.88188663145367));
#26169=CARTESIAN_POINT('Ctrl Pts',(0.175538155840648,-1.,1.88742606273259));
#26170=CARTESIAN_POINT('Ctrl Pts',(0.175274276190844,-1.,1.892646301985));
#26171=CARTESIAN_POINT('Ctrl Pts',(0.174879405091263,-1.,1.89788101117132));
#26172=CARTESIAN_POINT('Ctrl Pts',(0.174375518661085,-1.,1.90335253862834));
#26173=CARTESIAN_POINT('Ctrl Pts',(0.173776635257816,-1.,1.90911693975267));
#26174=CARTESIAN_POINT('Ctrl Pts',(0.173090695383496,-1.,1.91511429159527));
#26175=CARTESIAN_POINT('Ctrl Pts',(0.172321621259513,-1.,1.9212233439798));
#26176=CARTESIAN_POINT('Ctrl Pts',(0.171471191532988,-1.,1.92731093582036));
#26177=CARTESIAN_POINT('Ctrl Pts',(0.170541253116201,-1.,1.93329183155539));
#26178=CARTESIAN_POINT('Ctrl Pts',(0.16953490481749,-1.,1.93915639211581));
#26179=CARTESIAN_POINT('Ctrl Pts',(0.168455741607556,-1.,1.94493757756931));
#26180=CARTESIAN_POINT('Ctrl Pts',(0.167307501784475,-1.,1.95069027794294));
#26181=CARTESIAN_POINT('Ctrl Pts',(0.166093592002812,-1.,1.9564675971873));
#26182=CARTESIAN_POINT('Ctrl Pts',(0.164816568920269,-1.,1.96229379940136));
#26183=CARTESIAN_POINT('Ctrl Pts',(0.163478185457734,-1.,1.96816512677967));
#26184=CARTESIAN_POINT('Ctrl Pts',(0.162079693556288,-1.,1.97406280235188));
#26185=CARTESIAN_POINT('Ctrl Pts',(0.160622060784611,-1.,1.97996195437559));
#26186=CARTESIAN_POINT('Ctrl Pts',(0.159106226437299,-1.,1.98584238283292));
#26187=CARTESIAN_POINT('Ctrl Pts',(0.157533331459227,-1.,1.99169810931908));
#26188=CARTESIAN_POINT('Ctrl Pts',(0.155904629548783,-1.,1.99753284771497));
#26189=CARTESIAN_POINT('Ctrl Pts',(0.154221403049722,-1.,2.00335565310543));
#26190=CARTESIAN_POINT('Ctrl Pts',(0.152484883621449,-1.,2.00917680318424));
#26191=CARTESIAN_POINT('Ctrl Pts',(0.150696157673078,-1.,2.01500291940238));
#26192=CARTESIAN_POINT('Ctrl Pts',(0.148856124775337,-1.,2.02083464969894));
#26193=CARTESIAN_POINT('Ctrl Pts',(0.146965557332583,-1.,2.02666926182017));
#26194=CARTESIAN_POINT('Ctrl Pts',(0.145025140186057,-1.,2.03250223739942));
#26195=CARTESIAN_POINT('Ctrl Pts',(0.143035515058208,-1.,2.03832911025912));
#26196=CARTESIAN_POINT('Ctrl Pts',(0.140997332152546,-1.,2.04414757947916));
#26197=CARTESIAN_POINT('Ctrl Pts',(0.138911255368966,-1.,2.04995762001328));
#26198=CARTESIAN_POINT('Ctrl Pts',(0.136777941218043,-1.,2.05576044414264));
#26199=CARTESIAN_POINT('Ctrl Pts',(0.134598026192106,-1.,2.06155781517842));
#26200=CARTESIAN_POINT('Ctrl Pts',(0.13237211154771,-1.,2.06735123910326));
#26201=CARTESIAN_POINT('Ctrl Pts',(0.130100748328403,-1.,2.07314114713063));
#26202=CARTESIAN_POINT('Ctrl Pts',(0.12778444527612,-1.,2.07892715110987));
#26203=CARTESIAN_POINT('Ctrl Pts',(0.125423679412061,-1.,2.08470840653643));
#26204=CARTESIAN_POINT('Ctrl Pts',(0.123018905621083,-1.,2.09048392424825));
#26205=CARTESIAN_POINT('Ctrl Pts',(0.120570567965122,-1.,2.0962529286773));
#26206=CARTESIAN_POINT('Ctrl Pts',(0.118079107988355,-1.,2.102015121329));
#26207=CARTESIAN_POINT('Ctrl Pts',(0.115544957687926,-1.,2.10777050261309));
#26208=CARTESIAN_POINT('Ctrl Pts',(0.112968534419737,-1.,2.11351924490306));
#26209=CARTESIAN_POINT('Ctrl Pts',(0.110350236135025,-1.,2.11926155590865));
#26210=CARTESIAN_POINT('Ctrl Pts',(0.10769043523109,-1.,2.12499752307));
#26211=CARTESIAN_POINT('Ctrl Pts',(0.104989479152739,-1.,2.13072704887293));
#26212=CARTESIAN_POINT('Ctrl Pts',(0.1022477005561,-1.,2.13644992667165));
#26213=CARTESIAN_POINT('Ctrl Pts',(0.0994654261990913,-1.,2.14216588396025));
#26214=CARTESIAN_POINT('Ctrl Pts',(0.0966429852305456,-1.,2.14787463531795));
#26215=CARTESIAN_POINT('Ctrl Pts',(0.0937807218867641,-1.,2.1535759397817));
#26216=CARTESIAN_POINT('Ctrl Pts',(0.0908789888107263,-1.,2.15926961544516));
#26217=CARTESIAN_POINT('Ctrl Pts',(0.087938129138692,-1.,2.16495552645014));
#26218=CARTESIAN_POINT('Ctrl Pts',(0.084958462083537,-1.,2.17063357870952));
#26219=CARTESIAN_POINT('Ctrl Pts',(0.0819402680872763,-1.,2.176303712113));
#26220=CARTESIAN_POINT('Ctrl Pts',(0.078883772768524,-1.,2.18196589448887));
#26221=CARTESIAN_POINT('Ctrl Pts',(0.0757891465836145,-1.,2.1876201139953));
#26222=CARTESIAN_POINT('Ctrl Pts',(0.0732830357306722,-1.,2.19213712013662));
#26223=CARTESIAN_POINT('Ctrl Pts',(0.0713863779526151,-1.,2.19552129484002));
#26224=CARTESIAN_POINT('Ctrl Pts',(0.0701143536325487,-1.,2.19777582085423));
#26225=CARTESIAN_POINT('Ctrl Pts',(0.0694764450219578,-1.,2.19890268624765));
#26226=CARTESIAN_POINT('',(-0.0694764450219586,-1.,2.19890268624765));
#26227=CARTESIAN_POINT('',(0.0694764450219578,-1.,2.19890268624765));
#26228=CARTESIAN_POINT('',(-0.163289472382896,-1.,1.74236521665491));
#26229=CARTESIAN_POINT('Ctrl Pts',(-0.0694764450219586,-1.,2.19890268624765));
#26230=CARTESIAN_POINT('Ctrl Pts',(-0.0701143536324929,-1.,2.19777582085261));
#26231=CARTESIAN_POINT('Ctrl Pts',(-0.071386377952463,-1.,2.19552129483562));
#26232=CARTESIAN_POINT('Ctrl Pts',(-0.0732830357304279,-1.,2.19213712012956));
#26233=CARTESIAN_POINT('Ctrl Pts',(-0.0757891465833414,-1.,2.1876201139874));
#26234=CARTESIAN_POINT('Ctrl Pts',(-0.078883772768323,-1.,2.18196589448304));
#26235=CARTESIAN_POINT('Ctrl Pts',(-0.0819402680871942,-1.,2.1763037121106));
#26236=CARTESIAN_POINT('Ctrl Pts',(-0.0849584620835646,-1.,2.17063357871031));
#26237=CARTESIAN_POINT('Ctrl Pts',(-0.0879381291387825,-1.,2.16495552645275));
#26238=CARTESIAN_POINT('Ctrl Pts',(-0.0908789888108269,-1.,2.15926961544808));
#26239=CARTESIAN_POINT('Ctrl Pts',(-0.0937807218868348,-1.,2.15357593978377));
#26240=CARTESIAN_POINT('Ctrl Pts',(-0.0966429852305691,-1.,2.14787463531864));
#26241=CARTESIAN_POINT('Ctrl Pts',(-0.0994654261990745,-1.,2.14216588395974));
#26242=CARTESIAN_POINT('Ctrl Pts',(-0.102247700556064,-1.,2.13644992667052));
#26243=CARTESIAN_POINT('Ctrl Pts',(-0.104989479152703,-1.,2.1307270488718));
#26244=CARTESIAN_POINT('Ctrl Pts',(-0.107690435231068,-1.,2.12499752306927));
#26245=CARTESIAN_POINT('Ctrl Pts',(-0.11035023613502,-1.,2.11926155590849));
#26246=CARTESIAN_POINT('Ctrl Pts',(-0.112968534419746,-1.,2.11351924490335));
#26247=CARTESIAN_POINT('Ctrl Pts',(-0.115544957687941,-1.,2.10777050261359));
#26248=CARTESIAN_POINT('Ctrl Pts',(-0.118079107988368,-1.,2.10201512132945));
#26249=CARTESIAN_POINT('Ctrl Pts',(-0.120570567965129,-1.,2.09625292867756));
#26250=CARTESIAN_POINT('Ctrl Pts',(-0.123018905621083,-1.,2.09048392424826));
#26251=CARTESIAN_POINT('Ctrl Pts',(-0.125423679412058,-1.,2.08470840653628));
#26252=CARTESIAN_POINT('Ctrl Pts',(-0.127784445276116,-1.,2.07892715110967));
#26253=CARTESIAN_POINT('Ctrl Pts',(-0.130100748328401,-1.,2.07314114713047));
#26254=CARTESIAN_POINT('Ctrl Pts',(-0.13237211154771,-1.,2.06735123910319));
#26255=CARTESIAN_POINT('Ctrl Pts',(-0.134598026192107,-1.,2.06155781517844));
#26256=CARTESIAN_POINT('Ctrl Pts',(-0.136777941218044,-1.,2.0557604441427));
#26257=CARTESIAN_POINT('Ctrl Pts',(-0.138911255368966,-1.,2.04995762001333));
#26258=CARTESIAN_POINT('Ctrl Pts',(-0.140997332152546,-1.,2.04414757947919));
#26259=CARTESIAN_POINT('Ctrl Pts',(-0.143035515058208,-1.,2.03832911025913));
#26260=CARTESIAN_POINT('Ctrl Pts',(-0.145025140186058,-1.,2.03250223739941));
#26261=CARTESIAN_POINT('Ctrl Pts',(-0.146965557332586,-1.,2.02666926182017));
#26262=CARTESIAN_POINT('Ctrl Pts',(-0.148856124775343,-1.,2.02083464969897));
#26263=CARTESIAN_POINT('Ctrl Pts',(-0.150696157673084,-1.,2.01500291940243));
#26264=CARTESIAN_POINT('Ctrl Pts',(-0.152484883621452,-1.,2.00917680318426));
#26265=CARTESIAN_POINT('Ctrl Pts',(-0.154221403049719,-1.,2.00335565310539));
#26266=CARTESIAN_POINT('Ctrl Pts',(-0.155904629548775,-1.,1.99753284771487));
#26267=CARTESIAN_POINT('Ctrl Pts',(-0.157533331459215,-1.,1.99169810931893));
#26268=CARTESIAN_POINT('Ctrl Pts',(-0.159106226437289,-1.,1.98584238283279));
#26269=CARTESIAN_POINT('Ctrl Pts',(-0.16062206078461,-1.,1.97996195437557));
#26270=CARTESIAN_POINT('Ctrl Pts',(-0.162079693556302,-1.,1.97406280235204));
#26271=CARTESIAN_POINT('Ctrl Pts',(-0.16347818545776,-1.,1.96816512678));
#26272=CARTESIAN_POINT('Ctrl Pts',(-0.1648165689203,-1.,1.96229379940174));
#26273=CARTESIAN_POINT('Ctrl Pts',(-0.166093592002833,-1.,1.95646759718755));
#26274=CARTESIAN_POINT('Ctrl Pts',(-0.167307501784469,-1.,1.95069027794286));
#26275=CARTESIAN_POINT('Ctrl Pts',(-0.168455741607516,-1.,1.94493757756879));
#26276=CARTESIAN_POINT('Ctrl Pts',(-0.169534904817425,-1.,1.93915639211497));
#26277=CARTESIAN_POINT('Ctrl Pts',(-0.170541253116136,-1.,1.93329183155455));
#26278=CARTESIAN_POINT('Ctrl Pts',(-0.17147119153296,-1.,1.92731093582));
#26279=CARTESIAN_POINT('Ctrl Pts',(-0.172321621259557,-1.,1.92122334398034));
#26280=CARTESIAN_POINT('Ctrl Pts',(-0.173090695383619,-1.,1.91511429159681));
#26281=CARTESIAN_POINT('Ctrl Pts',(-0.173776635257984,-1.,1.90911693975475));
#26282=CARTESIAN_POINT('Ctrl Pts',(-0.174375518661222,-1.,1.90335253863003));
#26283=CARTESIAN_POINT('Ctrl Pts',(-0.174879405091277,-1.,1.89788101117148));
#26284=CARTESIAN_POINT('Ctrl Pts',(-0.175274276190664,-1.,1.89264630198279));
#26285=CARTESIAN_POINT('Ctrl Pts',(-0.175538155840286,-1.,1.88742606272818));
#26286=CARTESIAN_POINT('Ctrl Pts',(-0.175644148889271,-1.,1.88188663144846));
#26287=CARTESIAN_POINT('Ctrl Pts',(-0.175563480746206,-1.,1.87563767773249));
#26288=CARTESIAN_POINT('Ctrl Pts',(-0.175268337590901,-1.,1.86828349694972));
#26289=CARTESIAN_POINT('Ctrl Pts',(-0.174735259276856,-1.,1.85948367089838));
#26290=CARTESIAN_POINT('Ctrl Pts',(-0.173946627589401,-1.,1.84898113200543));
#26291=CARTESIAN_POINT('Ctrl Pts',(-0.17288944289442,-1.,1.83658380530747));
#26292=CARTESIAN_POINT('Ctrl Pts',(-0.171554770207306,-1.,1.82215766815414));
#26293=CARTESIAN_POINT('Ctrl Pts',(-0.169936923908078,-1.,1.80561530633924));
#26294=CARTESIAN_POINT('Ctrl Pts',(-0.16803277280837,-1.,1.78690649988931));
#26295=CARTESIAN_POINT('Ctrl Pts',(-0.166279355148738,-1.,1.77018771687692));
#26296=CARTESIAN_POINT('Ctrl Pts',(-0.164834765708484,-1.,1.75666056640041));
#26297=CARTESIAN_POINT('Ctrl Pts',(-0.163814161002474,-1.,1.74720349503904));
#26298=CARTESIAN_POINT('Ctrl Pts',(-0.163289472382896,-1.,1.74236521665491));
#26299=CARTESIAN_POINT('',(-0.383122945602004,-1.,1.7075470150345));
#26300=CARTESIAN_POINT('Origin',(0.,-1.,0.));
#26301=CARTESIAN_POINT('',(-0.61342227326009,-1.,2.11275013067528));
#26302=CARTESIAN_POINT('Ctrl Pts',(-0.383122945602004,-1.,1.7075470150345));
#26303=CARTESIAN_POINT('Ctrl Pts',(-0.384119047314215,-1.,1.71231062891398));
#26304=CARTESIAN_POINT('Ctrl Pts',(-0.386070790323281,-1.,1.72162022244582));
#26305=CARTESIAN_POINT('Ctrl Pts',(-0.388877023502615,-1.,1.73493170972829));
#26306=CARTESIAN_POINT('Ctrl Pts',(-0.392375812285395,-1.,1.75137405310193));
#26307=CARTESIAN_POINT('Ctrl Pts',(-0.396346196110688,-1.,1.76975560043442));
#26308=CARTESIAN_POINT('Ctrl Pts',(-0.399919403774155,-1.,1.78598826343754));
#26309=CARTESIAN_POINT('Ctrl Pts',(-0.403107976163396,-1.,1.80012077173238));
#26310=CARTESIAN_POINT('Ctrl Pts',(-0.405933518407175,-1.,1.81223801812013));
#26311=CARTESIAN_POINT('Ctrl Pts',(-0.408428948106227,-1.,1.82247022677562));
#26312=CARTESIAN_POINT('Ctrl Pts',(-0.410641256301276,-1.,1.83100408895047));
#26313=CARTESIAN_POINT('Ctrl Pts',(-0.412633125322945,-1.,1.8380895347617));
#26314=CARTESIAN_POINT('Ctrl Pts',(-0.414487438255542,-1.,1.84405757074218));
#26315=CARTESIAN_POINT('Ctrl Pts',(-0.416300022039885,-1.,1.84929312930314));
#26316=CARTESIAN_POINT('Ctrl Pts',(-0.418164129144045,-1.,1.8541763285645));
#26317=CARTESIAN_POINT('Ctrl Pts',(-0.420157287975583,-1.,1.8590328109667));
#26318=CARTESIAN_POINT('Ctrl Pts',(-0.422327307417885,-1.,1.86408083333863));
#26319=CARTESIAN_POINT('Ctrl Pts',(-0.424678177290876,-1.,1.8693780394412));
#26320=CARTESIAN_POINT('Ctrl Pts',(-0.427183828518743,-1.,1.87486989291333));
#26321=CARTESIAN_POINT('Ctrl Pts',(-0.429803062482217,-1.,1.88044229001778));
#26322=CARTESIAN_POINT('Ctrl Pts',(-0.432493038548833,-1.,1.88596913666828));
#26323=CARTESIAN_POINT('Ctrl Pts',(-0.43522566096358,-1.,1.89136993975585));
#26324=CARTESIAN_POINT('Ctrl Pts',(-0.437995003948443,-1.,1.89663648956549));
#26325=CARTESIAN_POINT('Ctrl Pts',(-0.440807833704161,-1.,1.90180124389137));
#26326=CARTESIAN_POINT('Ctrl Pts',(-0.44367755684917,-1.,1.90691756144906));
#26327=CARTESIAN_POINT('Ctrl Pts',(-0.446617343485651,-1.,1.91203699981095));
#26328=CARTESIAN_POINT('Ctrl Pts',(-0.449632260106572,-1.,1.91718342555717));
#26329=CARTESIAN_POINT('Ctrl Pts',(-0.452719478359356,-1.,1.9223538064847));
#26330=CARTESIAN_POINT('Ctrl Pts',(-0.455872005174335,-1.,1.92753067150461));
#26331=CARTESIAN_POINT('Ctrl Pts',(-0.459081234547931,-1.,1.93269066517936));
#26332=CARTESIAN_POINT('Ctrl Pts',(-0.462340031009087,-1.,1.93781486640834));
#26333=CARTESIAN_POINT('Ctrl Pts',(-0.465645462026065,-1.,1.94289794196205));
#26334=CARTESIAN_POINT('Ctrl Pts',(-0.468997482913158,-1.,1.94794381136524));
#26335=CARTESIAN_POINT('Ctrl Pts',(-0.47239767226408,-1.,1.95296148278136));
#26336=CARTESIAN_POINT('Ctrl Pts',(-0.475848034683172,-1.,1.95796111148175));
#26337=CARTESIAN_POINT('Ctrl Pts',(-0.479349583074846,-1.,1.96294933055938));
#26338=CARTESIAN_POINT('Ctrl Pts',(-0.482901662120687,-1.,1.96792703422358));
#26339=CARTESIAN_POINT('Ctrl Pts',(-0.486502692907661,-1.,1.97289186263272));
#26340=CARTESIAN_POINT('Ctrl Pts',(-0.490150627860955,-1.,1.97783973019229));
#26341=CARTESIAN_POINT('Ctrl Pts',(-0.493843476541492,-1.,1.9827665876182));
#26342=CARTESIAN_POINT('Ctrl Pts',(-0.497579909545564,-1.,1.98767044752929));
#26343=CARTESIAN_POINT('Ctrl Pts',(-0.501359287727129,-1.,1.9925514912615));
#26344=CARTESIAN_POINT('Ctrl Pts',(-0.505181361323011,-1.,1.99741107463567));
#26345=CARTESIAN_POINT('Ctrl Pts',(-0.509046069886152,-1.,2.00225107134733));
#26346=CARTESIAN_POINT('Ctrl Pts',(-0.512953306961814,-1.,2.00707309946955));
#26347=CARTESIAN_POINT('Ctrl Pts',(-0.516902681728733,-1.,2.01187773939257));
#26348=CARTESIAN_POINT('Ctrl Pts',(-0.520893590399428,-1.,2.01666477917305));
#26349=CARTESIAN_POINT('Ctrl Pts',(-0.524925318333518,-1.,2.02143356304712));
#26350=CARTESIAN_POINT('Ctrl Pts',(-0.528997127241911,-1.,2.02618329083289));
#26351=CARTESIAN_POINT('Ctrl Pts',(-0.533108355132905,-1.,2.03091336214401));
#26352=CARTESIAN_POINT('Ctrl Pts',(-0.537258489833134,-1.,2.03562362953993));
#26353=CARTESIAN_POINT('Ctrl Pts',(-0.54144712061552,-1.,2.0403142269048));
#26354=CARTESIAN_POINT('Ctrl Pts',(-0.545673903817348,-1.,2.0449854471456));
#26355=CARTESIAN_POINT('Ctrl Pts',(-0.549938525150342,-1.,2.04963761077974));
#26356=CARTESIAN_POINT('Ctrl Pts',(-0.55424065746411,-1.,2.05427091604482));
#26357=CARTESIAN_POINT('Ctrl Pts',(-0.558579940185467,-1.,2.05888537756571));
#26358=CARTESIAN_POINT('Ctrl Pts',(-0.562955993082574,-1.,2.06348090160697));
#26359=CARTESIAN_POINT('Ctrl Pts',(-0.567368421181229,-1.,2.06805732997383));
#26360=CARTESIAN_POINT('Ctrl Pts',(-0.571816823242411,-1.,2.07261449292757));
#26361=CARTESIAN_POINT('Ctrl Pts',(-0.576300797416275,-1.,2.07715226767361));
#26362=CARTESIAN_POINT('Ctrl Pts',(-0.580819952107257,-1.,2.08167059018138));
#26363=CARTESIAN_POINT('Ctrl Pts',(-0.585373918990895,-1.,2.086169437277));
#26364=CARTESIAN_POINT('Ctrl Pts',(-0.589962365403189,-1.,2.09064881812053));
#26365=CARTESIAN_POINT('Ctrl Pts',(-0.594585006052824,-1.,2.09510876220501));
#26366=CARTESIAN_POINT('Ctrl Pts',(-0.599241616422144,-1.,2.09954930865331));
#26367=CARTESIAN_POINT('Ctrl Pts',(-0.603932030738212,-1.,2.10397049887709));
#26368=CARTESIAN_POINT('Ctrl Pts',(-0.607711315456826,-1.,2.10749199615859));
#26369=CARTESIAN_POINT('Ctrl Pts',(-0.610560911691113,-1.,2.11012443807661));
#26370=CARTESIAN_POINT('Ctrl Pts',(-0.61246736556225,-1.,2.11187554260142));
#26371=CARTESIAN_POINT('Ctrl Pts',(-0.61342227326009,-1.,2.11275013067528));
#26372=CARTESIAN_POINT('',(-0.745574324794401,-1.,2.0698113262342));
#26373=CARTESIAN_POINT('',(-0.61342227326009,-1.,2.11275013067528));
#26374=CARTESIAN_POINT('',(-0.693717979106306,-1.,1.60662857109684));
#26375=CARTESIAN_POINT('Ctrl Pts',(-0.745574324794401,-1.,2.0698113262342));
#26376=CARTESIAN_POINT('Ctrl Pts',(-0.74583279137781,-1.,2.06854248895575));
#26377=CARTESIAN_POINT('Ctrl Pts',(-0.746345871542696,-1.,2.06600523016401));
#26378=CARTESIAN_POINT('Ctrl Pts',(-0.747103932785504,-1.,2.06220058927162));
#26379=CARTESIAN_POINT('Ctrl Pts',(-0.748091554181101,-1.,2.05713023030263));
#26380=CARTESIAN_POINT('Ctrl Pts',(-0.749287468663053,-1.,2.05079645591606));
#26381=CARTESIAN_POINT('Ctrl Pts',(-0.750444657874758,-1.,2.04446689147754));
#26382=CARTESIAN_POINT('Ctrl Pts',(-0.751562963361384,-1.,2.03814160092173));
#26383=CARTESIAN_POINT('Ctrl Pts',(-0.752642180488104,-1.,2.03182068456467));
#26384=CARTESIAN_POINT('Ctrl Pts',(-0.753682061113766,-1.,2.02550428623587));
#26385=CARTESIAN_POINT('Ctrl Pts',(-0.75468233072352,-1.,2.01919259406003));
#26386=CARTESIAN_POINT('Ctrl Pts',(-0.7556427049581,-1.,2.01288584328149));
#26387=CARTESIAN_POINT('Ctrl Pts',(-0.756562904646496,-1.,2.00658431587682));
#26388=CARTESIAN_POINT('Ctrl Pts',(-0.757442676862341,-1.,2.00028834739072));
#26389=CARTESIAN_POINT('Ctrl Pts',(-0.758281796766377,-1.,1.9939983109871));
#26390=CARTESIAN_POINT('Ctrl Pts',(-0.759080037802243,-1.,1.98771456680806));
#26391=CARTESIAN_POINT('Ctrl Pts',(-0.759837147452135,-1.,1.98143741418156));
#26392=CARTESIAN_POINT('Ctrl Pts',(-0.760552825409855,-1.,1.97516705321521));
#26393=CARTESIAN_POINT('Ctrl Pts',(-0.761226690483986,-1.,1.96890351582545));
#26394=CARTESIAN_POINT('Ctrl Pts',(-0.761858300014575,-1.,1.96264672744229));
#26395=CARTESIAN_POINT('Ctrl Pts',(-0.762447203806263,-1.,1.95639665309893));
#26396=CARTESIAN_POINT('Ctrl Pts',(-0.762992990878774,-1.,1.95015342590025));
#26397=CARTESIAN_POINT('Ctrl Pts',(-0.76349533353858,-1.,1.94391746617626));
#26398=CARTESIAN_POINT('Ctrl Pts',(-0.763954049121393,-1.,1.93768964875867));
#26399=CARTESIAN_POINT('Ctrl Pts',(-0.764369010673889,-1.,1.93147105496367));
#26400=CARTESIAN_POINT('Ctrl Pts',(-0.764740025488189,-1.,1.92526263537041));
#26401=CARTESIAN_POINT('Ctrl Pts',(-0.765066729667095,-1.,1.91906491634197));
#26402=CARTESIAN_POINT('Ctrl Pts',(-0.765348465884739,-1.,1.91287765805174));
#26403=CARTESIAN_POINT('Ctrl Pts',(-0.765584196937936,-1.,1.90669961402362));
#26404=CARTESIAN_POINT('Ctrl Pts',(-0.765772772593395,-1.,1.90052930393599));
#26405=CARTESIAN_POINT('Ctrl Pts',(-0.765913193856979,-1.,1.89436577771389));
#26406=CARTESIAN_POINT('Ctrl Pts',(-0.76600483706209,-1.,1.88820926433409));
#26407=CARTESIAN_POINT('Ctrl Pts',(-0.766047794851869,-1.,1.88206215302561));
#26408=CARTESIAN_POINT('Ctrl Pts',(-0.766042837036759,-1.,1.87592888967886));
#26409=CARTESIAN_POINT('Ctrl Pts',(-0.765990708546111,-1.,1.86981398314345));
#26410=CARTESIAN_POINT('Ctrl Pts',(-0.765891519092557,-1.,1.86372027063314));
#26411=CARTESIAN_POINT('Ctrl Pts',(-0.765744212909305,-1.,1.85764741390391));
#26412=CARTESIAN_POINT('Ctrl Pts',(-0.765545710619023,-1.,1.85158945130054));
#26413=CARTESIAN_POINT('Ctrl Pts',(-0.765291664861971,-1.,1.8455369887591));
#26414=CARTESIAN_POINT('Ctrl Pts',(-0.764978057881687,-1.,1.83948181064823));
#26415=CARTESIAN_POINT('Ctrl Pts',(-0.764602549687845,-1.,1.8334207722714));
#26416=CARTESIAN_POINT('Ctrl Pts',(-0.764165902606055,-1.,1.8273599120008));
#26417=CARTESIAN_POINT('Ctrl Pts',(-0.763673465462854,-1.,1.82131873145297));
#26418=CARTESIAN_POINT('Ctrl Pts',(-0.763132003836783,-1.,1.81532118405566));
#26419=CARTESIAN_POINT('Ctrl Pts',(-0.762546129464036,-1.,1.80938551463989));
#26420=CARTESIAN_POINT('Ctrl Pts',(-0.761915336443516,-1.,1.80351583877334));
#26421=CARTESIAN_POINT('Ctrl Pts',(-0.761229695230359,-1.,1.79768986997735));
#26422=CARTESIAN_POINT('Ctrl Pts',(-0.760469555880425,-1.,1.79185815610802));
#26423=CARTESIAN_POINT('Ctrl Pts',(-0.759614401109868,-1.,1.78596964884526));
#26424=CARTESIAN_POINT('Ctrl Pts',(-0.75865062667738,-1.,1.77999411220912));
#26425=CARTESIAN_POINT('Ctrl Pts',(-0.757578264077238,-1.,1.77394167108342));
#26426=CARTESIAN_POINT('Ctrl Pts',(-0.756421896028403,-1.,1.76789396003141));
#26427=CARTESIAN_POINT('Ctrl Pts',(-0.755220979975262,-1.,1.7619781724032));
#26428=CARTESIAN_POINT('Ctrl Pts',(-0.75400925402848,-1.,1.75631083600175));
#26429=CARTESIAN_POINT('Ctrl Pts',(-0.752797683531377,-1.,1.75095139468809));
#26430=CARTESIAN_POINT('Ctrl Pts',(-0.751555614163629,-1.,1.74585086852298));
#26431=CARTESIAN_POINT('Ctrl Pts',(-0.75019343597954,-1.,1.74080458266705));
#26432=CARTESIAN_POINT('Ctrl Pts',(-0.748582462954855,-1.,1.73550351679848));
#26433=CARTESIAN_POINT('Ctrl Pts',(-0.746574710096436,-1.,1.72958533647399));
#26434=CARTESIAN_POINT('Ctrl Pts',(-0.744021445433764,-1.,1.7226822991693));
#26435=CARTESIAN_POINT('Ctrl Pts',(-0.740795162032088,-1.,1.71447789751927));
#26436=CARTESIAN_POINT('Ctrl Pts',(-0.736799665724771,-1.,1.70473309006121));
#26437=CARTESIAN_POINT('Ctrl Pts',(-0.731963238697195,-1.,1.69326921975743));
#26438=CARTESIAN_POINT('Ctrl Pts',(-0.726235967997433,-1.,1.67996158455503));
#26439=CARTESIAN_POINT('Ctrl Pts',(-0.719585433804282,-1.,1.6647288055568));
#26440=CARTESIAN_POINT('Ctrl Pts',(-0.711993139355394,-1.,1.64752408832016));
#26441=CARTESIAN_POINT('Ctrl Pts',(-0.705159151988319,-1.,1.63216541664676));
#26442=CARTESIAN_POINT('Ctrl Pts',(-0.699605146405088,-1.,1.61974673472612));
#26443=CARTESIAN_POINT('Ctrl Pts',(-0.695712097881194,-1.,1.61106790958151));
#26444=CARTESIAN_POINT('Ctrl Pts',(-0.693717979106306,-1.,1.60662857109684));
#26445=CARTESIAN_POINT('',(-0.892032620296855,-1.,1.5055822144029));
#26446=CARTESIAN_POINT('Origin',(0.,-1.,0.));
#26447=CARTESIAN_POINT('',(-1.23627494547115,-1.,1.81978687191668));
#26448=CARTESIAN_POINT('Ctrl Pts',(-0.892032620296855,-1.,1.5055822144029));
#26449=CARTESIAN_POINT('Ctrl Pts',(-0.894452006964543,-1.,1.50980486806688));
#26450=CARTESIAN_POINT('Ctrl Pts',(-0.899185047483511,-1.,1.51805569590094));
#26451=CARTESIAN_POINT('Ctrl Pts',(-0.905967409625651,-1.,1.52984849887993));
#26452=CARTESIAN_POINT('Ctrl Pts',(-0.914375919026456,-1.,1.54440491149498));
#26453=CARTESIAN_POINT('Ctrl Pts',(-0.923832188944341,-1.,1.56065988578893));
#26454=CARTESIAN_POINT('Ctrl Pts',(-0.932246680108685,-1.,1.57499388382243));
#26455=CARTESIAN_POINT('Ctrl Pts',(-0.939646377893399,-1.,1.58744937487176));
#26456=CARTESIAN_POINT('Ctrl Pts',(-0.946078063315257,-1.,1.59810042043673));
#26457=CARTESIAN_POINT('Ctrl Pts',(-0.951613284356035,-1.,1.60706069896936));
#26458=CARTESIAN_POINT('Ctrl Pts',(-0.956354422920671,-1.,1.61449324337085));
#26459=CARTESIAN_POINT('Ctrl Pts',(-0.960438326101729,-1.,1.62061638140221));
#26460=CARTESIAN_POINT('Ctrl Pts',(-0.964046107040536,-1.,1.62571930670187));
#26461=CARTESIAN_POINT('Ctrl Pts',(-0.967387853230345,-1.,1.63013849959461));
#26462=CARTESIAN_POINT('Ctrl Pts',(-0.970669715997509,-1.,1.63420665729798));
#26463=CARTESIAN_POINT('Ctrl Pts',(-0.974066058287418,-1.,1.63820952658144));
#26464=CARTESIAN_POINT('Ctrl Pts',(-0.977689794119416,-1.,1.64233990826687));
#26465=CARTESIAN_POINT('Ctrl Pts',(-0.981562530939489,-1.,1.64665139190656));
#26466=CARTESIAN_POINT('Ctrl Pts',(-0.985642622920821,-1.,1.65110016612638));
#26467=CARTESIAN_POINT('Ctrl Pts',(-0.989855627854165,-1.,1.65559044289699));
#26468=CARTESIAN_POINT('Ctrl Pts',(-0.994121836661306,-1.,1.66001553809947));
#26469=CARTESIAN_POINT('Ctrl Pts',(-0.998389654952758,-1.,1.66430758030376));
#26470=CARTESIAN_POINT('Ctrl Pts',(-1.00265091003727,-1.,1.66846059277303));
#26471=CARTESIAN_POINT('Ctrl Pts',(-1.00692206696414,-1.,1.67250335383293));
#26472=CARTESIAN_POINT('Ctrl Pts',(-1.01123236493511,-1.,1.67648246776464));
#26473=CARTESIAN_POINT('Ctrl Pts',(-1.01561026162773,-1.,1.68044289894798));
#26474=CARTESIAN_POINT('Ctrl Pts',(-1.02006795074201,-1.,1.68440578021706));
#26475=CARTESIAN_POINT('Ctrl Pts',(-1.02460180535255,-1.,1.68836910178447));
#26476=CARTESIAN_POINT('Ctrl Pts',(-1.02919977579147,-1.,1.69231840863458));
#26477=CARTESIAN_POINT('Ctrl Pts',(-1.03384646003588,-1.,1.69623414782771));
#26478=CARTESIAN_POINT('Ctrl Pts',(-1.03852922490789,-1.,1.70010052930962));
#26479=CARTESIAN_POINT('Ctrl Pts',(-1.04324363334554,-1.,1.70391338707982));
#26480=CARTESIAN_POINT('Ctrl Pts',(-1.04799085404995,-1.,1.70767646263649));
#26481=CARTESIAN_POINT('Ctrl Pts',(-1.05277517202855,-1.,1.71139783543989));
#26482=CARTESIAN_POINT('Ctrl Pts',(-1.05760163192479,-1.,1.7150865442702));
#26483=CARTESIAN_POINT('Ctrl Pts',(-1.06247324680647,-1.,1.71874858456904));
#26484=CARTESIAN_POINT('Ctrl Pts',(-1.06738966975462,-1.,1.72238500928453));
#26485=CARTESIAN_POINT('Ctrl Pts',(-1.07234866990252,-1.,1.72599406198488));
#26486=CARTESIAN_POINT('Ctrl Pts',(-1.0773470373727,-1.,1.72957248977424));
#26487=CARTESIAN_POINT('Ctrl Pts',(-1.08238162784749,-1.,1.73311705663407));
#26488=CARTESIAN_POINT('Ctrl Pts',(-1.08745056285427,-1.,1.73662628326091));
#26489=CARTESIAN_POINT('Ctrl Pts',(-1.09255329056493,-1.,1.74010053962247));
#26490=CARTESIAN_POINT('Ctrl Pts',(-1.09768999241225,-1.,1.74354119236208));
#26491=CARTESIAN_POINT('Ctrl Pts',(-1.10286118991143,-1.,1.74695004214923));
#26492=CARTESIAN_POINT('Ctrl Pts',(-1.10806728183007,-1.,1.7503286607592));
#26493=CARTESIAN_POINT('Ctrl Pts',(-1.11330807582551,-1.,1.7536777209463));
#26494=CARTESIAN_POINT('Ctrl Pts',(-1.11858293216763,-1.,1.75699720772105));
#26495=CARTESIAN_POINT('Ctrl Pts',(-1.12389096855086,-1.,1.76028671825096));
#26496=CARTESIAN_POINT('Ctrl Pts',(-1.12923123555075,-1.,1.7635457196617));
#26497=CARTESIAN_POINT('Ctrl Pts',(-1.1346029180462,-1.,1.76677384551862));
#26498=CARTESIAN_POINT('Ctrl Pts',(-1.14000548336975,-1.,1.76997111386769));
#26499=CARTESIAN_POINT('Ctrl Pts',(-1.1454385822692,-1.,1.77313777896194));
#26500=CARTESIAN_POINT('Ctrl Pts',(-1.15090197841515,-1.,1.7762742255701));
#26501=CARTESIAN_POINT('Ctrl Pts',(-1.15639547194698,-1.,1.77938085564275));
#26502=CARTESIAN_POINT('Ctrl Pts',(-1.16191881298499,-1.,1.78245795881009));
#26503=CARTESIAN_POINT('Ctrl Pts',(-1.16747166312303,-1.,1.78550566040443));
#26504=CARTESIAN_POINT('Ctrl Pts',(-1.17305363177328,-1.,1.78852398877616));
#26505=CARTESIAN_POINT('Ctrl Pts',(-1.17866429440809,-1.,1.79151291552689));
#26506=CARTESIAN_POINT('Ctrl Pts',(-1.18430321697432,-1.,1.79447240321515));
#26507=CARTESIAN_POINT('Ctrl Pts',(-1.18996997934445,-1.,1.79740245923478));
#26508=CARTESIAN_POINT('Ctrl Pts',(-1.19566418930242,-1.,1.80030314369879));
#26509=CARTESIAN_POINT('Ctrl Pts',(-1.20138548938974,-1.,1.80317454838603));
#26510=CARTESIAN_POINT('Ctrl Pts',(-1.20713356605475,-1.,1.80601678480707));
#26511=CARTESIAN_POINT('Ctrl Pts',(-1.21290815708314,-1.,1.80882996917129));
#26512=CARTESIAN_POINT('Ctrl Pts',(-1.21870906103557,-1.,1.81161420806656));
#26513=CARTESIAN_POINT('Ctrl Pts',(-1.2245361330495,-1.,1.81436959210434));
#26514=CARTESIAN_POINT('Ctrl Pts',(-1.2292186489137,-1.,1.8165508718364));
#26515=CARTESIAN_POINT('Ctrl Pts',(-1.2327422452705,-1.,1.81817389921279));
#26516=CARTESIAN_POINT('Ctrl Pts',(-1.23509651170476,-1.,1.81925017193666));
#26517=CARTESIAN_POINT('Ctrl Pts',(-1.23627494547115,-1.,1.81978687191668));
#26518=CARTESIAN_POINT('',(-1.34869019493419,-1.,1.73811241238545));
#26519=CARTESIAN_POINT('',(-1.23627494547115,-1.,1.81978687191668));
#26520=CARTESIAN_POINT('',(-1.15624053661742,-1.,1.31362392696032));
#26521=CARTESIAN_POINT('Ctrl Pts',(-1.34869019493419,-1.,1.73811241238545));
#26522=CARTESIAN_POINT('Ctrl Pts',(-1.34854391898045,-1.,1.73682580585691));
#26523=CARTESIAN_POINT('Ctrl Pts',(-1.34824783112887,-1.,1.73425417885907));
#26524=CARTESIAN_POINT('Ctrl Pts',(-1.34779309152035,-1.,1.7304014965394));
#26525=CARTESIAN_POINT('Ctrl Pts',(-1.34716554819527,-1.,1.72527410680674));
#26526=CARTESIAN_POINT('Ctrl Pts',(-1.34634568653227,-1.,1.7188807715049));
#26527=CARTESIAN_POINT('Ctrl Pts',(-1.34549029589416,-1.,1.71250340686822));
#26528=CARTESIAN_POINT('Ctrl Pts',(-1.34459924533831,-1.,1.70614212266738));
#26529=CARTESIAN_POINT('Ctrl Pts',(-1.34367237124483,-1.,1.69979707754427));
#26530=CARTESIAN_POINT('Ctrl Pts',(-1.34270948206319,-1.,1.6934684849687));
#26531=CARTESIAN_POINT('Ctrl Pts',(-1.341710374848,-1.,1.68715660868764));
#26532=CARTESIAN_POINT('Ctrl Pts',(-1.34067485185203,-1.,1.68086176030362));
#26533=CARTESIAN_POINT('Ctrl Pts',(-1.3396027347034,-1.,1.67458429426086));
#26534=CARTESIAN_POINT('Ctrl Pts',(-1.33849388654388,-1.,1.66832460783989));
#26535=CARTESIAN_POINT('Ctrl Pts',(-1.33734820885262,-1.,1.66208312541983));
#26536=CARTESIAN_POINT('Ctrl Pts',(-1.33616559745172,-1.,1.65586025952593));
#26537=CARTESIAN_POINT('Ctrl Pts',(-1.33494590467993,-1.,1.6496563728683));
#26538=CARTESIAN_POINT('Ctrl Pts',(-1.33368890676572,-1.,1.6434717485603));
#26539=CARTESIAN_POINT('Ctrl Pts',(-1.33239425103724,-1.,1.63730653475089));
#26540=CARTESIAN_POINT('Ctrl Pts',(-1.33106149345645,-1.,1.63116079730923));
#26541=CARTESIAN_POINT('Ctrl Pts',(-1.3296901950568,-1.,1.62503464209797));
#26542=CARTESIAN_POINT('Ctrl Pts',(-1.32828000610449,-1.,1.61892832270724));
#26543=CARTESIAN_POINT('Ctrl Pts',(-1.32683074483356,-1.,1.6128423401575));
#26544=CARTESIAN_POINT('Ctrl Pts',(-1.32534250785782,-1.,1.60677758290954));
#26545=CARTESIAN_POINT('Ctrl Pts',(-1.32381550858256,-1.,1.60073511858687));
#26546=CARTESIAN_POINT('Ctrl Pts',(-1.32224985747682,-1.,1.59471591079403));
#26547=CARTESIAN_POINT('Ctrl Pts',(-1.32064537110892,-1.,1.58872057258245));
#26548=CARTESIAN_POINT('Ctrl Pts',(-1.31900135021432,-1.,1.58274907898834));
#26549=CARTESIAN_POINT('Ctrl Pts',(-1.31731642317187,-1.,1.5768005650559));
#26550=CARTESIAN_POINT('Ctrl Pts',(-1.31558903860016,-1.,1.57087397835723));
#26551=CARTESIAN_POINT('Ctrl Pts',(-1.31381795281002,-1.,1.56496872402353));
#26552=CARTESIAN_POINT('Ctrl Pts',(-1.31200264341696,-1.,1.55908521254821));
#26553=CARTESIAN_POINT('Ctrl Pts',(-1.31014393684222,-1.,1.55322568759481));
#26554=CARTESIAN_POINT('Ctrl Pts',(-1.30824393907473,-1.,1.54739413957185));
#26555=CARTESIAN_POINT('Ctrl Pts',(-1.30630475189556,-1.,1.54159462645432));
#26556=CARTESIAN_POINT('Ctrl Pts',(-1.30432735639489,-1.,1.53582981268977));
#26557=CARTESIAN_POINT('Ctrl Pts',(-1.30231064395568,-1.,1.53009970283891));
#26558=CARTESIAN_POINT('Ctrl Pts',(-1.30024984366328,-1.,1.52439957861062));
#26559=CARTESIAN_POINT('Ctrl Pts',(-1.29813791800747,-1.,1.51872184912724));
#26560=CARTESIAN_POINT('Ctrl Pts',(-1.29596850710509,-1.,1.51305994241402));
#26561=CARTESIAN_POINT('Ctrl Pts',(-1.29373841372842,-1.,1.50741159078365));
#26562=CARTESIAN_POINT('Ctrl Pts',(-1.29145022885181,-1.,1.50178230149776));
#26563=CARTESIAN_POINT('Ctrl Pts',(-1.28911506584254,-1.,1.49618896881754));
#26564=CARTESIAN_POINT('Ctrl Pts',(-1.2867467611644,-1.,1.4906522831278));
#26565=CARTESIAN_POINT('Ctrl Pts',(-1.28435533880201,-1.,1.4851881711891));
#26566=CARTESIAN_POINT('Ctrl Pts',(-1.28194158939517,-1.,1.47980070347095));
#26567=CARTESIAN_POINT('Ctrl Pts',(-1.2794891824849,-1.,1.4744717526707));
#26568=CARTESIAN_POINT('Ctrl Pts',(-1.27696414831089,-1.,1.46916035917133));
#26569=CARTESIAN_POINT('Ctrl Pts',(-1.27433119897822,-1.,1.46382431332476));
#26570=CARTESIAN_POINT('Ctrl Pts',(-1.27156805265289,-1.,1.45843906294697));
#26571=CARTESIAN_POINT('Ctrl Pts',(-1.2686778680489,-1.,1.45301422764247));
#26572=CARTESIAN_POINT('Ctrl Pts',(-1.26570925118868,-1.,1.44761985001662));
#26573=CARTESIAN_POINT('Ctrl Pts',(-1.26273903323859,-1.,1.44236470511303));
#26574=CARTESIAN_POINT('Ctrl Pts',(-1.25983531012005,-1.,1.43734919180848));
#26575=CARTESIAN_POINT('Ctrl Pts',(-1.25702687965755,-1.,1.43262645609691));
#26576=CARTESIAN_POINT('Ctrl Pts',(-1.25426945222639,-1.,1.42815938799387));
#26577=CARTESIAN_POINT('Ctrl Pts',(-1.2514145557001,-1.,1.42378102115575));
#26578=CARTESIAN_POINT('Ctrl Pts',(-1.24824430986571,-1.,1.41923722596025));
#26579=CARTESIAN_POINT('Ctrl Pts',(-1.24450600513056,-1.,1.41422913175179));
#26580=CARTESIAN_POINT('Ctrl Pts',(-1.23994455029534,-1.,1.40845295531283));
#26581=CARTESIAN_POINT('Ctrl Pts',(-1.23434087290423,-1.,1.40164708206106));
#26582=CARTESIAN_POINT('Ctrl Pts',(-1.22752961899387,-1.,1.39361389568796));
#26583=CARTESIAN_POINT('Ctrl Pts',(-1.21938737280852,-1.,1.38420564527715));
#26584=CARTESIAN_POINT('Ctrl Pts',(-1.20982812925645,-1.,1.37331915607905));
#26585=CARTESIAN_POINT('Ctrl Pts',(-1.1987959077932,-1.,1.36088705043885));
#26586=CARTESIAN_POINT('Ctrl Pts',(-1.18625865667441,-1.,1.34687054001093));
#26587=CARTESIAN_POINT('Ctrl Pts',(-1.17501305789857,-1.,1.33437539347008));
#26588=CARTESIAN_POINT('Ctrl Pts',(-1.16589330093588,-1.,1.32428080721772));
#26589=CARTESIAN_POINT('Ctrl Pts',(-1.15950888730809,-1.,1.31722977216397));
#26590=CARTESIAN_POINT('Ctrl Pts',(-1.15624053661742,-1.,1.31362392696032));
#26591=CARTESIAN_POINT('',(-1.31362392696033,-1.,1.15624053661742));
#26592=CARTESIAN_POINT('Origin',(0.,-1.,0.));
#26593=CARTESIAN_POINT('',(-1.73811241238545,-1.,1.34869019493419));
#26594=CARTESIAN_POINT('Ctrl Pts',(-1.31362392696033,-1.,1.15624053661742));
#26595=CARTESIAN_POINT('Ctrl Pts',(-1.3172297721596,-1.,1.15950888730433));
#26596=CARTESIAN_POINT('Ctrl Pts',(-1.32428080720544,-1.,1.16589330092532));
#26597=CARTESIAN_POINT('Ctrl Pts',(-1.33437539344842,-1.,1.17501305787994));
#26598=CARTESIAN_POINT('Ctrl Pts',(-1.34687053998157,-1.,1.18625865664915));
#26599=CARTESIAN_POINT('Ctrl Pts',(-1.36088705040677,-1.,1.1987959077656));
#26600=CARTESIAN_POINT('Ctrl Pts',(-1.37331915604962,-1.,1.20982812923113));
#26601=CARTESIAN_POINT('Ctrl Pts',(-1.38420564525391,-1.,1.21938737278853));
#26602=CARTESIAN_POINT('Ctrl Pts',(-1.39361389567257,-1.,1.22752961898063));
#26603=CARTESIAN_POINT('Ctrl Pts',(-1.40164708205345,-1.,1.23434087289768));
#26604=CARTESIAN_POINT('Ctrl Pts',(-1.40845295531151,-1.,1.23994455029421));
#26605=CARTESIAN_POINT('Ctrl Pts',(-1.41422913175437,-1.,1.24450600513278));
#26606=CARTESIAN_POINT('Ctrl Pts',(-1.41923722596421,-1.,1.24824430986911));
#26607=CARTESIAN_POINT('Ctrl Pts',(-1.42378102115911,-1.,1.25141455570299));
#26608=CARTESIAN_POINT('Ctrl Pts',(-1.42815938799555,-1.,1.25426945222783));
#26609=CARTESIAN_POINT('Ctrl Pts',(-1.43262645609679,-1.,1.25702687965744));
#26610=CARTESIAN_POINT('Ctrl Pts',(-1.43734919180719,-1.,1.25983531011894));
#26611=CARTESIAN_POINT('Ctrl Pts',(-1.44236470511145,-1.,1.26273903323723));
#26612=CARTESIAN_POINT('Ctrl Pts',(-1.44761985001544,-1.,1.26570925118767));
#26613=CARTESIAN_POINT('Ctrl Pts',(-1.45301422764205,-1.,1.26867786804854));
#26614=CARTESIAN_POINT('Ctrl Pts',(-1.45843906294725,-1.,1.27156805265312));
#26615=CARTESIAN_POINT('Ctrl Pts',(-1.4638243133254,-1.,1.27433119897877));
#26616=CARTESIAN_POINT('Ctrl Pts',(-1.46916035917197,-1.,1.27696414831144));
#26617=CARTESIAN_POINT('Ctrl Pts',(-1.4744717526711,-1.,1.27948918248524));
#26618=CARTESIAN_POINT('Ctrl Pts',(-1.47980070347102,-1.,1.28194158939522));
#26619=CARTESIAN_POINT('Ctrl Pts',(-1.48518817118891,-1.,1.28435533880184));
#26620=CARTESIAN_POINT('Ctrl Pts',(-1.4906522831275,-1.,1.28674676116415));
#26621=CARTESIAN_POINT('Ctrl Pts',(-1.49618896881729,-1.,1.28911506584232));
#26622=CARTESIAN_POINT('Ctrl Pts',(-1.50178230149764,-1.,1.29145022885171));
#26623=CARTESIAN_POINT('Ctrl Pts',(-1.50741159078367,-1.,1.29373841372843));
#26624=CARTESIAN_POINT('Ctrl Pts',(-1.51305994241412,-1.,1.29596850710518));
#26625=CARTESIAN_POINT('Ctrl Pts',(-1.51872184912735,-1.,1.29813791800757));
#26626=CARTESIAN_POINT('Ctrl Pts',(-1.5243995786107,-1.,1.30024984366334));
#26627=CARTESIAN_POINT('Ctrl Pts',(-1.53009970283893,-1.,1.3023106439557));
#26628=CARTESIAN_POINT('Ctrl Pts',(-1.53582981268976,-1.,1.30432735639487));
#26629=CARTESIAN_POINT('Ctrl Pts',(-1.54159462645428,-1.,1.30630475189553));
#26630=CARTESIAN_POINT('Ctrl Pts',(-1.54739413957183,-1.,1.30824393907471));
#26631=CARTESIAN_POINT('Ctrl Pts',(-1.55322568759481,-1.,1.31014393684221));
#26632=CARTESIAN_POINT('Ctrl Pts',(-1.55908521254822,-1.,1.31200264341696));
#26633=CARTESIAN_POINT('Ctrl Pts',(-1.56496872402352,-1.,1.31381795281002));
#26634=CARTESIAN_POINT('Ctrl Pts',(-1.57087397835721,-1.,1.31558903860015));
#26635=CARTESIAN_POINT('Ctrl Pts',(-1.57680056505585,-1.,1.31731642317183));
#26636=CARTESIAN_POINT('Ctrl Pts',(-1.58274907898829,-1.,1.31900135021428));
#26637=CARTESIAN_POINT('Ctrl Pts',(-1.58872057258244,-1.,1.32064537110891));
#26638=CARTESIAN_POINT('Ctrl Pts',(-1.59471591079408,-1.,1.32224985747686));
#26639=CARTESIAN_POINT('Ctrl Pts',(-1.600735118587,-1.,1.32381550858266));
#26640=CARTESIAN_POINT('Ctrl Pts',(-1.6067775829097,-1.,1.32534250785794));
#26641=CARTESIAN_POINT('Ctrl Pts',(-1.61284234015762,-1.,1.32683074483365));
#26642=CARTESIAN_POINT('Ctrl Pts',(-1.61892832270723,-1.,1.32828000610448));
#26643=CARTESIAN_POINT('Ctrl Pts',(-1.62503464209777,-1.,1.32969019505665));
#26644=CARTESIAN_POINT('Ctrl Pts',(-1.63116079730887,-1.,1.33106149345618));
#26645=CARTESIAN_POINT('Ctrl Pts',(-1.6373065347505,-1.,1.33239425103694));
#26646=CARTESIAN_POINT('Ctrl Pts',(-1.64347174856007,-1.,1.33368890676554));
#26647=CARTESIAN_POINT('Ctrl Pts',(-1.64965637286843,-1.,1.33494590468003));
#26648=CARTESIAN_POINT('Ctrl Pts',(-1.65586025952651,-1.,1.33616559745217));
#26649=CARTESIAN_POINT('Ctrl Pts',(-1.66208312542073,-1.,1.33734820885331));
#26650=CARTESIAN_POINT('Ctrl Pts',(-1.66832460784078,-1.,1.33849388654458));
#26651=CARTESIAN_POINT('Ctrl Pts',(-1.67458429426126,-1.,1.33960273470372));
#26652=CARTESIAN_POINT('Ctrl Pts',(-1.68086176030308,-1.,1.3406748518516));
#26653=CARTESIAN_POINT('Ctrl Pts',(-1.68715660868602,-1.,1.34171037484673));
#26654=CARTESIAN_POINT('Ctrl Pts',(-1.6934684849664,-1.,1.34270948206139));
#26655=CARTESIAN_POINT('Ctrl Pts',(-1.69979707754221,-1.,1.34367237124322));
#26656=CARTESIAN_POINT('Ctrl Pts',(-1.70614212266676,-1.,1.34459924533783));
#26657=CARTESIAN_POINT('Ctrl Pts',(-1.71250340687011,-1.,1.34549029589563));
#26658=CARTESIAN_POINT('Ctrl Pts',(-1.7188807715095,-1.,1.34634568653586));
#26659=CARTESIAN_POINT('Ctrl Pts',(-1.72527410681298,-1.,1.34716554820013));
#26660=CARTESIAN_POINT('Ctrl Pts',(-1.73040149654497,-1.,1.3477930915247));
#26661=CARTESIAN_POINT('Ctrl Pts',(-1.73425417886255,-1.,1.34824783113158));
#26662=CARTESIAN_POINT('Ctrl Pts',(-1.73682580585819,-1.,1.34854391898145));
#26663=CARTESIAN_POINT('Ctrl Pts',(-1.73811241238545,-1.,1.34869019493419));
#26664=CARTESIAN_POINT('',(-1.81978687191668,-1.,1.23627494547115));
#26665=CARTESIAN_POINT('',(-1.73811241238545,-1.,1.34869019493419));
#26666=CARTESIAN_POINT('',(-1.5055822144029,-1.,0.892032620296855));
#26667=CARTESIAN_POINT('Ctrl Pts',(-1.81978687191668,-1.,1.23627494547115));
#26668=CARTESIAN_POINT('Ctrl Pts',(-1.81925017193531,-1.,1.23509651170384));
#26669=CARTESIAN_POINT('Ctrl Pts',(-1.81817389920914,-1.,1.23274224526804));
#26670=CARTESIAN_POINT('Ctrl Pts',(-1.81655087183054,-1.,1.22921864890975));
#26671=CARTESIAN_POINT('Ctrl Pts',(-1.81436959209778,-1.,1.22453613304507));
#26672=CARTESIAN_POINT('Ctrl Pts',(-1.81161420806172,-1.,1.2187090610323));
#26673=CARTESIAN_POINT('Ctrl Pts',(-1.80882996916931,-1.,1.2129081570818));
#26674=CARTESIAN_POINT('Ctrl Pts',(-1.80601678480772,-1.,1.20713356605519));
#26675=CARTESIAN_POINT('Ctrl Pts',(-1.8031745483882,-1.,1.2013854893912));
#26676=CARTESIAN_POINT('Ctrl Pts',(-1.80030314370121,-1.,1.19566418930405));
#26677=CARTESIAN_POINT('Ctrl Pts',(-1.79740245923649,-1.,1.1899699793456));
#26678=CARTESIAN_POINT('Ctrl Pts',(-1.79447240321572,-1.,1.18430321697471));
#26679=CARTESIAN_POINT('Ctrl Pts',(-1.79151291552646,-1.,1.17866429440781));
#26680=CARTESIAN_POINT('Ctrl Pts',(-1.78852398877523,-1.,1.17305363177265));
#26681=CARTESIAN_POINT('Ctrl Pts',(-1.78550566040349,-1.,1.16747166312239));
#26682=CARTESIAN_POINT('Ctrl Pts',(-1.78245795880949,-1.,1.16191881298458));
#26683=CARTESIAN_POINT('Ctrl Pts',(-1.77938085564261,-1.,1.15639547194689));
#26684=CARTESIAN_POINT('Ctrl Pts',(-1.77627422557034,-1.,1.15090197841531));
#26685=CARTESIAN_POINT('Ctrl Pts',(-1.77313777896234,-1.,1.14543858226948));
#26686=CARTESIAN_POINT('Ctrl Pts',(-1.76997111386806,-1.,1.14000548337));
#26687=CARTESIAN_POINT('Ctrl Pts',(-1.76677384551883,-1.,1.13460291804635));
#26688=CARTESIAN_POINT('Ctrl Pts',(-1.76354571966171,-1.,1.12923123555076));
#26689=CARTESIAN_POINT('Ctrl Pts',(-1.76028671825084,-1.,1.12389096855078));
#26690=CARTESIAN_POINT('Ctrl Pts',(-1.75699720772089,-1.,1.11858293216752));
#26691=CARTESIAN_POINT('Ctrl Pts',(-1.75367772094617,-1.,1.11330807582542));
#26692=CARTESIAN_POINT('Ctrl Pts',(-1.75032866075914,-1.,1.10806728183003));
#26693=CARTESIAN_POINT('Ctrl Pts',(-1.74695004214924,-1.,1.10286118991144));
#26694=CARTESIAN_POINT('Ctrl Pts',(-1.74354119236212,-1.,1.09768999241229));
#26695=CARTESIAN_POINT('Ctrl Pts',(-1.74010053962252,-1.,1.09255329056496));
#26696=CARTESIAN_POINT('Ctrl Pts',(-1.73662628326093,-1.,1.08745056285429));
#26697=CARTESIAN_POINT('Ctrl Pts',(-1.73311705663407,-1.,1.08238162784749));
#26698=CARTESIAN_POINT('Ctrl Pts',(-1.72957248977424,-1.,1.0773470373727));
#26699=CARTESIAN_POINT('Ctrl Pts',(-1.72599406198489,-1.,1.07234866990252));
#26700=CARTESIAN_POINT('Ctrl Pts',(-1.72238500928456,-1.,1.06738966975463));
#26701=CARTESIAN_POINT('Ctrl Pts',(-1.71874858456908,-1.,1.0624732468065));
#26702=CARTESIAN_POINT('Ctrl Pts',(-1.71508654427022,-1.,1.05760163192481));
#26703=CARTESIAN_POINT('Ctrl Pts',(-1.71139783543986,-1.,1.05277517202854));
#26704=CARTESIAN_POINT('Ctrl Pts',(-1.70767646263641,-1.,1.0479908540499));
#26705=CARTESIAN_POINT('Ctrl Pts',(-1.70391338707969,-1.,1.04324363334546));
#26706=CARTESIAN_POINT('Ctrl Pts',(-1.70010052930951,-1.,1.03852922490782));
#26707=CARTESIAN_POINT('Ctrl Pts',(-1.69623414782769,-1.,1.03384646003587));
#26708=CARTESIAN_POINT('Ctrl Pts',(-1.69231840863471,-1.,1.02919977579155));
#26709=CARTESIAN_POINT('Ctrl Pts',(-1.68836910178475,-1.,1.02460180535272));
#26710=CARTESIAN_POINT('Ctrl Pts',(-1.68440578021739,-1.,1.02006795074222));
#26711=CARTESIAN_POINT('Ctrl Pts',(-1.6804428989482,-1.,1.01561026162787));
#26712=CARTESIAN_POINT('Ctrl Pts',(-1.67648246776457,-1.,1.01123236493507));
#26713=CARTESIAN_POINT('Ctrl Pts',(-1.67250335383248,-1.,1.00692206696387));
#26714=CARTESIAN_POINT('Ctrl Pts',(-1.66846059277231,-1.,1.00265091003682));
#26715=CARTESIAN_POINT('Ctrl Pts',(-1.66430758030304,-1.,0.998389654952317));
#26716=CARTESIAN_POINT('Ctrl Pts',(-1.66001553809916,-1.,0.994121836661116));
#26717=CARTESIAN_POINT('Ctrl Pts',(-1.65559044289746,-1.,0.98985562785445));
#26718=CARTESIAN_POINT('Ctrl Pts',(-1.6511001661277,-1.,0.985642622921626));
#26719=CARTESIAN_POINT('Ctrl Pts',(-1.64665139190834,-1.,0.981562530940574));
#26720=CARTESIAN_POINT('Ctrl Pts',(-1.64233990826831,-1.,0.977689794120297));
#26721=CARTESIAN_POINT('Ctrl Pts',(-1.63820952658157,-1.,0.974066058287501));
#26722=CARTESIAN_POINT('Ctrl Pts',(-1.63420665729609,-1.,0.970669715996356));
#26723=CARTESIAN_POINT('Ctrl Pts',(-1.63013849959083,-1.,0.967387853228041));
#26724=CARTESIAN_POINT('Ctrl Pts',(-1.6257193066974,-1.,0.964046107037821));
#26725=CARTESIAN_POINT('Ctrl Pts',(-1.62061638139929,-1.,0.960438326099958));
#26726=CARTESIAN_POINT('Ctrl Pts',(-1.61449324337233,-1.,0.956354422921573));
#26727=CARTESIAN_POINT('Ctrl Pts',(-1.60706069897794,-1.,0.951613284361248));
#26728=CARTESIAN_POINT('Ctrl Pts',(-1.59810042045408,-1.,0.946078063325796));
#26729=CARTESIAN_POINT('Ctrl Pts',(-1.58744937489796,-1.,0.939646377909319));
#26730=CARTESIAN_POINT('Ctrl Pts',(-1.57499388385561,-1.,0.932246680128849));
#26731=CARTESIAN_POINT('Ctrl Pts',(-1.56065988582509,-1.,0.923832188966322));
#26732=CARTESIAN_POINT('Ctrl Pts',(-1.54440491152808,-1.,0.91437591904658));
#26733=CARTESIAN_POINT('Ctrl Pts',(-1.52984849890434,-1.,0.905967409640499));
#26734=CARTESIAN_POINT('Ctrl Pts',(-1.51805569591479,-1.,0.89918504749193));
#26735=CARTESIAN_POINT('Ctrl Pts',(-1.50980486807181,-1.,0.894452006967538));
#26736=CARTESIAN_POINT('Ctrl Pts',(-1.5055822144029,-1.,0.892032620296855));
#26737=CARTESIAN_POINT('',(-1.60662857109684,-1.,0.693717979106305));
#26738=CARTESIAN_POINT('Origin',(0.,-1.,0.));
#26739=CARTESIAN_POINT('',(-2.0698113262342,-1.,0.7455743247944));
#26740=CARTESIAN_POINT('Ctrl Pts',(-1.60662857109684,-1.,0.693717979106305));
#26741=CARTESIAN_POINT('Ctrl Pts',(-1.61106790957619,-1.,0.69571209787897));
#26742=CARTESIAN_POINT('Ctrl Pts',(-1.61974673471117,-1.,0.699605146398837));
#26743=CARTESIAN_POINT('Ctrl Pts',(-1.6321654166204,-1.,0.705159151977294));
#26744=CARTESIAN_POINT('Ctrl Pts',(-1.64752408828442,-1.,0.711993139340447));
#26745=CARTESIAN_POINT('Ctrl Pts',(-1.66472880551777,-1.,0.71958543378795));
#26746=CARTESIAN_POINT('Ctrl Pts',(-1.67996158451922,-1.,0.726235967982445));
#26747=CARTESIAN_POINT('Ctrl Pts',(-1.69326921972915,-1.,0.731963238685357));
#26748=CARTESIAN_POINT('Ctrl Pts',(-1.70473309004249,-1.,0.736799665716932));
#26749=CARTESIAN_POINT('Ctrl Pts',(-1.71447789751001,-1.,0.74079516202821));
#26750=CARTESIAN_POINT('Ctrl Pts',(-1.72268229916769,-1.,0.744021445433093));
#26751=CARTESIAN_POINT('Ctrl Pts',(-1.72958533647714,-1.,0.746574710097752));
#26752=CARTESIAN_POINT('Ctrl Pts',(-1.7355035168033,-1.,0.74858246295687));
#26753=CARTESIAN_POINT('Ctrl Pts',(-1.74080458267114,-1.,0.750193435981249));
#26754=CARTESIAN_POINT('Ctrl Pts',(-1.74585086852502,-1.,0.751555614164482));
#26755=CARTESIAN_POINT('Ctrl Pts',(-1.75095139468794,-1.,0.752797683531314));
#26756=CARTESIAN_POINT('Ctrl Pts',(-1.75631083600019,-1.,0.754009254027829));
#26757=CARTESIAN_POINT('Ctrl Pts',(-1.76197817240128,-1.,0.755220979974461));
#26758=CARTESIAN_POINT('Ctrl Pts',(-1.76789396002998,-1.,0.75642189602781));
#26759=CARTESIAN_POINT('Ctrl Pts',(-1.77394167108292,-1.,0.757578264077029));
#26760=CARTESIAN_POINT('Ctrl Pts',(-1.77999411220945,-1.,0.758650626677518));
#26761=CARTESIAN_POINT('Ctrl Pts',(-1.78596964884604,-1.,0.759614401110189));
#26762=CARTESIAN_POINT('Ctrl Pts',(-1.7918581561088,-1.,0.760469555880749));
#26763=CARTESIAN_POINT('Ctrl Pts',(-1.79768986997783,-1.,0.761229695230558));
#26764=CARTESIAN_POINT('Ctrl Pts',(-1.80351583877342,-1.,0.761915336443547));
#26765=CARTESIAN_POINT('Ctrl Pts',(-1.80938551463965,-1.,0.762546129463938));
#26766=CARTESIAN_POINT('Ctrl Pts',(-1.8153211840553,-1.,0.763132003836634));
#26767=CARTESIAN_POINT('Ctrl Pts',(-1.82131873145266,-1.,0.763673465462726));
#26768=CARTESIAN_POINT('Ctrl Pts',(-1.82735991200065,-1.,0.764165902605995));
#26769=CARTESIAN_POINT('Ctrl Pts',(-1.83342077227142,-1.,0.764602549687853));
#26770=CARTESIAN_POINT('Ctrl Pts',(-1.83948181064835,-1.,0.764978057881737));
#26771=CARTESIAN_POINT('Ctrl Pts',(-1.84553698875924,-1.,0.765291664862029));
#26772=CARTESIAN_POINT('Ctrl Pts',(-1.85158945130063,-1.,0.765545710619062));
#26773=CARTESIAN_POINT('Ctrl Pts',(-1.85764741390394,-1.,0.765744212909318));
#26774=CARTESIAN_POINT('Ctrl Pts',(-1.86372027063312,-1.,0.765891519092547));
#26775=CARTESIAN_POINT('Ctrl Pts',(-1.86981398314341,-1.,0.765990708546091));
#26776=CARTESIAN_POINT('Ctrl Pts',(-1.87592888967883,-1.,0.766042837036744));
#26777=CARTESIAN_POINT('Ctrl Pts',(-1.88206215302561,-1.,0.766047794851864));
#26778=CARTESIAN_POINT('Ctrl Pts',(-1.88820926433409,-1.,0.766004837062091));
#26779=CARTESIAN_POINT('Ctrl Pts',(-1.89436577771388,-1.,0.765913193856978));
#26780=CARTESIAN_POINT('Ctrl Pts',(-1.90052930393596,-1.,0.765772772593386));
#26781=CARTESIAN_POINT('Ctrl Pts',(-1.90669961402356,-1.,0.765584196937919));
#26782=CARTESIAN_POINT('Ctrl Pts',(-1.91287765805169,-1.,0.765348465884722));
#26783=CARTESIAN_POINT('Ctrl Pts',(-1.91906491634196,-1.,0.765066729667088));
#26784=CARTESIAN_POINT('Ctrl Pts',(-1.92526263537048,-1.,0.764740025488211));
#26785=CARTESIAN_POINT('Ctrl Pts',(-1.93147105496382,-1.,0.76436901067394));
#26786=CARTESIAN_POINT('Ctrl Pts',(-1.93768964875886,-1.,0.763954049121458));
#26787=CARTESIAN_POINT('Ctrl Pts',(-1.9439174661764,-1.,0.763495333538629));
#26788=CARTESIAN_POINT('Ctrl Pts',(-1.95015342590024,-1.,0.762992990878769));
#26789=CARTESIAN_POINT('Ctrl Pts',(-1.95639665309869,-1.,0.762447203806179));
#26790=CARTESIAN_POINT('Ctrl Pts',(-1.96264672744186,-1.,0.761858300014423));
#26791=CARTESIAN_POINT('Ctrl Pts',(-1.96890351582499,-1.,0.76122669048382));
#26792=CARTESIAN_POINT('Ctrl Pts',(-1.97516705321494,-1.,0.760552825409757));
#26793=CARTESIAN_POINT('Ctrl Pts',(-1.98143741418172,-1.,0.75983714745219));
#26794=CARTESIAN_POINT('Ctrl Pts',(-1.98771456680874,-1.,0.759080037802488));
#26795=CARTESIAN_POINT('Ctrl Pts',(-1.99399831098817,-1.,0.758281796766761));
#26796=CARTESIAN_POINT('Ctrl Pts',(-2.00028834739178,-1.,0.757442676862724));
#26797=CARTESIAN_POINT('Ctrl Pts',(-2.0065843158773,-1.,0.75656290464667));
#26798=CARTESIAN_POINT('Ctrl Pts',(-2.01288584328084,-1.,0.755642704957865));
#26799=CARTESIAN_POINT('Ctrl Pts',(-2.01919259405809,-1.,0.754682330722816));
#26800=CARTESIAN_POINT('Ctrl Pts',(-2.02550428623313,-1.,0.753682061112768));
#26801=CARTESIAN_POINT('Ctrl Pts',(-2.03182068456221,-1.,0.752642180487211));
#26802=CARTESIAN_POINT('Ctrl Pts',(-2.03814160092099,-1.,0.751562963361115));
#26803=CARTESIAN_POINT('Ctrl Pts',(-2.04446689147979,-1.,0.750444657875576));
#26804=CARTESIAN_POINT('Ctrl Pts',(-2.05079645592154,-1.,0.749287468665046));
#26805=CARTESIAN_POINT('Ctrl Pts',(-2.05713023031006,-1.,0.748091554183802));
#26806=CARTESIAN_POINT('Ctrl Pts',(-2.06220058927826,-1.,0.747103932787919));
#26807=CARTESIAN_POINT('Ctrl Pts',(-2.06600523016815,-1.,0.7463458715442));
#26808=CARTESIAN_POINT('Ctrl Pts',(-2.06854248895728,-1.,0.745832791378367));
#26809=CARTESIAN_POINT('Ctrl Pts',(-2.0698113262342,-1.,0.7455743247944));
#26810=CARTESIAN_POINT('',(-2.11275013067528,-1.,0.61342227326009));
#26811=CARTESIAN_POINT('',(-2.0698113262342,-1.,0.7455743247944));
#26812=CARTESIAN_POINT('',(-1.7075470150345,-1.,0.383122945602004));
#26813=CARTESIAN_POINT('Ctrl Pts',(-2.11275013067528,-1.,0.61342227326009));
#26814=CARTESIAN_POINT('Ctrl Pts',(-2.11187554259986,-1.,0.6124673655618));
#26815=CARTESIAN_POINT('Ctrl Pts',(-2.11012443807238,-1.,0.610560911689899));
#26816=CARTESIAN_POINT('Ctrl Pts',(-2.1074919961518,-1.,0.607711315454876));
#26817=CARTESIAN_POINT('Ctrl Pts',(-2.10397049886949,-1.,0.60393203073603));
#26818=CARTESIAN_POINT('Ctrl Pts',(-2.0995493086477,-1.,0.599241616420533));
#26819=CARTESIAN_POINT('Ctrl Pts',(-2.0951087622027,-1.,0.594585006052162));
#26820=CARTESIAN_POINT('Ctrl Pts',(-2.09064881812129,-1.,0.589962365403406));
#26821=CARTESIAN_POINT('Ctrl Pts',(-2.08616943727951,-1.,0.585373918991617));
#26822=CARTESIAN_POINT('Ctrl Pts',(-2.08167059018418,-1.,0.580819952108063));
#26823=CARTESIAN_POINT('Ctrl Pts',(-2.07715226767559,-1.,0.576300797416844));
#26824=CARTESIAN_POINT('Ctrl Pts',(-2.07261449292824,-1.,0.571816823242603));
#26825=CARTESIAN_POINT('Ctrl Pts',(-2.06805732997334,-1.,0.567368421181087));
#26826=CARTESIAN_POINT('Ctrl Pts',(-2.06348090160589,-1.,0.562955993082261));
#26827=CARTESIAN_POINT('Ctrl Pts',(-2.05888537756462,-1.,0.558579940185151));
#26828=CARTESIAN_POINT('Ctrl Pts',(-2.05427091604413,-1.,0.554240657463906));
#26829=CARTESIAN_POINT('Ctrl Pts',(-2.04963761077958,-1.,0.549938525150295));
#26830=CARTESIAN_POINT('Ctrl Pts',(-2.04498544714588,-1.,0.54567390381743));
#26831=CARTESIAN_POINT('Ctrl Pts',(-2.04031422690527,-1.,0.541447120615659));
#26832=CARTESIAN_POINT('Ctrl Pts',(-2.03562362954037,-1.,0.537258489833262));
#26833=CARTESIAN_POINT('Ctrl Pts',(-2.03091336214426,-1.,0.533108355132976));
#26834=CARTESIAN_POINT('Ctrl Pts',(-2.0261832908329,-1.,0.528997127241914));
#26835=CARTESIAN_POINT('Ctrl Pts',(-2.02143356304698,-1.,0.524925318333476));
#26836=CARTESIAN_POINT('Ctrl Pts',(-2.01666477917286,-1.,0.52089359039937));
#26837=CARTESIAN_POINT('Ctrl Pts',(-2.01187773939242,-1.,0.516902681728687));
#26838=CARTESIAN_POINT('Ctrl Pts',(-2.00707309946949,-1.,0.512953306961792));
#26839=CARTESIAN_POINT('Ctrl Pts',(-2.00225107134734,-1.,0.509046069886157));
#26840=CARTESIAN_POINT('Ctrl Pts',(-1.99741107463572,-1.,0.505181361323026));
#26841=CARTESIAN_POINT('Ctrl Pts',(-1.99255149126155,-1.,0.501359287727146));
#26842=CARTESIAN_POINT('Ctrl Pts',(-1.98767044752932,-1.,0.497579909545574));
#26843=CARTESIAN_POINT('Ctrl Pts',(-1.98276658761821,-1.,0.493843476541494));
#26844=CARTESIAN_POINT('Ctrl Pts',(-1.97783973019229,-1.,0.490150627860952));
#26845=CARTESIAN_POINT('Ctrl Pts',(-1.97289186263272,-1.,0.486502692907659));
#26846=CARTESIAN_POINT('Ctrl Pts',(-1.96792703422362,-1.,0.48290166212069));
#26847=CARTESIAN_POINT('Ctrl Pts',(-1.96294933055943,-1.,0.479349583074855));
#26848=CARTESIAN_POINT('Ctrl Pts',(-1.95796111148177,-1.,0.475848034683176));
#26849=CARTESIAN_POINT('Ctrl Pts',(-1.95296148278133,-1.,0.472397672264072));
#26850=CARTESIAN_POINT('Ctrl Pts',(-1.94794381136514,-1.,0.468997482913135));
#26851=CARTESIAN_POINT('Ctrl Pts',(-1.9428979419619,-1.,0.46564546202603));
#26852=CARTESIAN_POINT('Ctrl Pts',(-1.93781486640821,-1.,0.462340031009056));
#26853=CARTESIAN_POINT('Ctrl Pts',(-1.93269066517934,-1.,0.459081234547926));
#26854=CARTESIAN_POINT('Ctrl Pts',(-1.92753067150476,-1.,0.455872005174371));
#26855=CARTESIAN_POINT('Ctrl Pts',(-1.92235380648502,-1.,0.452719478359432));
#26856=CARTESIAN_POINT('Ctrl Pts',(-1.91718342555755,-1.,0.449632260106662));
#26857=CARTESIAN_POINT('Ctrl Pts',(-1.9120369998112,-1.,0.446617343485711));
#26858=CARTESIAN_POINT('Ctrl Pts',(-1.90691756144898,-1.,0.44367755684915));
#26859=CARTESIAN_POINT('Ctrl Pts',(-1.90180124389086,-1.,0.440807833704038));
#26860=CARTESIAN_POINT('Ctrl Pts',(-1.89663648956466,-1.,0.437995003948244));
#26861=CARTESIAN_POINT('Ctrl Pts',(-1.89136993975504,-1.,0.435225660963383));
#26862=CARTESIAN_POINT('Ctrl Pts',(-1.88596913666793,-1.,0.432493038548748));
#26863=CARTESIAN_POINT('Ctrl Pts',(-1.88044229001832,-1.,0.429803062482344));
#26864=CARTESIAN_POINT('Ctrl Pts',(-1.87486989291484,-1.,0.427183828519102));
#26865=CARTESIAN_POINT('Ctrl Pts',(-1.86937803944323,-1.,0.424678177291359));
#26866=CARTESIAN_POINT('Ctrl Pts',(-1.86408083334028,-1.,0.422327307418275));
#26867=CARTESIAN_POINT('Ctrl Pts',(-1.85903281096686,-1.,0.420157287975619));
#26868=CARTESIAN_POINT('Ctrl Pts',(-1.85417632856234,-1.,0.418164129143534));
#26869=CARTESIAN_POINT('Ctrl Pts',(-1.84929312929882,-1.,0.416300022038864));
#26870=CARTESIAN_POINT('Ctrl Pts',(-1.8440575707371,-1.,0.41448743825434));
#26871=CARTESIAN_POINT('Ctrl Pts',(-1.83808953475839,-1.,0.412633125322161));
#26872=CARTESIAN_POINT('Ctrl Pts',(-1.83100408895216,-1.,0.410641256301675));
#26873=CARTESIAN_POINT('Ctrl Pts',(-1.8224702267854,-1.,0.408428948108533));
#26874=CARTESIAN_POINT('Ctrl Pts',(-1.81223801813988,-1.,0.405933518411838));
#26875=CARTESIAN_POINT('Ctrl Pts',(-1.80012077176221,-1.,0.403107976170441));
#26876=CARTESIAN_POINT('Ctrl Pts',(-1.78598826347533,-1.,0.39991940378308));
#26877=CARTESIAN_POINT('Ctrl Pts',(-1.7697556004756,-1.,0.39634619612042));
#26878=CARTESIAN_POINT('Ctrl Pts',(-1.75137405313962,-1.,0.392375812294307));
#26879=CARTESIAN_POINT('Ctrl Pts',(-1.7349317097561,-1.,0.388877023509191));
#26880=CARTESIAN_POINT('Ctrl Pts',(-1.72162022246158,-1.,0.38607079032701));
#26881=CARTESIAN_POINT('Ctrl Pts',(-1.71231062891958,-1.,0.384119047315542));
#26882=CARTESIAN_POINT('Ctrl Pts',(-1.7075470150345,-1.,0.383122945602004));
#26883=CARTESIAN_POINT('',(-1.74236521665491,-1.,0.163289472382896));
#26884=CARTESIAN_POINT('Origin',(0.,-1.,0.));
#26885=CARTESIAN_POINT('',(-2.19890268624765,-1.,0.069476445021958));
#26886=CARTESIAN_POINT('Ctrl Pts',(-1.74236521665491,-1.,0.163289472382896));
#26887=CARTESIAN_POINT('Ctrl Pts',(-1.7472034950333,-1.,0.163814161002002));
#26888=CARTESIAN_POINT('Ctrl Pts',(-1.75666056638427,-1.,0.164834765707158));
#26889=CARTESIAN_POINT('Ctrl Pts',(-1.77018771684844,-1.,0.1662793551464));
#26890=CARTESIAN_POINT('Ctrl Pts',(-1.7869064998507,-1.,0.168032772805197));
#26891=CARTESIAN_POINT('Ctrl Pts',(-1.80561530629706,-1.,0.169936923904608));
#26892=CARTESIAN_POINT('Ctrl Pts',(-1.82215766811545,-1.,0.171554770204119));
#26893=CARTESIAN_POINT('Ctrl Pts',(-1.83658380527692,-1.,0.1728894428919));
#26894=CARTESIAN_POINT('Ctrl Pts',(-1.8489811319852,-1.,0.173946627587731));
#26895=CARTESIAN_POINT('Ctrl Pts',(-1.85948367088837,-1.,0.17473525927603));
#26896=CARTESIAN_POINT('Ctrl Pts',(-1.86828349694799,-1.,0.175268337590758));
#26897=CARTESIAN_POINT('Ctrl Pts',(-1.87563767773588,-1.,0.175563480746485));
#26898=CARTESIAN_POINT('Ctrl Pts',(-1.88188663145367,-1.,0.175644148889698));
#26899=CARTESIAN_POINT('Ctrl Pts',(-1.88742606273259,-1.,0.175538155840648));
#26900=CARTESIAN_POINT('Ctrl Pts',(-1.892646301985,-1.,0.175274276190844));
#26901=CARTESIAN_POINT('Ctrl Pts',(-1.89788101117132,-1.,0.174879405091263));
#26902=CARTESIAN_POINT('Ctrl Pts',(-1.90335253862834,-1.,0.174375518661085));
#26903=CARTESIAN_POINT('Ctrl Pts',(-1.90911693975267,-1.,0.173776635257817));
#26904=CARTESIAN_POINT('Ctrl Pts',(-1.91511429159527,-1.,0.173090695383496));
#26905=CARTESIAN_POINT('Ctrl Pts',(-1.9212233439798,-1.,0.172321621259514));
#26906=CARTESIAN_POINT('Ctrl Pts',(-1.92731093582036,-1.,0.171471191532988));
#26907=CARTESIAN_POINT('Ctrl Pts',(-1.93329183155539,-1.,0.170541253116201));
#26908=CARTESIAN_POINT('Ctrl Pts',(-1.93915639211581,-1.,0.169534904817491));
#26909=CARTESIAN_POINT('Ctrl Pts',(-1.94493757756931,-1.,0.168455741607556));
#26910=CARTESIAN_POINT('Ctrl Pts',(-1.95069027794294,-1.,0.167307501784475));
#26911=CARTESIAN_POINT('Ctrl Pts',(-1.9564675971873,-1.,0.166093592002812));
#26912=CARTESIAN_POINT('Ctrl Pts',(-1.96229379940136,-1.,0.164816568920269));
#26913=CARTESIAN_POINT('Ctrl Pts',(-1.96816512677967,-1.,0.163478185457734));
#26914=CARTESIAN_POINT('Ctrl Pts',(-1.97406280235188,-1.,0.162079693556288));
#26915=CARTESIAN_POINT('Ctrl Pts',(-1.97996195437559,-1.,0.160622060784611));
#26916=CARTESIAN_POINT('Ctrl Pts',(-1.98584238283292,-1.,0.159106226437299));
#26917=CARTESIAN_POINT('Ctrl Pts',(-1.99169810931908,-1.,0.157533331459227));
#26918=CARTESIAN_POINT('Ctrl Pts',(-1.99753284771497,-1.,0.155904629548783));
#26919=CARTESIAN_POINT('Ctrl Pts',(-2.00335565310543,-1.,0.154221403049722));
#26920=CARTESIAN_POINT('Ctrl Pts',(-2.00917680318424,-1.,0.15248488362145));
#26921=CARTESIAN_POINT('Ctrl Pts',(-2.01500291940238,-1.,0.150696157673078));
#26922=CARTESIAN_POINT('Ctrl Pts',(-2.02083464969894,-1.,0.148856124775337));
#26923=CARTESIAN_POINT('Ctrl Pts',(-2.02666926182017,-1.,0.146965557332583));
#26924=CARTESIAN_POINT('Ctrl Pts',(-2.03250223739942,-1.,0.145025140186057));
#26925=CARTESIAN_POINT('Ctrl Pts',(-2.03832911025912,-1.,0.143035515058209));
#26926=CARTESIAN_POINT('Ctrl Pts',(-2.04414757947916,-1.,0.140997332152546));
#26927=CARTESIAN_POINT('Ctrl Pts',(-2.04995762001328,-1.,0.138911255368966));
#26928=CARTESIAN_POINT('Ctrl Pts',(-2.05576044414264,-1.,0.136777941218043));
#26929=CARTESIAN_POINT('Ctrl Pts',(-2.06155781517842,-1.,0.134598026192106));
#26930=CARTESIAN_POINT('Ctrl Pts',(-2.06735123910326,-1.,0.13237211154771));
#26931=CARTESIAN_POINT('Ctrl Pts',(-2.07314114713063,-1.,0.130100748328403));
#26932=CARTESIAN_POINT('Ctrl Pts',(-2.07892715110987,-1.,0.12778444527612));
#26933=CARTESIAN_POINT('Ctrl Pts',(-2.08470840653643,-1.,0.125423679412061));
#26934=CARTESIAN_POINT('Ctrl Pts',(-2.09048392424825,-1.,0.123018905621083));
#26935=CARTESIAN_POINT('Ctrl Pts',(-2.0962529286773,-1.,0.120570567965122));
#26936=CARTESIAN_POINT('Ctrl Pts',(-2.102015121329,-1.,0.118079107988355));
#26937=CARTESIAN_POINT('Ctrl Pts',(-2.10777050261309,-1.,0.115544957687926));
#26938=CARTESIAN_POINT('Ctrl Pts',(-2.11351924490306,-1.,0.112968534419737));
#26939=CARTESIAN_POINT('Ctrl Pts',(-2.11926155590865,-1.,0.110350236135025));
#26940=CARTESIAN_POINT('Ctrl Pts',(-2.12499752307,-1.,0.10769043523109));
#26941=CARTESIAN_POINT('Ctrl Pts',(-2.13072704887293,-1.,0.104989479152739));
#26942=CARTESIAN_POINT('Ctrl Pts',(-2.13644992667165,-1.,0.1022477005561));
#26943=CARTESIAN_POINT('Ctrl Pts',(-2.14216588396025,-1.,0.0994654261990914));
#26944=CARTESIAN_POINT('Ctrl Pts',(-2.14787463531795,-1.,0.0966429852305457));
#26945=CARTESIAN_POINT('Ctrl Pts',(-2.1535759397817,-1.,0.0937807218867642));
#26946=CARTESIAN_POINT('Ctrl Pts',(-2.15926961544516,-1.,0.0908789888107264));
#26947=CARTESIAN_POINT('Ctrl Pts',(-2.16495552645014,-1.,0.0879381291386921));
#26948=CARTESIAN_POINT('Ctrl Pts',(-2.17063357870952,-1.,0.0849584620835371));
#26949=CARTESIAN_POINT('Ctrl Pts',(-2.176303712113,-1.,0.0819402680872764));
#26950=CARTESIAN_POINT('Ctrl Pts',(-2.18196589448887,-1.,0.0788837727685241));
#26951=CARTESIAN_POINT('Ctrl Pts',(-2.1876201139953,-1.,0.0757891465836146));
#26952=CARTESIAN_POINT('Ctrl Pts',(-2.19213712013662,-1.,0.0732830357306724));
#26953=CARTESIAN_POINT('Ctrl Pts',(-2.19552129484002,-1.,0.0713863779526153));
#26954=CARTESIAN_POINT('Ctrl Pts',(-2.19777582085423,-1.,0.0701143536325489));
#26955=CARTESIAN_POINT('Ctrl Pts',(-2.19890268624765,-1.,0.069476445021958));
#26956=CARTESIAN_POINT('',(-2.19890268624765,-1.,-0.0694764450219585));
#26957=CARTESIAN_POINT('',(-2.19890268624765,-1.,0.069476445021958));
#26958=CARTESIAN_POINT('',(-1.74236521665491,-1.,-0.163289472382896));
#26959=CARTESIAN_POINT('Ctrl Pts',(-2.19890268624765,-1.,-0.0694764450219585));
#26960=CARTESIAN_POINT('Ctrl Pts',(-2.19777582085261,-1.,-0.0701143536324927));
#26961=CARTESIAN_POINT('Ctrl Pts',(-2.19552129483562,-1.,-0.0713863779524629));
#26962=CARTESIAN_POINT('Ctrl Pts',(-2.19213712012956,-1.,-0.0732830357304277));
#26963=CARTESIAN_POINT('Ctrl Pts',(-2.1876201139874,-1.,-0.0757891465833413));
#26964=CARTESIAN_POINT('Ctrl Pts',(-2.18196589448304,-1.,-0.0788837727683229));
#26965=CARTESIAN_POINT('Ctrl Pts',(-2.1763037121106,-1.,-0.0819402680871941));
#26966=CARTESIAN_POINT('Ctrl Pts',(-2.17063357871031,-1.,-0.0849584620835644));
#26967=CARTESIAN_POINT('Ctrl Pts',(-2.16495552645275,-1.,-0.0879381291387824));
#26968=CARTESIAN_POINT('Ctrl Pts',(-2.15926961544808,-1.,-0.0908789888108267));
#26969=CARTESIAN_POINT('Ctrl Pts',(-2.15357593978377,-1.,-0.0937807218868346));
#26970=CARTESIAN_POINT('Ctrl Pts',(-2.14787463531864,-1.,-0.096642985230569));
#26971=CARTESIAN_POINT('Ctrl Pts',(-2.14216588395974,-1.,-0.0994654261990744));
#26972=CARTESIAN_POINT('Ctrl Pts',(-2.13644992667052,-1.,-0.102247700556064));
#26973=CARTESIAN_POINT('Ctrl Pts',(-2.1307270488718,-1.,-0.104989479152703));
#26974=CARTESIAN_POINT('Ctrl Pts',(-2.12499752306927,-1.,-0.107690435231068));
#26975=CARTESIAN_POINT('Ctrl Pts',(-2.11926155590849,-1.,-0.11035023613502));
#26976=CARTESIAN_POINT('Ctrl Pts',(-2.11351924490335,-1.,-0.112968534419746));
#26977=CARTESIAN_POINT('Ctrl Pts',(-2.10777050261359,-1.,-0.11554495768794));
#26978=CARTESIAN_POINT('Ctrl Pts',(-2.10201512132945,-1.,-0.118079107988368));
#26979=CARTESIAN_POINT('Ctrl Pts',(-2.09625292867756,-1.,-0.120570567965129));
#26980=CARTESIAN_POINT('Ctrl Pts',(-2.09048392424826,-1.,-0.123018905621083));
#26981=CARTESIAN_POINT('Ctrl Pts',(-2.08470840653628,-1.,-0.125423679412058));
#26982=CARTESIAN_POINT('Ctrl Pts',(-2.07892715110967,-1.,-0.127784445276116));
#26983=CARTESIAN_POINT('Ctrl Pts',(-2.07314114713047,-1.,-0.130100748328401));
#26984=CARTESIAN_POINT('Ctrl Pts',(-2.06735123910319,-1.,-0.13237211154771));
#26985=CARTESIAN_POINT('Ctrl Pts',(-2.06155781517844,-1.,-0.134598026192107));
#26986=CARTESIAN_POINT('Ctrl Pts',(-2.0557604441427,-1.,-0.136777941218044));
#26987=CARTESIAN_POINT('Ctrl Pts',(-2.04995762001333,-1.,-0.138911255368966));
#26988=CARTESIAN_POINT('Ctrl Pts',(-2.04414757947919,-1.,-0.140997332152545));
#26989=CARTESIAN_POINT('Ctrl Pts',(-2.03832911025913,-1.,-0.143035515058208));
#26990=CARTESIAN_POINT('Ctrl Pts',(-2.03250223739941,-1.,-0.145025140186058));
#26991=CARTESIAN_POINT('Ctrl Pts',(-2.02666926182017,-1.,-0.146965557332586));
#26992=CARTESIAN_POINT('Ctrl Pts',(-2.02083464969897,-1.,-0.148856124775343));
#26993=CARTESIAN_POINT('Ctrl Pts',(-2.01500291940243,-1.,-0.150696157673084));
#26994=CARTESIAN_POINT('Ctrl Pts',(-2.00917680318426,-1.,-0.152484883621452));
#26995=CARTESIAN_POINT('Ctrl Pts',(-2.00335565310539,-1.,-0.154221403049719));
#26996=CARTESIAN_POINT('Ctrl Pts',(-1.99753284771487,-1.,-0.155904629548775));
#26997=CARTESIAN_POINT('Ctrl Pts',(-1.99169810931893,-1.,-0.157533331459215));
#26998=CARTESIAN_POINT('Ctrl Pts',(-1.98584238283279,-1.,-0.159106226437289));
#26999=CARTESIAN_POINT('Ctrl Pts',(-1.97996195437557,-1.,-0.16062206078461));
#27000=CARTESIAN_POINT('Ctrl Pts',(-1.97406280235204,-1.,-0.162079693556302));
#27001=CARTESIAN_POINT('Ctrl Pts',(-1.96816512678,-1.,-0.16347818545776));
#27002=CARTESIAN_POINT('Ctrl Pts',(-1.96229379940174,-1.,-0.1648165689203));
#27003=CARTESIAN_POINT('Ctrl Pts',(-1.95646759718755,-1.,-0.166093592002833));
#27004=CARTESIAN_POINT('Ctrl Pts',(-1.95069027794286,-1.,-0.167307501784469));
#27005=CARTESIAN_POINT('Ctrl Pts',(-1.94493757756879,-1.,-0.168455741607516));
#27006=CARTESIAN_POINT('Ctrl Pts',(-1.93915639211497,-1.,-0.169534904817425));
#27007=CARTESIAN_POINT('Ctrl Pts',(-1.93329183155455,-1.,-0.170541253116136));
#27008=CARTESIAN_POINT('Ctrl Pts',(-1.92731093582,-1.,-0.17147119153296));
#27009=CARTESIAN_POINT('Ctrl Pts',(-1.92122334398034,-1.,-0.172321621259557));
#27010=CARTESIAN_POINT('Ctrl Pts',(-1.91511429159681,-1.,-0.173090695383619));
#27011=CARTESIAN_POINT('Ctrl Pts',(-1.90911693975475,-1.,-0.173776635257984));
#27012=CARTESIAN_POINT('Ctrl Pts',(-1.90335253863003,-1.,-0.174375518661222));
#27013=CARTESIAN_POINT('Ctrl Pts',(-1.89788101117148,-1.,-0.174879405091277));
#27014=CARTESIAN_POINT('Ctrl Pts',(-1.89264630198279,-1.,-0.175274276190664));
#27015=CARTESIAN_POINT('Ctrl Pts',(-1.88742606272818,-1.,-0.175538155840286));
#27016=CARTESIAN_POINT('Ctrl Pts',(-1.88188663144846,-1.,-0.175644148889271));
#27017=CARTESIAN_POINT('Ctrl Pts',(-1.87563767773249,-1.,-0.175563480746205));
#27018=CARTESIAN_POINT('Ctrl Pts',(-1.86828349694972,-1.,-0.175268337590901));
#27019=CARTESIAN_POINT('Ctrl Pts',(-1.85948367089838,-1.,-0.174735259276856));
#27020=CARTESIAN_POINT('Ctrl Pts',(-1.84898113200543,-1.,-0.173946627589401));
#27021=CARTESIAN_POINT('Ctrl Pts',(-1.83658380530747,-1.,-0.17288944289442));
#27022=CARTESIAN_POINT('Ctrl Pts',(-1.82215766815414,-1.,-0.171554770207306));
#27023=CARTESIAN_POINT('Ctrl Pts',(-1.80561530633924,-1.,-0.169936923908078));
#27024=CARTESIAN_POINT('Ctrl Pts',(-1.78690649988931,-1.,-0.16803277280837));
#27025=CARTESIAN_POINT('Ctrl Pts',(-1.77018771687692,-1.,-0.166279355148738));
#27026=CARTESIAN_POINT('Ctrl Pts',(-1.75666056640041,-1.,-0.164834765708484));
#27027=CARTESIAN_POINT('Ctrl Pts',(-1.74720349503904,-1.,-0.163814161002474));
#27028=CARTESIAN_POINT('Ctrl Pts',(-1.74236521665491,-1.,-0.163289472382896));
#27029=CARTESIAN_POINT('',(-1.7075470150345,-1.,-0.383122945602004));
#27030=CARTESIAN_POINT('Origin',(0.,-1.,0.));
#27031=CARTESIAN_POINT('',(-2.11275013067528,-1.,-0.61342227326009));
#27032=CARTESIAN_POINT('Ctrl Pts',(-1.7075470150345,-1.,-0.383122945602004));
#27033=CARTESIAN_POINT('Ctrl Pts',(-1.71231062891398,-1.,-0.384119047314215));
#27034=CARTESIAN_POINT('Ctrl Pts',(-1.72162022244582,-1.,-0.386070790323281));
#27035=CARTESIAN_POINT('Ctrl Pts',(-1.73493170972829,-1.,-0.388877023502615));
#27036=CARTESIAN_POINT('Ctrl Pts',(-1.75137405310193,-1.,-0.392375812285395));
#27037=CARTESIAN_POINT('Ctrl Pts',(-1.76975560043442,-1.,-0.396346196110688));
#27038=CARTESIAN_POINT('Ctrl Pts',(-1.78598826343754,-1.,-0.399919403774155));
#27039=CARTESIAN_POINT('Ctrl Pts',(-1.80012077173238,-1.,-0.403107976163396));
#27040=CARTESIAN_POINT('Ctrl Pts',(-1.81223801812013,-1.,-0.405933518407175));
#27041=CARTESIAN_POINT('Ctrl Pts',(-1.82247022677562,-1.,-0.408428948106227));
#27042=CARTESIAN_POINT('Ctrl Pts',(-1.83100408895047,-1.,-0.410641256301276));
#27043=CARTESIAN_POINT('Ctrl Pts',(-1.8380895347617,-1.,-0.412633125322945));
#27044=CARTESIAN_POINT('Ctrl Pts',(-1.84405757074218,-1.,-0.414487438255542));
#27045=CARTESIAN_POINT('Ctrl Pts',(-1.84929312930314,-1.,-0.416300022039885));
#27046=CARTESIAN_POINT('Ctrl Pts',(-1.8541763285645,-1.,-0.418164129144045));
#27047=CARTESIAN_POINT('Ctrl Pts',(-1.8590328109667,-1.,-0.420157287975583));
#27048=CARTESIAN_POINT('Ctrl Pts',(-1.86408083333863,-1.,-0.422327307417884));
#27049=CARTESIAN_POINT('Ctrl Pts',(-1.8693780394412,-1.,-0.424678177290876));
#27050=CARTESIAN_POINT('Ctrl Pts',(-1.87486989291333,-1.,-0.427183828518743));
#27051=CARTESIAN_POINT('Ctrl Pts',(-1.88044229001778,-1.,-0.429803062482217));
#27052=CARTESIAN_POINT('Ctrl Pts',(-1.88596913666828,-1.,-0.432493038548833));
#27053=CARTESIAN_POINT('Ctrl Pts',(-1.89136993975585,-1.,-0.43522566096358));
#27054=CARTESIAN_POINT('Ctrl Pts',(-1.89663648956549,-1.,-0.437995003948443));
#27055=CARTESIAN_POINT('Ctrl Pts',(-1.90180124389137,-1.,-0.44080783370416));
#27056=CARTESIAN_POINT('Ctrl Pts',(-1.90691756144906,-1.,-0.44367755684917));
#27057=CARTESIAN_POINT('Ctrl Pts',(-1.91203699981095,-1.,-0.446617343485651));
#27058=CARTESIAN_POINT('Ctrl Pts',(-1.91718342555717,-1.,-0.449632260106572));
#27059=CARTESIAN_POINT('Ctrl Pts',(-1.9223538064847,-1.,-0.452719478359356));
#27060=CARTESIAN_POINT('Ctrl Pts',(-1.92753067150461,-1.,-0.455872005174335));
#27061=CARTESIAN_POINT('Ctrl Pts',(-1.93269066517936,-1.,-0.459081234547931));
#27062=CARTESIAN_POINT('Ctrl Pts',(-1.93781486640834,-1.,-0.462340031009087));
#27063=CARTESIAN_POINT('Ctrl Pts',(-1.94289794196205,-1.,-0.465645462026064));
#27064=CARTESIAN_POINT('Ctrl Pts',(-1.94794381136524,-1.,-0.468997482913158));
#27065=CARTESIAN_POINT('Ctrl Pts',(-1.95296148278136,-1.,-0.472397672264079));
#27066=CARTESIAN_POINT('Ctrl Pts',(-1.95796111148175,-1.,-0.475848034683171));
#27067=CARTESIAN_POINT('Ctrl Pts',(-1.96294933055938,-1.,-0.479349583074846));
#27068=CARTESIAN_POINT('Ctrl Pts',(-1.96792703422358,-1.,-0.482901662120686));
#27069=CARTESIAN_POINT('Ctrl Pts',(-1.97289186263272,-1.,-0.486502692907661));
#27070=CARTESIAN_POINT('Ctrl Pts',(-1.97783973019229,-1.,-0.490150627860955));
#27071=CARTESIAN_POINT('Ctrl Pts',(-1.9827665876182,-1.,-0.493843476541492));
#27072=CARTESIAN_POINT('Ctrl Pts',(-1.98767044752929,-1.,-0.497579909545564));
#27073=CARTESIAN_POINT('Ctrl Pts',(-1.9925514912615,-1.,-0.501359287727129));
#27074=CARTESIAN_POINT('Ctrl Pts',(-1.99741107463567,-1.,-0.505181361323011));
#27075=CARTESIAN_POINT('Ctrl Pts',(-2.00225107134733,-1.,-0.509046069886152));
#27076=CARTESIAN_POINT('Ctrl Pts',(-2.00707309946955,-1.,-0.512953306961813));
#27077=CARTESIAN_POINT('Ctrl Pts',(-2.01187773939257,-1.,-0.516902681728733));
#27078=CARTESIAN_POINT('Ctrl Pts',(-2.01666477917305,-1.,-0.520893590399428));
#27079=CARTESIAN_POINT('Ctrl Pts',(-2.02143356304712,-1.,-0.524925318333518));
#27080=CARTESIAN_POINT('Ctrl Pts',(-2.02618329083289,-1.,-0.52899712724191));
#27081=CARTESIAN_POINT('Ctrl Pts',(-2.03091336214401,-1.,-0.533108355132905));
#27082=CARTESIAN_POINT('Ctrl Pts',(-2.03562362953993,-1.,-0.537258489833134));
#27083=CARTESIAN_POINT('Ctrl Pts',(-2.0403142269048,-1.,-0.54144712061552));
#27084=CARTESIAN_POINT('Ctrl Pts',(-2.0449854471456,-1.,-0.545673903817348));
#27085=CARTESIAN_POINT('Ctrl Pts',(-2.04963761077974,-1.,-0.549938525150342));
#27086=CARTESIAN_POINT('Ctrl Pts',(-2.05427091604482,-1.,-0.554240657464109));
#27087=CARTESIAN_POINT('Ctrl Pts',(-2.05888537756571,-1.,-0.558579940185467));
#27088=CARTESIAN_POINT('Ctrl Pts',(-2.06348090160697,-1.,-0.562955993082574));
#27089=CARTESIAN_POINT('Ctrl Pts',(-2.06805732997383,-1.,-0.567368421181229));
#27090=CARTESIAN_POINT('Ctrl Pts',(-2.07261449292757,-1.,-0.571816823242411));
#27091=CARTESIAN_POINT('Ctrl Pts',(-2.07715226767361,-1.,-0.576300797416274));
#27092=CARTESIAN_POINT('Ctrl Pts',(-2.08167059018138,-1.,-0.580819952107257));
#27093=CARTESIAN_POINT('Ctrl Pts',(-2.086169437277,-1.,-0.585373918990895));
#27094=CARTESIAN_POINT('Ctrl Pts',(-2.09064881812053,-1.,-0.589962365403189));
#27095=CARTESIAN_POINT('Ctrl Pts',(-2.09510876220501,-1.,-0.594585006052823));
#27096=CARTESIAN_POINT('Ctrl Pts',(-2.09954930865331,-1.,-0.599241616422144));
#27097=CARTESIAN_POINT('Ctrl Pts',(-2.10397049887709,-1.,-0.603932030738212));
#27098=CARTESIAN_POINT('Ctrl Pts',(-2.10749199615859,-1.,-0.607711315456826));
#27099=CARTESIAN_POINT('Ctrl Pts',(-2.11012443807661,-1.,-0.610560911691113));
#27100=CARTESIAN_POINT('Ctrl Pts',(-2.11187554260142,-1.,-0.61246736556225));
#27101=CARTESIAN_POINT('Ctrl Pts',(-2.11275013067528,-1.,-0.61342227326009));
#27102=CARTESIAN_POINT('',(-2.0698113262342,-1.,-0.745574324794401));
#27103=CARTESIAN_POINT('',(-2.11275013067528,-1.,-0.61342227326009));
#27104=CARTESIAN_POINT('',(-1.60662857109684,-1.,-0.693717979106306));
#27105=CARTESIAN_POINT('Ctrl Pts',(-2.0698113262342,-1.,-0.745574324794401));
#27106=CARTESIAN_POINT('Ctrl Pts',(-2.06854248895575,-1.,-0.74583279137781));
#27107=CARTESIAN_POINT('Ctrl Pts',(-2.06600523016401,-1.,-0.746345871542695));
#27108=CARTESIAN_POINT('Ctrl Pts',(-2.06220058927162,-1.,-0.747103932785504));
#27109=CARTESIAN_POINT('Ctrl Pts',(-2.05713023030263,-1.,-0.748091554181101));
#27110=CARTESIAN_POINT('Ctrl Pts',(-2.05079645591606,-1.,-0.749287468663053));
#27111=CARTESIAN_POINT('Ctrl Pts',(-2.04446689147754,-1.,-0.750444657874758));
#27112=CARTESIAN_POINT('Ctrl Pts',(-2.03814160092173,-1.,-0.751562963361383));
#27113=CARTESIAN_POINT('Ctrl Pts',(-2.03182068456467,-1.,-0.752642180488104));
#27114=CARTESIAN_POINT('Ctrl Pts',(-2.02550428623587,-1.,-0.753682061113765));
#27115=CARTESIAN_POINT('Ctrl Pts',(-2.01919259406003,-1.,-0.75468233072352));
#27116=CARTESIAN_POINT('Ctrl Pts',(-2.01288584328149,-1.,-0.7556427049581));
#27117=CARTESIAN_POINT('Ctrl Pts',(-2.00658431587682,-1.,-0.756562904646496));
#27118=CARTESIAN_POINT('Ctrl Pts',(-2.00028834739072,-1.,-0.757442676862341));
#27119=CARTESIAN_POINT('Ctrl Pts',(-1.9939983109871,-1.,-0.758281796766377));
#27120=CARTESIAN_POINT('Ctrl Pts',(-1.98771456680806,-1.,-0.759080037802242));
#27121=CARTESIAN_POINT('Ctrl Pts',(-1.98143741418156,-1.,-0.759837147452135));
#27122=CARTESIAN_POINT('Ctrl Pts',(-1.97516705321521,-1.,-0.760552825409855));
#27123=CARTESIAN_POINT('Ctrl Pts',(-1.96890351582545,-1.,-0.761226690483986));
#27124=CARTESIAN_POINT('Ctrl Pts',(-1.96264672744229,-1.,-0.761858300014575));
#27125=CARTESIAN_POINT('Ctrl Pts',(-1.95639665309893,-1.,-0.762447203806263));
#27126=CARTESIAN_POINT('Ctrl Pts',(-1.95015342590025,-1.,-0.762992990878774));
#27127=CARTESIAN_POINT('Ctrl Pts',(-1.94391746617626,-1.,-0.76349533353858));
#27128=CARTESIAN_POINT('Ctrl Pts',(-1.93768964875867,-1.,-0.763954049121393));
#27129=CARTESIAN_POINT('Ctrl Pts',(-1.93147105496367,-1.,-0.764369010673889));
#27130=CARTESIAN_POINT('Ctrl Pts',(-1.92526263537041,-1.,-0.764740025488189));
#27131=CARTESIAN_POINT('Ctrl Pts',(-1.91906491634197,-1.,-0.765066729667095));
#27132=CARTESIAN_POINT('Ctrl Pts',(-1.91287765805174,-1.,-0.765348465884739));
#27133=CARTESIAN_POINT('Ctrl Pts',(-1.90669961402362,-1.,-0.765584196937936));
#27134=CARTESIAN_POINT('Ctrl Pts',(-1.90052930393599,-1.,-0.765772772593395));
#27135=CARTESIAN_POINT('Ctrl Pts',(-1.89436577771389,-1.,-0.765913193856979));
#27136=CARTESIAN_POINT('Ctrl Pts',(-1.88820926433409,-1.,-0.76600483706209));
#27137=CARTESIAN_POINT('Ctrl Pts',(-1.88206215302561,-1.,-0.766047794851868));
#27138=CARTESIAN_POINT('Ctrl Pts',(-1.87592888967886,-1.,-0.766042837036759));
#27139=CARTESIAN_POINT('Ctrl Pts',(-1.86981398314345,-1.,-0.765990708546111));
#27140=CARTESIAN_POINT('Ctrl Pts',(-1.86372027063314,-1.,-0.765891519092557));
#27141=CARTESIAN_POINT('Ctrl Pts',(-1.85764741390391,-1.,-0.765744212909305));
#27142=CARTESIAN_POINT('Ctrl Pts',(-1.85158945130054,-1.,-0.765545710619023));
#27143=CARTESIAN_POINT('Ctrl Pts',(-1.8455369887591,-1.,-0.765291664861971));
#27144=CARTESIAN_POINT('Ctrl Pts',(-1.83948181064823,-1.,-0.764978057881687));
#27145=CARTESIAN_POINT('Ctrl Pts',(-1.8334207722714,-1.,-0.764602549687845));
#27146=CARTESIAN_POINT('Ctrl Pts',(-1.8273599120008,-1.,-0.764165902606055));
#27147=CARTESIAN_POINT('Ctrl Pts',(-1.82131873145297,-1.,-0.763673465462854));
#27148=CARTESIAN_POINT('Ctrl Pts',(-1.81532118405566,-1.,-0.763132003836783));
#27149=CARTESIAN_POINT('Ctrl Pts',(-1.80938551463989,-1.,-0.762546129464036));
#27150=CARTESIAN_POINT('Ctrl Pts',(-1.80351583877334,-1.,-0.761915336443515));
#27151=CARTESIAN_POINT('Ctrl Pts',(-1.79768986997735,-1.,-0.761229695230359));
#27152=CARTESIAN_POINT('Ctrl Pts',(-1.79185815610802,-1.,-0.760469555880425));
#27153=CARTESIAN_POINT('Ctrl Pts',(-1.78596964884526,-1.,-0.759614401109868));
#27154=CARTESIAN_POINT('Ctrl Pts',(-1.77999411220912,-1.,-0.75865062667738));
#27155=CARTESIAN_POINT('Ctrl Pts',(-1.77394167108342,-1.,-0.757578264077238));
#27156=CARTESIAN_POINT('Ctrl Pts',(-1.76789396003141,-1.,-0.756421896028403));
#27157=CARTESIAN_POINT('Ctrl Pts',(-1.7619781724032,-1.,-0.755220979975262));
#27158=CARTESIAN_POINT('Ctrl Pts',(-1.75631083600175,-1.,-0.75400925402848));
#27159=CARTESIAN_POINT('Ctrl Pts',(-1.75095139468809,-1.,-0.752797683531377));
#27160=CARTESIAN_POINT('Ctrl Pts',(-1.74585086852298,-1.,-0.751555614163629));
#27161=CARTESIAN_POINT('Ctrl Pts',(-1.74080458266705,-1.,-0.75019343597954));
#27162=CARTESIAN_POINT('Ctrl Pts',(-1.73550351679848,-1.,-0.748582462954854));
#27163=CARTESIAN_POINT('Ctrl Pts',(-1.72958533647399,-1.,-0.746574710096436));
#27164=CARTESIAN_POINT('Ctrl Pts',(-1.7226822991693,-1.,-0.744021445433764));
#27165=CARTESIAN_POINT('Ctrl Pts',(-1.71447789751927,-1.,-0.740795162032087));
#27166=CARTESIAN_POINT('Ctrl Pts',(-1.70473309006121,-1.,-0.736799665724771));
#27167=CARTESIAN_POINT('Ctrl Pts',(-1.69326921975743,-1.,-0.731963238697195));
#27168=CARTESIAN_POINT('Ctrl Pts',(-1.67996158455503,-1.,-0.726235967997433));
#27169=CARTESIAN_POINT('Ctrl Pts',(-1.6647288055568,-1.,-0.719585433804282));
#27170=CARTESIAN_POINT('Ctrl Pts',(-1.64752408832016,-1.,-0.711993139355394));
#27171=CARTESIAN_POINT('Ctrl Pts',(-1.63216541664676,-1.,-0.705159151988319));
#27172=CARTESIAN_POINT('Ctrl Pts',(-1.61974673472612,-1.,-0.699605146405088));
#27173=CARTESIAN_POINT('Ctrl Pts',(-1.61106790958151,-1.,-0.695712097881194));
#27174=CARTESIAN_POINT('Ctrl Pts',(-1.60662857109684,-1.,-0.693717979106306));
#27175=CARTESIAN_POINT('',(-1.5055822144029,-1.,-0.892032620296855));
#27176=CARTESIAN_POINT('Origin',(0.,-1.,0.));
#27177=CARTESIAN_POINT('',(-1.81978687191668,-1.,-1.23627494547115));
#27178=CARTESIAN_POINT('Ctrl Pts',(-1.5055822144029,-1.,-0.892032620296855));
#27179=CARTESIAN_POINT('Ctrl Pts',(-1.50980486806688,-1.,-0.894452006964543));
#27180=CARTESIAN_POINT('Ctrl Pts',(-1.51805569590094,-1.,-0.899185047483511));
#27181=CARTESIAN_POINT('Ctrl Pts',(-1.52984849887993,-1.,-0.905967409625651));
#27182=CARTESIAN_POINT('Ctrl Pts',(-1.54440491149498,-1.,-0.914375919026456));
#27183=CARTESIAN_POINT('Ctrl Pts',(-1.56065988578893,-1.,-0.923832188944341));
#27184=CARTESIAN_POINT('Ctrl Pts',(-1.57499388382243,-1.,-0.932246680108685));
#27185=CARTESIAN_POINT('Ctrl Pts',(-1.58744937487176,-1.,-0.939646377893399));
#27186=CARTESIAN_POINT('Ctrl Pts',(-1.59810042043673,-1.,-0.946078063315257));
#27187=CARTESIAN_POINT('Ctrl Pts',(-1.60706069896936,-1.,-0.951613284356035));
#27188=CARTESIAN_POINT('Ctrl Pts',(-1.61449324337085,-1.,-0.956354422920671));
#27189=CARTESIAN_POINT('Ctrl Pts',(-1.62061638140221,-1.,-0.960438326101729));
#27190=CARTESIAN_POINT('Ctrl Pts',(-1.62571930670187,-1.,-0.964046107040536));
#27191=CARTESIAN_POINT('Ctrl Pts',(-1.63013849959461,-1.,-0.967387853230345));
#27192=CARTESIAN_POINT('Ctrl Pts',(-1.63420665729798,-1.,-0.970669715997509));
#27193=CARTESIAN_POINT('Ctrl Pts',(-1.63820952658144,-1.,-0.974066058287418));
#27194=CARTESIAN_POINT('Ctrl Pts',(-1.64233990826687,-1.,-0.977689794119416));
#27195=CARTESIAN_POINT('Ctrl Pts',(-1.64665139190656,-1.,-0.981562530939489));
#27196=CARTESIAN_POINT('Ctrl Pts',(-1.65110016612638,-1.,-0.985642622920821));
#27197=CARTESIAN_POINT('Ctrl Pts',(-1.65559044289699,-1.,-0.989855627854165));
#27198=CARTESIAN_POINT('Ctrl Pts',(-1.66001553809947,-1.,-0.994121836661306));
#27199=CARTESIAN_POINT('Ctrl Pts',(-1.66430758030376,-1.,-0.998389654952758));
#27200=CARTESIAN_POINT('Ctrl Pts',(-1.66846059277303,-1.,-1.00265091003727));
#27201=CARTESIAN_POINT('Ctrl Pts',(-1.67250335383293,-1.,-1.00692206696414));
#27202=CARTESIAN_POINT('Ctrl Pts',(-1.67648246776464,-1.,-1.01123236493511));
#27203=CARTESIAN_POINT('Ctrl Pts',(-1.68044289894798,-1.,-1.01561026162773));
#27204=CARTESIAN_POINT('Ctrl Pts',(-1.68440578021706,-1.,-1.02006795074201));
#27205=CARTESIAN_POINT('Ctrl Pts',(-1.68836910178447,-1.,-1.02460180535255));
#27206=CARTESIAN_POINT('Ctrl Pts',(-1.69231840863458,-1.,-1.02919977579147));
#27207=CARTESIAN_POINT('Ctrl Pts',(-1.69623414782771,-1.,-1.03384646003588));
#27208=CARTESIAN_POINT('Ctrl Pts',(-1.70010052930962,-1.,-1.03852922490789));
#27209=CARTESIAN_POINT('Ctrl Pts',(-1.70391338707982,-1.,-1.04324363334554));
#27210=CARTESIAN_POINT('Ctrl Pts',(-1.70767646263649,-1.,-1.04799085404995));
#27211=CARTESIAN_POINT('Ctrl Pts',(-1.71139783543989,-1.,-1.05277517202855));
#27212=CARTESIAN_POINT('Ctrl Pts',(-1.7150865442702,-1.,-1.05760163192479));
#27213=CARTESIAN_POINT('Ctrl Pts',(-1.71874858456904,-1.,-1.06247324680647));
#27214=CARTESIAN_POINT('Ctrl Pts',(-1.72238500928453,-1.,-1.06738966975462));
#27215=CARTESIAN_POINT('Ctrl Pts',(-1.72599406198488,-1.,-1.07234866990252));
#27216=CARTESIAN_POINT('Ctrl Pts',(-1.72957248977424,-1.,-1.0773470373727));
#27217=CARTESIAN_POINT('Ctrl Pts',(-1.73311705663407,-1.,-1.08238162784749));
#27218=CARTESIAN_POINT('Ctrl Pts',(-1.73662628326091,-1.,-1.08745056285427));
#27219=CARTESIAN_POINT('Ctrl Pts',(-1.74010053962247,-1.,-1.09255329056493));
#27220=CARTESIAN_POINT('Ctrl Pts',(-1.74354119236208,-1.,-1.09768999241225));
#27221=CARTESIAN_POINT('Ctrl Pts',(-1.74695004214923,-1.,-1.10286118991143));
#27222=CARTESIAN_POINT('Ctrl Pts',(-1.7503286607592,-1.,-1.10806728183007));
#27223=CARTESIAN_POINT('Ctrl Pts',(-1.7536777209463,-1.,-1.11330807582551));
#27224=CARTESIAN_POINT('Ctrl Pts',(-1.75699720772105,-1.,-1.11858293216763));
#27225=CARTESIAN_POINT('Ctrl Pts',(-1.76028671825096,-1.,-1.12389096855086));
#27226=CARTESIAN_POINT('Ctrl Pts',(-1.7635457196617,-1.,-1.12923123555075));
#27227=CARTESIAN_POINT('Ctrl Pts',(-1.76677384551862,-1.,-1.1346029180462));
#27228=CARTESIAN_POINT('Ctrl Pts',(-1.76997111386769,-1.,-1.14000548336975));
#27229=CARTESIAN_POINT('Ctrl Pts',(-1.77313777896194,-1.,-1.1454385822692));
#27230=CARTESIAN_POINT('Ctrl Pts',(-1.7762742255701,-1.,-1.15090197841515));
#27231=CARTESIAN_POINT('Ctrl Pts',(-1.77938085564275,-1.,-1.15639547194698));
#27232=CARTESIAN_POINT('Ctrl Pts',(-1.78245795881009,-1.,-1.16191881298499));
#27233=CARTESIAN_POINT('Ctrl Pts',(-1.78550566040443,-1.,-1.16747166312303));
#27234=CARTESIAN_POINT('Ctrl Pts',(-1.78852398877616,-1.,-1.17305363177328));
#27235=CARTESIAN_POINT('Ctrl Pts',(-1.79151291552689,-1.,-1.17866429440809));
#27236=CARTESIAN_POINT('Ctrl Pts',(-1.79447240321515,-1.,-1.18430321697432));
#27237=CARTESIAN_POINT('Ctrl Pts',(-1.79740245923478,-1.,-1.18996997934445));
#27238=CARTESIAN_POINT('Ctrl Pts',(-1.80030314369879,-1.,-1.19566418930242));
#27239=CARTESIAN_POINT('Ctrl Pts',(-1.80317454838603,-1.,-1.20138548938974));
#27240=CARTESIAN_POINT('Ctrl Pts',(-1.80601678480707,-1.,-1.20713356605475));
#27241=CARTESIAN_POINT('Ctrl Pts',(-1.80882996917129,-1.,-1.21290815708314));
#27242=CARTESIAN_POINT('Ctrl Pts',(-1.81161420806656,-1.,-1.21870906103557));
#27243=CARTESIAN_POINT('Ctrl Pts',(-1.81436959210434,-1.,-1.2245361330495));
#27244=CARTESIAN_POINT('Ctrl Pts',(-1.8165508718364,-1.,-1.2292186489137));
#27245=CARTESIAN_POINT('Ctrl Pts',(-1.81817389921279,-1.,-1.2327422452705));
#27246=CARTESIAN_POINT('Ctrl Pts',(-1.81925017193666,-1.,-1.23509651170476));
#27247=CARTESIAN_POINT('Ctrl Pts',(-1.81978687191668,-1.,-1.23627494547115));
#27248=CARTESIAN_POINT('',(-1.73811241238545,-1.,-1.34869019493419));
#27249=CARTESIAN_POINT('',(-1.81978687191668,-1.,-1.23627494547115));
#27250=CARTESIAN_POINT('',(-1.31362392696032,-1.,-1.15624053661742));
#27251=CARTESIAN_POINT('Ctrl Pts',(-1.73811241238545,-1.,-1.34869019493419));
#27252=CARTESIAN_POINT('Ctrl Pts',(-1.73682580585691,-1.,-1.34854391898045));
#27253=CARTESIAN_POINT('Ctrl Pts',(-1.73425417885907,-1.,-1.34824783112887));
#27254=CARTESIAN_POINT('Ctrl Pts',(-1.7304014965394,-1.,-1.34779309152035));
#27255=CARTESIAN_POINT('Ctrl Pts',(-1.72527410680674,-1.,-1.34716554819527));
#27256=CARTESIAN_POINT('Ctrl Pts',(-1.7188807715049,-1.,-1.34634568653227));
#27257=CARTESIAN_POINT('Ctrl Pts',(-1.71250340686822,-1.,-1.34549029589416));
#27258=CARTESIAN_POINT('Ctrl Pts',(-1.70614212266738,-1.,-1.34459924533831));
#27259=CARTESIAN_POINT('Ctrl Pts',(-1.69979707754427,-1.,-1.34367237124483));
#27260=CARTESIAN_POINT('Ctrl Pts',(-1.6934684849687,-1.,-1.34270948206319));
#27261=CARTESIAN_POINT('Ctrl Pts',(-1.68715660868764,-1.,-1.341710374848));
#27262=CARTESIAN_POINT('Ctrl Pts',(-1.68086176030362,-1.,-1.34067485185203));
#27263=CARTESIAN_POINT('Ctrl Pts',(-1.67458429426086,-1.,-1.3396027347034));
#27264=CARTESIAN_POINT('Ctrl Pts',(-1.66832460783989,-1.,-1.33849388654388));
#27265=CARTESIAN_POINT('Ctrl Pts',(-1.66208312541983,-1.,-1.33734820885262));
#27266=CARTESIAN_POINT('Ctrl Pts',(-1.65586025952593,-1.,-1.33616559745172));
#27267=CARTESIAN_POINT('Ctrl Pts',(-1.6496563728683,-1.,-1.33494590467993));
#27268=CARTESIAN_POINT('Ctrl Pts',(-1.6434717485603,-1.,-1.33368890676572));
#27269=CARTESIAN_POINT('Ctrl Pts',(-1.63730653475089,-1.,-1.33239425103724));
#27270=CARTESIAN_POINT('Ctrl Pts',(-1.63116079730923,-1.,-1.33106149345645));
#27271=CARTESIAN_POINT('Ctrl Pts',(-1.62503464209797,-1.,-1.3296901950568));
#27272=CARTESIAN_POINT('Ctrl Pts',(-1.61892832270724,-1.,-1.32828000610449));
#27273=CARTESIAN_POINT('Ctrl Pts',(-1.6128423401575,-1.,-1.32683074483356));
#27274=CARTESIAN_POINT('Ctrl Pts',(-1.60677758290954,-1.,-1.32534250785782));
#27275=CARTESIAN_POINT('Ctrl Pts',(-1.60073511858687,-1.,-1.32381550858256));
#27276=CARTESIAN_POINT('Ctrl Pts',(-1.59471591079403,-1.,-1.32224985747682));
#27277=CARTESIAN_POINT('Ctrl Pts',(-1.58872057258245,-1.,-1.32064537110892));
#27278=CARTESIAN_POINT('Ctrl Pts',(-1.58274907898834,-1.,-1.31900135021432));
#27279=CARTESIAN_POINT('Ctrl Pts',(-1.5768005650559,-1.,-1.31731642317187));
#27280=CARTESIAN_POINT('Ctrl Pts',(-1.57087397835723,-1.,-1.31558903860016));
#27281=CARTESIAN_POINT('Ctrl Pts',(-1.56496872402353,-1.,-1.31381795281002));
#27282=CARTESIAN_POINT('Ctrl Pts',(-1.55908521254821,-1.,-1.31200264341696));
#27283=CARTESIAN_POINT('Ctrl Pts',(-1.55322568759481,-1.,-1.31014393684222));
#27284=CARTESIAN_POINT('Ctrl Pts',(-1.54739413957185,-1.,-1.30824393907473));
#27285=CARTESIAN_POINT('Ctrl Pts',(-1.54159462645432,-1.,-1.30630475189556));
#27286=CARTESIAN_POINT('Ctrl Pts',(-1.53582981268977,-1.,-1.30432735639489));
#27287=CARTESIAN_POINT('Ctrl Pts',(-1.53009970283891,-1.,-1.30231064395568));
#27288=CARTESIAN_POINT('Ctrl Pts',(-1.52439957861062,-1.,-1.30024984366328));
#27289=CARTESIAN_POINT('Ctrl Pts',(-1.51872184912724,-1.,-1.29813791800747));
#27290=CARTESIAN_POINT('Ctrl Pts',(-1.51305994241402,-1.,-1.29596850710509));
#27291=CARTESIAN_POINT('Ctrl Pts',(-1.50741159078365,-1.,-1.29373841372842));
#27292=CARTESIAN_POINT('Ctrl Pts',(-1.50178230149776,-1.,-1.29145022885181));
#27293=CARTESIAN_POINT('Ctrl Pts',(-1.49618896881754,-1.,-1.28911506584254));
#27294=CARTESIAN_POINT('Ctrl Pts',(-1.4906522831278,-1.,-1.2867467611644));
#27295=CARTESIAN_POINT('Ctrl Pts',(-1.4851881711891,-1.,-1.28435533880201));
#27296=CARTESIAN_POINT('Ctrl Pts',(-1.47980070347095,-1.,-1.28194158939517));
#27297=CARTESIAN_POINT('Ctrl Pts',(-1.4744717526707,-1.,-1.2794891824849));
#27298=CARTESIAN_POINT('Ctrl Pts',(-1.46916035917133,-1.,-1.27696414831089));
#27299=CARTESIAN_POINT('Ctrl Pts',(-1.46382431332476,-1.,-1.27433119897822));
#27300=CARTESIAN_POINT('Ctrl Pts',(-1.45843906294697,-1.,-1.27156805265289));
#27301=CARTESIAN_POINT('Ctrl Pts',(-1.45301422764247,-1.,-1.2686778680489));
#27302=CARTESIAN_POINT('Ctrl Pts',(-1.44761985001662,-1.,-1.26570925118868));
#27303=CARTESIAN_POINT('Ctrl Pts',(-1.44236470511303,-1.,-1.26273903323859));
#27304=CARTESIAN_POINT('Ctrl Pts',(-1.43734919180848,-1.,-1.25983531012005));
#27305=CARTESIAN_POINT('Ctrl Pts',(-1.43262645609691,-1.,-1.25702687965755));
#27306=CARTESIAN_POINT('Ctrl Pts',(-1.42815938799387,-1.,-1.25426945222639));
#27307=CARTESIAN_POINT('Ctrl Pts',(-1.42378102115575,-1.,-1.2514145557001));
#27308=CARTESIAN_POINT('Ctrl Pts',(-1.41923722596025,-1.,-1.24824430986571));
#27309=CARTESIAN_POINT('Ctrl Pts',(-1.41422913175179,-1.,-1.24450600513056));
#27310=CARTESIAN_POINT('Ctrl Pts',(-1.40845295531283,-1.,-1.23994455029534));
#27311=CARTESIAN_POINT('Ctrl Pts',(-1.40164708206106,-1.,-1.23434087290423));
#27312=CARTESIAN_POINT('Ctrl Pts',(-1.39361389568796,-1.,-1.22752961899387));
#27313=CARTESIAN_POINT('Ctrl Pts',(-1.38420564527715,-1.,-1.21938737280852));
#27314=CARTESIAN_POINT('Ctrl Pts',(-1.37331915607905,-1.,-1.20982812925645));
#27315=CARTESIAN_POINT('Ctrl Pts',(-1.36088705043885,-1.,-1.1987959077932));
#27316=CARTESIAN_POINT('Ctrl Pts',(-1.34687054001093,-1.,-1.18625865667441));
#27317=CARTESIAN_POINT('Ctrl Pts',(-1.33437539347008,-1.,-1.17501305789857));
#27318=CARTESIAN_POINT('Ctrl Pts',(-1.32428080721772,-1.,-1.16589330093588));
#27319=CARTESIAN_POINT('Ctrl Pts',(-1.31722977216397,-1.,-1.15950888730809));
#27320=CARTESIAN_POINT('Ctrl Pts',(-1.31362392696032,-1.,-1.15624053661742));
#27321=CARTESIAN_POINT('',(-1.15624053661742,-1.,-1.31362392696033));
#27322=CARTESIAN_POINT('Origin',(0.,-1.,0.));
#27323=CARTESIAN_POINT('',(-1.34869019493419,-1.,-1.73811241238545));
#27324=CARTESIAN_POINT('Ctrl Pts',(-1.15624053661742,-1.,-1.31362392696033));
#27325=CARTESIAN_POINT('Ctrl Pts',(-1.15950888730433,-1.,-1.3172297721596));
#27326=CARTESIAN_POINT('Ctrl Pts',(-1.16589330092532,-1.,-1.32428080720544));
#27327=CARTESIAN_POINT('Ctrl Pts',(-1.17501305787994,-1.,-1.33437539344842));
#27328=CARTESIAN_POINT('Ctrl Pts',(-1.18625865664915,-1.,-1.34687053998157));
#27329=CARTESIAN_POINT('Ctrl Pts',(-1.1987959077656,-1.,-1.36088705040677));
#27330=CARTESIAN_POINT('Ctrl Pts',(-1.20982812923113,-1.,-1.37331915604962));
#27331=CARTESIAN_POINT('Ctrl Pts',(-1.21938737278853,-1.,-1.38420564525391));
#27332=CARTESIAN_POINT('Ctrl Pts',(-1.22752961898063,-1.,-1.39361389567257));
#27333=CARTESIAN_POINT('Ctrl Pts',(-1.23434087289768,-1.,-1.40164708205345));
#27334=CARTESIAN_POINT('Ctrl Pts',(-1.23994455029421,-1.,-1.40845295531151));
#27335=CARTESIAN_POINT('Ctrl Pts',(-1.24450600513278,-1.,-1.41422913175437));
#27336=CARTESIAN_POINT('Ctrl Pts',(-1.24824430986911,-1.,-1.41923722596421));
#27337=CARTESIAN_POINT('Ctrl Pts',(-1.25141455570299,-1.,-1.42378102115911));
#27338=CARTESIAN_POINT('Ctrl Pts',(-1.25426945222783,-1.,-1.42815938799555));
#27339=CARTESIAN_POINT('Ctrl Pts',(-1.25702687965744,-1.,-1.43262645609679));
#27340=CARTESIAN_POINT('Ctrl Pts',(-1.25983531011894,-1.,-1.43734919180719));
#27341=CARTESIAN_POINT('Ctrl Pts',(-1.26273903323723,-1.,-1.44236470511145));
#27342=CARTESIAN_POINT('Ctrl Pts',(-1.26570925118767,-1.,-1.44761985001544));
#27343=CARTESIAN_POINT('Ctrl Pts',(-1.26867786804854,-1.,-1.45301422764205));
#27344=CARTESIAN_POINT('Ctrl Pts',(-1.27156805265312,-1.,-1.45843906294725));
#27345=CARTESIAN_POINT('Ctrl Pts',(-1.27433119897877,-1.,-1.4638243133254));
#27346=CARTESIAN_POINT('Ctrl Pts',(-1.27696414831144,-1.,-1.46916035917197));
#27347=CARTESIAN_POINT('Ctrl Pts',(-1.27948918248524,-1.,-1.4744717526711));
#27348=CARTESIAN_POINT('Ctrl Pts',(-1.28194158939522,-1.,-1.47980070347102));
#27349=CARTESIAN_POINT('Ctrl Pts',(-1.28435533880184,-1.,-1.48518817118891));
#27350=CARTESIAN_POINT('Ctrl Pts',(-1.28674676116415,-1.,-1.4906522831275));
#27351=CARTESIAN_POINT('Ctrl Pts',(-1.28911506584232,-1.,-1.49618896881729));
#27352=CARTESIAN_POINT('Ctrl Pts',(-1.29145022885171,-1.,-1.50178230149764));
#27353=CARTESIAN_POINT('Ctrl Pts',(-1.29373841372843,-1.,-1.50741159078367));
#27354=CARTESIAN_POINT('Ctrl Pts',(-1.29596850710518,-1.,-1.51305994241412));
#27355=CARTESIAN_POINT('Ctrl Pts',(-1.29813791800757,-1.,-1.51872184912735));
#27356=CARTESIAN_POINT('Ctrl Pts',(-1.30024984366334,-1.,-1.5243995786107));
#27357=CARTESIAN_POINT('Ctrl Pts',(-1.3023106439557,-1.,-1.53009970283893));
#27358=CARTESIAN_POINT('Ctrl Pts',(-1.30432735639487,-1.,-1.53582981268976));
#27359=CARTESIAN_POINT('Ctrl Pts',(-1.30630475189553,-1.,-1.54159462645428));
#27360=CARTESIAN_POINT('Ctrl Pts',(-1.30824393907471,-1.,-1.54739413957183));
#27361=CARTESIAN_POINT('Ctrl Pts',(-1.31014393684221,-1.,-1.55322568759481));
#27362=CARTESIAN_POINT('Ctrl Pts',(-1.31200264341696,-1.,-1.55908521254822));
#27363=CARTESIAN_POINT('Ctrl Pts',(-1.31381795281002,-1.,-1.56496872402352));
#27364=CARTESIAN_POINT('Ctrl Pts',(-1.31558903860015,-1.,-1.57087397835721));
#27365=CARTESIAN_POINT('Ctrl Pts',(-1.31731642317183,-1.,-1.57680056505585));
#27366=CARTESIAN_POINT('Ctrl Pts',(-1.31900135021428,-1.,-1.58274907898829));
#27367=CARTESIAN_POINT('Ctrl Pts',(-1.32064537110891,-1.,-1.58872057258244));
#27368=CARTESIAN_POINT('Ctrl Pts',(-1.32224985747686,-1.,-1.59471591079408));
#27369=CARTESIAN_POINT('Ctrl Pts',(-1.32381550858266,-1.,-1.600735118587));
#27370=CARTESIAN_POINT('Ctrl Pts',(-1.32534250785794,-1.,-1.6067775829097));
#27371=CARTESIAN_POINT('Ctrl Pts',(-1.32683074483365,-1.,-1.61284234015762));
#27372=CARTESIAN_POINT('Ctrl Pts',(-1.32828000610448,-1.,-1.61892832270723));
#27373=CARTESIAN_POINT('Ctrl Pts',(-1.32969019505665,-1.,-1.62503464209777));
#27374=CARTESIAN_POINT('Ctrl Pts',(-1.33106149345618,-1.,-1.63116079730887));
#27375=CARTESIAN_POINT('Ctrl Pts',(-1.33239425103694,-1.,-1.6373065347505));
#27376=CARTESIAN_POINT('Ctrl Pts',(-1.33368890676554,-1.,-1.64347174856007));
#27377=CARTESIAN_POINT('Ctrl Pts',(-1.33494590468003,-1.,-1.64965637286843));
#27378=CARTESIAN_POINT('Ctrl Pts',(-1.33616559745217,-1.,-1.65586025952651));
#27379=CARTESIAN_POINT('Ctrl Pts',(-1.33734820885331,-1.,-1.66208312542073));
#27380=CARTESIAN_POINT('Ctrl Pts',(-1.33849388654458,-1.,-1.66832460784078));
#27381=CARTESIAN_POINT('Ctrl Pts',(-1.33960273470372,-1.,-1.67458429426126));
#27382=CARTESIAN_POINT('Ctrl Pts',(-1.3406748518516,-1.,-1.68086176030308));
#27383=CARTESIAN_POINT('Ctrl Pts',(-1.34171037484673,-1.,-1.68715660868602));
#27384=CARTESIAN_POINT('Ctrl Pts',(-1.34270948206139,-1.,-1.6934684849664));
#27385=CARTESIAN_POINT('Ctrl Pts',(-1.34367237124322,-1.,-1.69979707754221));
#27386=CARTESIAN_POINT('Ctrl Pts',(-1.34459924533783,-1.,-1.70614212266676));
#27387=CARTESIAN_POINT('Ctrl Pts',(-1.34549029589563,-1.,-1.71250340687011));
#27388=CARTESIAN_POINT('Ctrl Pts',(-1.34634568653586,-1.,-1.7188807715095));
#27389=CARTESIAN_POINT('Ctrl Pts',(-1.34716554820013,-1.,-1.72527410681298));
#27390=CARTESIAN_POINT('Ctrl Pts',(-1.3477930915247,-1.,-1.73040149654497));
#27391=CARTESIAN_POINT('Ctrl Pts',(-1.34824783113158,-1.,-1.73425417886255));
#27392=CARTESIAN_POINT('Ctrl Pts',(-1.34854391898145,-1.,-1.73682580585819));
#27393=CARTESIAN_POINT('Ctrl Pts',(-1.34869019493419,-1.,-1.73811241238545));
#27394=CARTESIAN_POINT('',(-1.23627494547115,-1.,-1.81978687191668));
#27395=CARTESIAN_POINT('',(-1.34869019493419,-1.,-1.73811241238545));
#27396=CARTESIAN_POINT('',(-0.892032620296855,-1.,-1.5055822144029));
#27397=CARTESIAN_POINT('Ctrl Pts',(-1.23627494547115,-1.,-1.81978687191668));
#27398=CARTESIAN_POINT('Ctrl Pts',(-1.23509651170384,-1.,-1.81925017193531));
#27399=CARTESIAN_POINT('Ctrl Pts',(-1.23274224526804,-1.,-1.81817389920914));
#27400=CARTESIAN_POINT('Ctrl Pts',(-1.22921864890975,-1.,-1.81655087183054));
#27401=CARTESIAN_POINT('Ctrl Pts',(-1.22453613304507,-1.,-1.81436959209778));
#27402=CARTESIAN_POINT('Ctrl Pts',(-1.2187090610323,-1.,-1.81161420806172));
#27403=CARTESIAN_POINT('Ctrl Pts',(-1.2129081570818,-1.,-1.80882996916931));
#27404=CARTESIAN_POINT('Ctrl Pts',(-1.20713356605519,-1.,-1.80601678480772));
#27405=CARTESIAN_POINT('Ctrl Pts',(-1.2013854893912,-1.,-1.8031745483882));
#27406=CARTESIAN_POINT('Ctrl Pts',(-1.19566418930405,-1.,-1.80030314370121));
#27407=CARTESIAN_POINT('Ctrl Pts',(-1.1899699793456,-1.,-1.79740245923649));
#27408=CARTESIAN_POINT('Ctrl Pts',(-1.18430321697471,-1.,-1.79447240321572));
#27409=CARTESIAN_POINT('Ctrl Pts',(-1.17866429440781,-1.,-1.79151291552646));
#27410=CARTESIAN_POINT('Ctrl Pts',(-1.17305363177265,-1.,-1.78852398877523));
#27411=CARTESIAN_POINT('Ctrl Pts',(-1.16747166312239,-1.,-1.78550566040349));
#27412=CARTESIAN_POINT('Ctrl Pts',(-1.16191881298458,-1.,-1.78245795880949));
#27413=CARTESIAN_POINT('Ctrl Pts',(-1.15639547194689,-1.,-1.77938085564261));
#27414=CARTESIAN_POINT('Ctrl Pts',(-1.15090197841531,-1.,-1.77627422557034));
#27415=CARTESIAN_POINT('Ctrl Pts',(-1.14543858226948,-1.,-1.77313777896234));
#27416=CARTESIAN_POINT('Ctrl Pts',(-1.14000548337,-1.,-1.76997111386806));
#27417=CARTESIAN_POINT('Ctrl Pts',(-1.13460291804635,-1.,-1.76677384551883));
#27418=CARTESIAN_POINT('Ctrl Pts',(-1.12923123555076,-1.,-1.76354571966171));
#27419=CARTESIAN_POINT('Ctrl Pts',(-1.12389096855078,-1.,-1.76028671825084));
#27420=CARTESIAN_POINT('Ctrl Pts',(-1.11858293216752,-1.,-1.75699720772089));
#27421=CARTESIAN_POINT('Ctrl Pts',(-1.11330807582542,-1.,-1.75367772094617));
#27422=CARTESIAN_POINT('Ctrl Pts',(-1.10806728183003,-1.,-1.75032866075914));
#27423=CARTESIAN_POINT('Ctrl Pts',(-1.10286118991144,-1.,-1.74695004214924));
#27424=CARTESIAN_POINT('Ctrl Pts',(-1.09768999241229,-1.,-1.74354119236212));
#27425=CARTESIAN_POINT('Ctrl Pts',(-1.09255329056496,-1.,-1.74010053962252));
#27426=CARTESIAN_POINT('Ctrl Pts',(-1.08745056285429,-1.,-1.73662628326093));
#27427=CARTESIAN_POINT('Ctrl Pts',(-1.08238162784749,-1.,-1.73311705663407));
#27428=CARTESIAN_POINT('Ctrl Pts',(-1.0773470373727,-1.,-1.72957248977424));
#27429=CARTESIAN_POINT('Ctrl Pts',(-1.07234866990252,-1.,-1.72599406198489));
#27430=CARTESIAN_POINT('Ctrl Pts',(-1.06738966975463,-1.,-1.72238500928456));
#27431=CARTESIAN_POINT('Ctrl Pts',(-1.0624732468065,-1.,-1.71874858456908));
#27432=CARTESIAN_POINT('Ctrl Pts',(-1.05760163192481,-1.,-1.71508654427022));
#27433=CARTESIAN_POINT('Ctrl Pts',(-1.05277517202854,-1.,-1.71139783543986));
#27434=CARTESIAN_POINT('Ctrl Pts',(-1.0479908540499,-1.,-1.70767646263641));
#27435=CARTESIAN_POINT('Ctrl Pts',(-1.04324363334546,-1.,-1.70391338707969));
#27436=CARTESIAN_POINT('Ctrl Pts',(-1.03852922490782,-1.,-1.70010052930951));
#27437=CARTESIAN_POINT('Ctrl Pts',(-1.03384646003587,-1.,-1.69623414782769));
#27438=CARTESIAN_POINT('Ctrl Pts',(-1.02919977579155,-1.,-1.69231840863471));
#27439=CARTESIAN_POINT('Ctrl Pts',(-1.02460180535272,-1.,-1.68836910178475));
#27440=CARTESIAN_POINT('Ctrl Pts',(-1.02006795074222,-1.,-1.68440578021739));
#27441=CARTESIAN_POINT('Ctrl Pts',(-1.01561026162787,-1.,-1.6804428989482));
#27442=CARTESIAN_POINT('Ctrl Pts',(-1.01123236493507,-1.,-1.67648246776457));
#27443=CARTESIAN_POINT('Ctrl Pts',(-1.00692206696387,-1.,-1.67250335383248));
#27444=CARTESIAN_POINT('Ctrl Pts',(-1.00265091003682,-1.,-1.66846059277231));
#27445=CARTESIAN_POINT('Ctrl Pts',(-0.998389654952317,-1.,-1.66430758030304));
#27446=CARTESIAN_POINT('Ctrl Pts',(-0.994121836661116,-1.,-1.66001553809916));
#27447=CARTESIAN_POINT('Ctrl Pts',(-0.98985562785445,-1.,-1.65559044289746));
#27448=CARTESIAN_POINT('Ctrl Pts',(-0.985642622921626,-1.,-1.6511001661277));
#27449=CARTESIAN_POINT('Ctrl Pts',(-0.981562530940574,-1.,-1.64665139190834));
#27450=CARTESIAN_POINT('Ctrl Pts',(-0.977689794120297,-1.,-1.64233990826831));
#27451=CARTESIAN_POINT('Ctrl Pts',(-0.974066058287501,-1.,-1.63820952658157));
#27452=CARTESIAN_POINT('Ctrl Pts',(-0.970669715996356,-1.,-1.63420665729609));
#27453=CARTESIAN_POINT('Ctrl Pts',(-0.967387853228041,-1.,-1.63013849959083));
#27454=CARTESIAN_POINT('Ctrl Pts',(-0.964046107037821,-1.,-1.6257193066974));
#27455=CARTESIAN_POINT('Ctrl Pts',(-0.960438326099958,-1.,-1.62061638139929));
#27456=CARTESIAN_POINT('Ctrl Pts',(-0.956354422921573,-1.,-1.61449324337233));
#27457=CARTESIAN_POINT('Ctrl Pts',(-0.951613284361248,-1.,-1.60706069897794));
#27458=CARTESIAN_POINT('Ctrl Pts',(-0.946078063325796,-1.,-1.59810042045408));
#27459=CARTESIAN_POINT('Ctrl Pts',(-0.939646377909319,-1.,-1.58744937489796));
#27460=CARTESIAN_POINT('Ctrl Pts',(-0.932246680128849,-1.,-1.57499388385561));
#27461=CARTESIAN_POINT('Ctrl Pts',(-0.923832188966322,-1.,-1.56065988582509));
#27462=CARTESIAN_POINT('Ctrl Pts',(-0.91437591904658,-1.,-1.54440491152808));
#27463=CARTESIAN_POINT('Ctrl Pts',(-0.905967409640499,-1.,-1.52984849890434));
#27464=CARTESIAN_POINT('Ctrl Pts',(-0.89918504749193,-1.,-1.51805569591479));
#27465=CARTESIAN_POINT('Ctrl Pts',(-0.894452006967538,-1.,-1.50980486807181));
#27466=CARTESIAN_POINT('Ctrl Pts',(-0.892032620296855,-1.,-1.5055822144029));
#27467=CARTESIAN_POINT('',(-0.693717979106305,-1.,-1.60662857109684));
#27468=CARTESIAN_POINT('Origin',(0.,-1.,0.));
#27469=CARTESIAN_POINT('',(-0.745574324794401,-1.,-2.0698113262342));
#27470=CARTESIAN_POINT('Ctrl Pts',(-0.693717979106305,-1.,-1.60662857109684));
#27471=CARTESIAN_POINT('Ctrl Pts',(-0.69571209787897,-1.,-1.61106790957619));
#27472=CARTESIAN_POINT('Ctrl Pts',(-0.699605146398837,-1.,-1.61974673471117));
#27473=CARTESIAN_POINT('Ctrl Pts',(-0.705159151977294,-1.,-1.6321654166204));
#27474=CARTESIAN_POINT('Ctrl Pts',(-0.711993139340447,-1.,-1.64752408828442));
#27475=CARTESIAN_POINT('Ctrl Pts',(-0.71958543378795,-1.,-1.66472880551777));
#27476=CARTESIAN_POINT('Ctrl Pts',(-0.726235967982445,-1.,-1.67996158451922));
#27477=CARTESIAN_POINT('Ctrl Pts',(-0.731963238685357,-1.,-1.69326921972915));
#27478=CARTESIAN_POINT('Ctrl Pts',(-0.736799665716932,-1.,-1.70473309004249));
#27479=CARTESIAN_POINT('Ctrl Pts',(-0.74079516202821,-1.,-1.71447789751001));
#27480=CARTESIAN_POINT('Ctrl Pts',(-0.744021445433093,-1.,-1.72268229916769));
#27481=CARTESIAN_POINT('Ctrl Pts',(-0.746574710097752,-1.,-1.72958533647714));
#27482=CARTESIAN_POINT('Ctrl Pts',(-0.74858246295687,-1.,-1.7355035168033));
#27483=CARTESIAN_POINT('Ctrl Pts',(-0.750193435981249,-1.,-1.74080458267114));
#27484=CARTESIAN_POINT('Ctrl Pts',(-0.751555614164482,-1.,-1.74585086852502));
#27485=CARTESIAN_POINT('Ctrl Pts',(-0.752797683531314,-1.,-1.75095139468794));
#27486=CARTESIAN_POINT('Ctrl Pts',(-0.754009254027829,-1.,-1.75631083600019));
#27487=CARTESIAN_POINT('Ctrl Pts',(-0.755220979974461,-1.,-1.76197817240128));
#27488=CARTESIAN_POINT('Ctrl Pts',(-0.75642189602781,-1.,-1.76789396002998));
#27489=CARTESIAN_POINT('Ctrl Pts',(-0.757578264077029,-1.,-1.77394167108292));
#27490=CARTESIAN_POINT('Ctrl Pts',(-0.758650626677518,-1.,-1.77999411220945));
#27491=CARTESIAN_POINT('Ctrl Pts',(-0.759614401110189,-1.,-1.78596964884604));
#27492=CARTESIAN_POINT('Ctrl Pts',(-0.760469555880749,-1.,-1.7918581561088));
#27493=CARTESIAN_POINT('Ctrl Pts',(-0.761229695230558,-1.,-1.79768986997783));
#27494=CARTESIAN_POINT('Ctrl Pts',(-0.761915336443547,-1.,-1.80351583877342));
#27495=CARTESIAN_POINT('Ctrl Pts',(-0.762546129463938,-1.,-1.80938551463965));
#27496=CARTESIAN_POINT('Ctrl Pts',(-0.763132003836634,-1.,-1.8153211840553));
#27497=CARTESIAN_POINT('Ctrl Pts',(-0.763673465462726,-1.,-1.82131873145266));
#27498=CARTESIAN_POINT('Ctrl Pts',(-0.764165902605995,-1.,-1.82735991200065));
#27499=CARTESIAN_POINT('Ctrl Pts',(-0.764602549687853,-1.,-1.83342077227142));
#27500=CARTESIAN_POINT('Ctrl Pts',(-0.764978057881737,-1.,-1.83948181064835));
#27501=CARTESIAN_POINT('Ctrl Pts',(-0.765291664862029,-1.,-1.84553698875924));
#27502=CARTESIAN_POINT('Ctrl Pts',(-0.765545710619062,-1.,-1.85158945130063));
#27503=CARTESIAN_POINT('Ctrl Pts',(-0.765744212909318,-1.,-1.85764741390394));
#27504=CARTESIAN_POINT('Ctrl Pts',(-0.765891519092547,-1.,-1.86372027063312));
#27505=CARTESIAN_POINT('Ctrl Pts',(-0.765990708546091,-1.,-1.86981398314341));
#27506=CARTESIAN_POINT('Ctrl Pts',(-0.766042837036744,-1.,-1.87592888967883));
#27507=CARTESIAN_POINT('Ctrl Pts',(-0.766047794851865,-1.,-1.88206215302561));
#27508=CARTESIAN_POINT('Ctrl Pts',(-0.766004837062091,-1.,-1.88820926433409));
#27509=CARTESIAN_POINT('Ctrl Pts',(-0.765913193856978,-1.,-1.89436577771388));
#27510=CARTESIAN_POINT('Ctrl Pts',(-0.765772772593386,-1.,-1.90052930393596));
#27511=CARTESIAN_POINT('Ctrl Pts',(-0.765584196937919,-1.,-1.90669961402356));
#27512=CARTESIAN_POINT('Ctrl Pts',(-0.765348465884722,-1.,-1.91287765805169));
#27513=CARTESIAN_POINT('Ctrl Pts',(-0.765066729667088,-1.,-1.91906491634196));
#27514=CARTESIAN_POINT('Ctrl Pts',(-0.764740025488211,-1.,-1.92526263537048));
#27515=CARTESIAN_POINT('Ctrl Pts',(-0.764369010673941,-1.,-1.93147105496382));
#27516=CARTESIAN_POINT('Ctrl Pts',(-0.763954049121458,-1.,-1.93768964875886));
#27517=CARTESIAN_POINT('Ctrl Pts',(-0.763495333538629,-1.,-1.9439174661764));
#27518=CARTESIAN_POINT('Ctrl Pts',(-0.762992990878769,-1.,-1.95015342590024));
#27519=CARTESIAN_POINT('Ctrl Pts',(-0.762447203806179,-1.,-1.95639665309869));
#27520=CARTESIAN_POINT('Ctrl Pts',(-0.761858300014423,-1.,-1.96264672744186));
#27521=CARTESIAN_POINT('Ctrl Pts',(-0.76122669048382,-1.,-1.96890351582499));
#27522=CARTESIAN_POINT('Ctrl Pts',(-0.760552825409757,-1.,-1.97516705321494));
#27523=CARTESIAN_POINT('Ctrl Pts',(-0.75983714745219,-1.,-1.98143741418172));
#27524=CARTESIAN_POINT('Ctrl Pts',(-0.759080037802488,-1.,-1.98771456680874));
#27525=CARTESIAN_POINT('Ctrl Pts',(-0.758281796766761,-1.,-1.99399831098817));
#27526=CARTESIAN_POINT('Ctrl Pts',(-0.757442676862724,-1.,-2.00028834739178));
#27527=CARTESIAN_POINT('Ctrl Pts',(-0.75656290464667,-1.,-2.0065843158773));
#27528=CARTESIAN_POINT('Ctrl Pts',(-0.755642704957865,-1.,-2.01288584328084));
#27529=CARTESIAN_POINT('Ctrl Pts',(-0.754682330722816,-1.,-2.01919259405809));
#27530=CARTESIAN_POINT('Ctrl Pts',(-0.753682061112768,-1.,-2.02550428623313));
#27531=CARTESIAN_POINT('Ctrl Pts',(-0.752642180487211,-1.,-2.03182068456221));
#27532=CARTESIAN_POINT('Ctrl Pts',(-0.751562963361115,-1.,-2.03814160092099));
#27533=CARTESIAN_POINT('Ctrl Pts',(-0.750444657875576,-1.,-2.04446689147979));
#27534=CARTESIAN_POINT('Ctrl Pts',(-0.749287468665046,-1.,-2.05079645592154));
#27535=CARTESIAN_POINT('Ctrl Pts',(-0.748091554183802,-1.,-2.05713023031006));
#27536=CARTESIAN_POINT('Ctrl Pts',(-0.747103932787919,-1.,-2.06220058927826));
#27537=CARTESIAN_POINT('Ctrl Pts',(-0.7463458715442,-1.,-2.06600523016815));
#27538=CARTESIAN_POINT('Ctrl Pts',(-0.745832791378367,-1.,-2.06854248895728));
#27539=CARTESIAN_POINT('Ctrl Pts',(-0.745574324794401,-1.,-2.0698113262342));
#27540=CARTESIAN_POINT('',(-0.61342227326009,-1.,-2.11275013067528));
#27541=CARTESIAN_POINT('',(-0.745574324794401,-1.,-2.0698113262342));
#27542=CARTESIAN_POINT('',(-0.383122945602004,-1.,-1.7075470150345));
#27543=CARTESIAN_POINT('Ctrl Pts',(-0.61342227326009,-1.,-2.11275013067528));
#27544=CARTESIAN_POINT('Ctrl Pts',(-0.6124673655618,-1.,-2.11187554259986));
#27545=CARTESIAN_POINT('Ctrl Pts',(-0.610560911689899,-1.,-2.11012443807238));
#27546=CARTESIAN_POINT('Ctrl Pts',(-0.607711315454876,-1.,-2.1074919961518));
#27547=CARTESIAN_POINT('Ctrl Pts',(-0.60393203073603,-1.,-2.10397049886949));
#27548=CARTESIAN_POINT('Ctrl Pts',(-0.599241616420533,-1.,-2.0995493086477));
#27549=CARTESIAN_POINT('Ctrl Pts',(-0.594585006052162,-1.,-2.0951087622027));
#27550=CARTESIAN_POINT('Ctrl Pts',(-0.589962365403406,-1.,-2.09064881812129));
#27551=CARTESIAN_POINT('Ctrl Pts',(-0.585373918991617,-1.,-2.08616943727951));
#27552=CARTESIAN_POINT('Ctrl Pts',(-0.580819952108063,-1.,-2.08167059018418));
#27553=CARTESIAN_POINT('Ctrl Pts',(-0.576300797416844,-1.,-2.07715226767559));
#27554=CARTESIAN_POINT('Ctrl Pts',(-0.571816823242603,-1.,-2.07261449292824));
#27555=CARTESIAN_POINT('Ctrl Pts',(-0.567368421181087,-1.,-2.06805732997334));
#27556=CARTESIAN_POINT('Ctrl Pts',(-0.562955993082261,-1.,-2.06348090160589));
#27557=CARTESIAN_POINT('Ctrl Pts',(-0.558579940185151,-1.,-2.05888537756462));
#27558=CARTESIAN_POINT('Ctrl Pts',(-0.554240657463906,-1.,-2.05427091604413));
#27559=CARTESIAN_POINT('Ctrl Pts',(-0.549938525150295,-1.,-2.04963761077958));
#27560=CARTESIAN_POINT('Ctrl Pts',(-0.54567390381743,-1.,-2.04498544714588));
#27561=CARTESIAN_POINT('Ctrl Pts',(-0.541447120615659,-1.,-2.04031422690527));
#27562=CARTESIAN_POINT('Ctrl Pts',(-0.537258489833262,-1.,-2.03562362954037));
#27563=CARTESIAN_POINT('Ctrl Pts',(-0.533108355132977,-1.,-2.03091336214426));
#27564=CARTESIAN_POINT('Ctrl Pts',(-0.528997127241914,-1.,-2.0261832908329));
#27565=CARTESIAN_POINT('Ctrl Pts',(-0.524925318333476,-1.,-2.02143356304698));
#27566=CARTESIAN_POINT('Ctrl Pts',(-0.52089359039937,-1.,-2.01666477917286));
#27567=CARTESIAN_POINT('Ctrl Pts',(-0.516902681728687,-1.,-2.01187773939242));
#27568=CARTESIAN_POINT('Ctrl Pts',(-0.512953306961792,-1.,-2.00707309946949));
#27569=CARTESIAN_POINT('Ctrl Pts',(-0.509046069886157,-1.,-2.00225107134734));
#27570=CARTESIAN_POINT('Ctrl Pts',(-0.505181361323026,-1.,-1.99741107463572));
#27571=CARTESIAN_POINT('Ctrl Pts',(-0.501359287727146,-1.,-1.99255149126155));
#27572=CARTESIAN_POINT('Ctrl Pts',(-0.497579909545574,-1.,-1.98767044752932));
#27573=CARTESIAN_POINT('Ctrl Pts',(-0.493843476541495,-1.,-1.98276658761821));
#27574=CARTESIAN_POINT('Ctrl Pts',(-0.490150627860952,-1.,-1.97783973019229));
#27575=CARTESIAN_POINT('Ctrl Pts',(-0.486502692907659,-1.,-1.97289186263272));
#27576=CARTESIAN_POINT('Ctrl Pts',(-0.482901662120691,-1.,-1.96792703422362));
#27577=CARTESIAN_POINT('Ctrl Pts',(-0.479349583074855,-1.,-1.96294933055943));
#27578=CARTESIAN_POINT('Ctrl Pts',(-0.475848034683176,-1.,-1.95796111148177));
#27579=CARTESIAN_POINT('Ctrl Pts',(-0.472397672264072,-1.,-1.95296148278133));
#27580=CARTESIAN_POINT('Ctrl Pts',(-0.468997482913135,-1.,-1.94794381136514));
#27581=CARTESIAN_POINT('Ctrl Pts',(-0.46564546202603,-1.,-1.9428979419619));
#27582=CARTESIAN_POINT('Ctrl Pts',(-0.462340031009056,-1.,-1.93781486640821));
#27583=CARTESIAN_POINT('Ctrl Pts',(-0.459081234547926,-1.,-1.93269066517934));
#27584=CARTESIAN_POINT('Ctrl Pts',(-0.455872005174371,-1.,-1.92753067150476));
#27585=CARTESIAN_POINT('Ctrl Pts',(-0.452719478359432,-1.,-1.92235380648502));
#27586=CARTESIAN_POINT('Ctrl Pts',(-0.449632260106662,-1.,-1.91718342555755));
#27587=CARTESIAN_POINT('Ctrl Pts',(-0.446617343485711,-1.,-1.9120369998112));
#27588=CARTESIAN_POINT('Ctrl Pts',(-0.443677556849151,-1.,-1.90691756144898));
#27589=CARTESIAN_POINT('Ctrl Pts',(-0.440807833704038,-1.,-1.90180124389086));
#27590=CARTESIAN_POINT('Ctrl Pts',(-0.437995003948244,-1.,-1.89663648956466));
#27591=CARTESIAN_POINT('Ctrl Pts',(-0.435225660963383,-1.,-1.89136993975504));
#27592=CARTESIAN_POINT('Ctrl Pts',(-0.432493038548748,-1.,-1.88596913666793));
#27593=CARTESIAN_POINT('Ctrl Pts',(-0.429803062482344,-1.,-1.88044229001832));
#27594=CARTESIAN_POINT('Ctrl Pts',(-0.427183828519102,-1.,-1.87486989291484));
#27595=CARTESIAN_POINT('Ctrl Pts',(-0.424678177291359,-1.,-1.86937803944323));
#27596=CARTESIAN_POINT('Ctrl Pts',(-0.422327307418275,-1.,-1.86408083334028));
#27597=CARTESIAN_POINT('Ctrl Pts',(-0.420157287975619,-1.,-1.85903281096686));
#27598=CARTESIAN_POINT('Ctrl Pts',(-0.418164129143534,-1.,-1.85417632856234));
#27599=CARTESIAN_POINT('Ctrl Pts',(-0.416300022038864,-1.,-1.84929312929882));
#27600=CARTESIAN_POINT('Ctrl Pts',(-0.41448743825434,-1.,-1.8440575707371));
#27601=CARTESIAN_POINT('Ctrl Pts',(-0.412633125322162,-1.,-1.83808953475839));
#27602=CARTESIAN_POINT('Ctrl Pts',(-0.410641256301675,-1.,-1.83100408895216));
#27603=CARTESIAN_POINT('Ctrl Pts',(-0.408428948108533,-1.,-1.8224702267854));
#27604=CARTESIAN_POINT('Ctrl Pts',(-0.405933518411838,-1.,-1.81223801813988));
#27605=CARTESIAN_POINT('Ctrl Pts',(-0.403107976170441,-1.,-1.80012077176221));
#27606=CARTESIAN_POINT('Ctrl Pts',(-0.39991940378308,-1.,-1.78598826347533));
#27607=CARTESIAN_POINT('Ctrl Pts',(-0.39634619612042,-1.,-1.7697556004756));
#27608=CARTESIAN_POINT('Ctrl Pts',(-0.392375812294307,-1.,-1.75137405313962));
#27609=CARTESIAN_POINT('Ctrl Pts',(-0.388877023509191,-1.,-1.7349317097561));
#27610=CARTESIAN_POINT('Ctrl Pts',(-0.38607079032701,-1.,-1.72162022246158));
#27611=CARTESIAN_POINT('Ctrl Pts',(-0.384119047315542,-1.,-1.71231062891958));
#27612=CARTESIAN_POINT('Ctrl Pts',(-0.383122945602004,-1.,-1.7075470150345));
#27613=CARTESIAN_POINT('',(-0.163289472382896,-1.,-1.74236521665491));
#27614=CARTESIAN_POINT('Origin',(0.,-1.,0.));
#27615=CARTESIAN_POINT('',(-0.0694764450219581,-1.,-2.19890268624765));
#27616=CARTESIAN_POINT('Ctrl Pts',(-0.163289472382896,-1.,-1.74236521665491));
#27617=CARTESIAN_POINT('Ctrl Pts',(-0.163814161002002,-1.,-1.7472034950333));
#27618=CARTESIAN_POINT('Ctrl Pts',(-0.164834765707158,-1.,-1.75666056638427));
#27619=CARTESIAN_POINT('Ctrl Pts',(-0.1662793551464,-1.,-1.77018771684844));
#27620=CARTESIAN_POINT('Ctrl Pts',(-0.168032772805197,-1.,-1.7869064998507));
#27621=CARTESIAN_POINT('Ctrl Pts',(-0.169936923904608,-1.,-1.80561530629706));
#27622=CARTESIAN_POINT('Ctrl Pts',(-0.171554770204119,-1.,-1.82215766811545));
#27623=CARTESIAN_POINT('Ctrl Pts',(-0.1728894428919,-1.,-1.83658380527692));
#27624=CARTESIAN_POINT('Ctrl Pts',(-0.173946627587731,-1.,-1.8489811319852));
#27625=CARTESIAN_POINT('Ctrl Pts',(-0.17473525927603,-1.,-1.85948367088837));
#27626=CARTESIAN_POINT('Ctrl Pts',(-0.175268337590758,-1.,-1.86828349694799));
#27627=CARTESIAN_POINT('Ctrl Pts',(-0.175563480746485,-1.,-1.87563767773588));
#27628=CARTESIAN_POINT('Ctrl Pts',(-0.175644148889699,-1.,-1.88188663145367));
#27629=CARTESIAN_POINT('Ctrl Pts',(-0.175538155840648,-1.,-1.88742606273259));
#27630=CARTESIAN_POINT('Ctrl Pts',(-0.175274276190844,-1.,-1.892646301985));
#27631=CARTESIAN_POINT('Ctrl Pts',(-0.174879405091263,-1.,-1.89788101117132));
#27632=CARTESIAN_POINT('Ctrl Pts',(-0.174375518661085,-1.,-1.90335253862834));
#27633=CARTESIAN_POINT('Ctrl Pts',(-0.173776635257817,-1.,-1.90911693975267));
#27634=CARTESIAN_POINT('Ctrl Pts',(-0.173090695383496,-1.,-1.91511429159527));
#27635=CARTESIAN_POINT('Ctrl Pts',(-0.172321621259514,-1.,-1.9212233439798));
#27636=CARTESIAN_POINT('Ctrl Pts',(-0.171471191532988,-1.,-1.92731093582036));
#27637=CARTESIAN_POINT('Ctrl Pts',(-0.170541253116202,-1.,-1.93329183155539));
#27638=CARTESIAN_POINT('Ctrl Pts',(-0.169534904817491,-1.,-1.93915639211581));
#27639=CARTESIAN_POINT('Ctrl Pts',(-0.168455741607556,-1.,-1.94493757756931));
#27640=CARTESIAN_POINT('Ctrl Pts',(-0.167307501784475,-1.,-1.95069027794294));
#27641=CARTESIAN_POINT('Ctrl Pts',(-0.166093592002812,-1.,-1.9564675971873));
#27642=CARTESIAN_POINT('Ctrl Pts',(-0.164816568920269,-1.,-1.96229379940136));
#27643=CARTESIAN_POINT('Ctrl Pts',(-0.163478185457734,-1.,-1.96816512677967));
#27644=CARTESIAN_POINT('Ctrl Pts',(-0.162079693556289,-1.,-1.97406280235188));
#27645=CARTESIAN_POINT('Ctrl Pts',(-0.160622060784611,-1.,-1.97996195437559));
#27646=CARTESIAN_POINT('Ctrl Pts',(-0.159106226437299,-1.,-1.98584238283292));
#27647=CARTESIAN_POINT('Ctrl Pts',(-0.157533331459227,-1.,-1.99169810931908));
#27648=CARTESIAN_POINT('Ctrl Pts',(-0.155904629548783,-1.,-1.99753284771497));
#27649=CARTESIAN_POINT('Ctrl Pts',(-0.154221403049722,-1.,-2.00335565310543));
#27650=CARTESIAN_POINT('Ctrl Pts',(-0.15248488362145,-1.,-2.00917680318424));
#27651=CARTESIAN_POINT('Ctrl Pts',(-0.150696157673078,-1.,-2.01500291940238));
#27652=CARTESIAN_POINT('Ctrl Pts',(-0.148856124775337,-1.,-2.02083464969894));
#27653=CARTESIAN_POINT('Ctrl Pts',(-0.146965557332583,-1.,-2.02666926182017));
#27654=CARTESIAN_POINT('Ctrl Pts',(-0.145025140186057,-1.,-2.03250223739942));
#27655=CARTESIAN_POINT('Ctrl Pts',(-0.143035515058209,-1.,-2.03832911025912));
#27656=CARTESIAN_POINT('Ctrl Pts',(-0.140997332152546,-1.,-2.04414757947916));
#27657=CARTESIAN_POINT('Ctrl Pts',(-0.138911255368966,-1.,-2.04995762001328));
#27658=CARTESIAN_POINT('Ctrl Pts',(-0.136777941218044,-1.,-2.05576044414264));
#27659=CARTESIAN_POINT('Ctrl Pts',(-0.134598026192106,-1.,-2.06155781517842));
#27660=CARTESIAN_POINT('Ctrl Pts',(-0.13237211154771,-1.,-2.06735123910326));
#27661=CARTESIAN_POINT('Ctrl Pts',(-0.130100748328403,-1.,-2.07314114713063));
#27662=CARTESIAN_POINT('Ctrl Pts',(-0.12778444527612,-1.,-2.07892715110987));
#27663=CARTESIAN_POINT('Ctrl Pts',(-0.125423679412061,-1.,-2.08470840653643));
#27664=CARTESIAN_POINT('Ctrl Pts',(-0.123018905621083,-1.,-2.09048392424825));
#27665=CARTESIAN_POINT('Ctrl Pts',(-0.120570567965122,-1.,-2.0962529286773));
#27666=CARTESIAN_POINT('Ctrl Pts',(-0.118079107988355,-1.,-2.102015121329));
#27667=CARTESIAN_POINT('Ctrl Pts',(-0.115544957687926,-1.,-2.10777050261309));
#27668=CARTESIAN_POINT('Ctrl Pts',(-0.112968534419737,-1.,-2.11351924490306));
#27669=CARTESIAN_POINT('Ctrl Pts',(-0.110350236135025,-1.,-2.11926155590865));
#27670=CARTESIAN_POINT('Ctrl Pts',(-0.10769043523109,-1.,-2.12499752307));
#27671=CARTESIAN_POINT('Ctrl Pts',(-0.104989479152739,-1.,-2.13072704887293));
#27672=CARTESIAN_POINT('Ctrl Pts',(-0.1022477005561,-1.,-2.13644992667165));
#27673=CARTESIAN_POINT('Ctrl Pts',(-0.0994654261990915,-1.,-2.14216588396025));
#27674=CARTESIAN_POINT('Ctrl Pts',(-0.0966429852305459,-1.,-2.14787463531795));
#27675=CARTESIAN_POINT('Ctrl Pts',(-0.0937807218867643,-1.,-2.1535759397817));
#27676=CARTESIAN_POINT('Ctrl Pts',(-0.0908789888107265,-1.,-2.15926961544516));
#27677=CARTESIAN_POINT('Ctrl Pts',(-0.0879381291386923,-1.,-2.16495552645014));
#27678=CARTESIAN_POINT('Ctrl Pts',(-0.0849584620835372,-1.,-2.17063357870952));
#27679=CARTESIAN_POINT('Ctrl Pts',(-0.0819402680872765,-1.,-2.176303712113));
#27680=CARTESIAN_POINT('Ctrl Pts',(-0.0788837727685243,-1.,-2.18196589448887));
#27681=CARTESIAN_POINT('Ctrl Pts',(-0.0757891465836148,-1.,-2.1876201139953));
#27682=CARTESIAN_POINT('Ctrl Pts',(-0.0732830357306725,-1.,-2.19213712013662));
#27683=CARTESIAN_POINT('Ctrl Pts',(-0.0713863779526154,-1.,-2.19552129484002));
#27684=CARTESIAN_POINT('Ctrl Pts',(-0.070114353632549,-1.,-2.19777582085423));
#27685=CARTESIAN_POINT('Ctrl Pts',(-0.0694764450219581,-1.,-2.19890268624765));
#27686=CARTESIAN_POINT('',(0.0694764450219584,-1.,-2.19890268624765));
#27687=CARTESIAN_POINT('',(-0.0694764450219581,-1.,-2.19890268624765));
#27688=CARTESIAN_POINT('',(0.163289472382896,-1.,-1.74236521665491));
#27689=CARTESIAN_POINT('Ctrl Pts',(0.0694764450219584,-1.,-2.19890268624765));
#27690=CARTESIAN_POINT('Ctrl Pts',(0.0701143536324926,-1.,-2.19777582085261));
#27691=CARTESIAN_POINT('Ctrl Pts',(0.0713863779524627,-1.,-2.19552129483562));
#27692=CARTESIAN_POINT('Ctrl Pts',(0.0732830357304276,-1.,-2.19213712012956));
#27693=CARTESIAN_POINT('Ctrl Pts',(0.0757891465833411,-1.,-2.1876201139874));
#27694=CARTESIAN_POINT('Ctrl Pts',(0.0788837727683228,-1.,-2.18196589448304));
#27695=CARTESIAN_POINT('Ctrl Pts',(0.0819402680871939,-1.,-2.1763037121106));
#27696=CARTESIAN_POINT('Ctrl Pts',(0.0849584620835643,-1.,-2.17063357871031));
#27697=CARTESIAN_POINT('Ctrl Pts',(0.0879381291387823,-1.,-2.16495552645275));
#27698=CARTESIAN_POINT('Ctrl Pts',(0.0908789888108266,-1.,-2.15926961544808));
#27699=CARTESIAN_POINT('Ctrl Pts',(0.0937807218868345,-1.,-2.15357593978377));
#27700=CARTESIAN_POINT('Ctrl Pts',(0.0966429852305689,-1.,-2.14787463531864));
#27701=CARTESIAN_POINT('Ctrl Pts',(0.0994654261990743,-1.,-2.14216588395974));
#27702=CARTESIAN_POINT('Ctrl Pts',(0.102247700556064,-1.,-2.13644992667052));
#27703=CARTESIAN_POINT('Ctrl Pts',(0.104989479152703,-1.,-2.1307270488718));
#27704=CARTESIAN_POINT('Ctrl Pts',(0.107690435231068,-1.,-2.12499752306927));
#27705=CARTESIAN_POINT('Ctrl Pts',(0.11035023613502,-1.,-2.11926155590849));
#27706=CARTESIAN_POINT('Ctrl Pts',(0.112968534419746,-1.,-2.11351924490335));
#27707=CARTESIAN_POINT('Ctrl Pts',(0.11554495768794,-1.,-2.10777050261359));
#27708=CARTESIAN_POINT('Ctrl Pts',(0.118079107988368,-1.,-2.10201512132945));
#27709=CARTESIAN_POINT('Ctrl Pts',(0.120570567965129,-1.,-2.09625292867756));
#27710=CARTESIAN_POINT('Ctrl Pts',(0.123018905621083,-1.,-2.09048392424826));
#27711=CARTESIAN_POINT('Ctrl Pts',(0.125423679412058,-1.,-2.08470840653628));
#27712=CARTESIAN_POINT('Ctrl Pts',(0.127784445276116,-1.,-2.07892715110967));
#27713=CARTESIAN_POINT('Ctrl Pts',(0.1301007483284,-1.,-2.07314114713047));
#27714=CARTESIAN_POINT('Ctrl Pts',(0.13237211154771,-1.,-2.06735123910319));
#27715=CARTESIAN_POINT('Ctrl Pts',(0.134598026192107,-1.,-2.06155781517844));
#27716=CARTESIAN_POINT('Ctrl Pts',(0.136777941218044,-1.,-2.0557604441427));
#27717=CARTESIAN_POINT('Ctrl Pts',(0.138911255368966,-1.,-2.04995762001333));
#27718=CARTESIAN_POINT('Ctrl Pts',(0.140997332152545,-1.,-2.04414757947919));
#27719=CARTESIAN_POINT('Ctrl Pts',(0.143035515058208,-1.,-2.03832911025913));
#27720=CARTESIAN_POINT('Ctrl Pts',(0.145025140186058,-1.,-2.03250223739941));
#27721=CARTESIAN_POINT('Ctrl Pts',(0.146965557332586,-1.,-2.02666926182017));
#27722=CARTESIAN_POINT('Ctrl Pts',(0.148856124775343,-1.,-2.02083464969897));
#27723=CARTESIAN_POINT('Ctrl Pts',(0.150696157673084,-1.,-2.01500291940243));
#27724=CARTESIAN_POINT('Ctrl Pts',(0.152484883621452,-1.,-2.00917680318426));
#27725=CARTESIAN_POINT('Ctrl Pts',(0.154221403049719,-1.,-2.00335565310539));
#27726=CARTESIAN_POINT('Ctrl Pts',(0.155904629548774,-1.,-1.99753284771487));
#27727=CARTESIAN_POINT('Ctrl Pts',(0.157533331459215,-1.,-1.99169810931893));
#27728=CARTESIAN_POINT('Ctrl Pts',(0.159106226437288,-1.,-1.98584238283279));
#27729=CARTESIAN_POINT('Ctrl Pts',(0.16062206078461,-1.,-1.97996195437557));
#27730=CARTESIAN_POINT('Ctrl Pts',(0.162079693556302,-1.,-1.97406280235204));
#27731=CARTESIAN_POINT('Ctrl Pts',(0.16347818545776,-1.,-1.96816512678));
#27732=CARTESIAN_POINT('Ctrl Pts',(0.1648165689203,-1.,-1.96229379940174));
#27733=CARTESIAN_POINT('Ctrl Pts',(0.166093592002833,-1.,-1.95646759718755));
#27734=CARTESIAN_POINT('Ctrl Pts',(0.167307501784469,-1.,-1.95069027794286));
#27735=CARTESIAN_POINT('Ctrl Pts',(0.168455741607516,-1.,-1.94493757756879));
#27736=CARTESIAN_POINT('Ctrl Pts',(0.169534904817425,-1.,-1.93915639211497));
#27737=CARTESIAN_POINT('Ctrl Pts',(0.170541253116136,-1.,-1.93329183155455));
#27738=CARTESIAN_POINT('Ctrl Pts',(0.17147119153296,-1.,-1.92731093582));
#27739=CARTESIAN_POINT('Ctrl Pts',(0.172321621259557,-1.,-1.92122334398034));
#27740=CARTESIAN_POINT('Ctrl Pts',(0.173090695383619,-1.,-1.91511429159681));
#27741=CARTESIAN_POINT('Ctrl Pts',(0.173776635257984,-1.,-1.90911693975475));
#27742=CARTESIAN_POINT('Ctrl Pts',(0.174375518661222,-1.,-1.90335253863003));
#27743=CARTESIAN_POINT('Ctrl Pts',(0.174879405091277,-1.,-1.89788101117148));
#27744=CARTESIAN_POINT('Ctrl Pts',(0.175274276190664,-1.,-1.89264630198279));
#27745=CARTESIAN_POINT('Ctrl Pts',(0.175538155840286,-1.,-1.88742606272818));
#27746=CARTESIAN_POINT('Ctrl Pts',(0.175644148889271,-1.,-1.88188663144846));
#27747=CARTESIAN_POINT('Ctrl Pts',(0.175563480746205,-1.,-1.87563767773249));
#27748=CARTESIAN_POINT('Ctrl Pts',(0.175268337590901,-1.,-1.86828349694972));
#27749=CARTESIAN_POINT('Ctrl Pts',(0.174735259276856,-1.,-1.85948367089838));
#27750=CARTESIAN_POINT('Ctrl Pts',(0.173946627589401,-1.,-1.84898113200543));
#27751=CARTESIAN_POINT('Ctrl Pts',(0.17288944289442,-1.,-1.83658380530747));
#27752=CARTESIAN_POINT('Ctrl Pts',(0.171554770207306,-1.,-1.82215766815414));
#27753=CARTESIAN_POINT('Ctrl Pts',(0.169936923908078,-1.,-1.80561530633924));
#27754=CARTESIAN_POINT('Ctrl Pts',(0.16803277280837,-1.,-1.78690649988931));
#27755=CARTESIAN_POINT('Ctrl Pts',(0.166279355148738,-1.,-1.77018771687692));
#27756=CARTESIAN_POINT('Ctrl Pts',(0.164834765708484,-1.,-1.75666056640041));
#27757=CARTESIAN_POINT('Ctrl Pts',(0.163814161002474,-1.,-1.74720349503904));
#27758=CARTESIAN_POINT('Ctrl Pts',(0.163289472382896,-1.,-1.74236521665491));
#27759=CARTESIAN_POINT('',(0.383122945602004,-1.,-1.7075470150345));
#27760=CARTESIAN_POINT('Origin',(0.,-1.,0.));
#27761=CARTESIAN_POINT('',(0.61342227326009,-1.,-2.11275013067528));
#27762=CARTESIAN_POINT('Ctrl Pts',(0.383122945602004,-1.,-1.7075470150345));
#27763=CARTESIAN_POINT('Ctrl Pts',(0.384119047314215,-1.,-1.71231062891398));
#27764=CARTESIAN_POINT('Ctrl Pts',(0.386070790323281,-1.,-1.72162022244582));
#27765=CARTESIAN_POINT('Ctrl Pts',(0.388877023502615,-1.,-1.73493170972829));
#27766=CARTESIAN_POINT('Ctrl Pts',(0.392375812285395,-1.,-1.75137405310193));
#27767=CARTESIAN_POINT('Ctrl Pts',(0.396346196110688,-1.,-1.76975560043442));
#27768=CARTESIAN_POINT('Ctrl Pts',(0.399919403774155,-1.,-1.78598826343754));
#27769=CARTESIAN_POINT('Ctrl Pts',(0.403107976163396,-1.,-1.80012077173238));
#27770=CARTESIAN_POINT('Ctrl Pts',(0.405933518407175,-1.,-1.81223801812013));
#27771=CARTESIAN_POINT('Ctrl Pts',(0.408428948106227,-1.,-1.82247022677562));
#27772=CARTESIAN_POINT('Ctrl Pts',(0.410641256301276,-1.,-1.83100408895047));
#27773=CARTESIAN_POINT('Ctrl Pts',(0.412633125322945,-1.,-1.8380895347617));
#27774=CARTESIAN_POINT('Ctrl Pts',(0.414487438255542,-1.,-1.84405757074218));
#27775=CARTESIAN_POINT('Ctrl Pts',(0.416300022039885,-1.,-1.84929312930314));
#27776=CARTESIAN_POINT('Ctrl Pts',(0.418164129144045,-1.,-1.8541763285645));
#27777=CARTESIAN_POINT('Ctrl Pts',(0.420157287975583,-1.,-1.8590328109667));
#27778=CARTESIAN_POINT('Ctrl Pts',(0.422327307417884,-1.,-1.86408083333863));
#27779=CARTESIAN_POINT('Ctrl Pts',(0.424678177290876,-1.,-1.8693780394412));
#27780=CARTESIAN_POINT('Ctrl Pts',(0.427183828518743,-1.,-1.87486989291334));
#27781=CARTESIAN_POINT('Ctrl Pts',(0.429803062482217,-1.,-1.88044229001779));
#27782=CARTESIAN_POINT('Ctrl Pts',(0.432493038548833,-1.,-1.88596913666828));
#27783=CARTESIAN_POINT('Ctrl Pts',(0.43522566096358,-1.,-1.89136993975585));
#27784=CARTESIAN_POINT('Ctrl Pts',(0.437995003948443,-1.,-1.89663648956549));
#27785=CARTESIAN_POINT('Ctrl Pts',(0.44080783370416,-1.,-1.90180124389137));
#27786=CARTESIAN_POINT('Ctrl Pts',(0.44367755684917,-1.,-1.90691756144906));
#27787=CARTESIAN_POINT('Ctrl Pts',(0.446617343485651,-1.,-1.91203699981095));
#27788=CARTESIAN_POINT('Ctrl Pts',(0.449632260106572,-1.,-1.91718342555717));
#27789=CARTESIAN_POINT('Ctrl Pts',(0.452719478359356,-1.,-1.9223538064847));
#27790=CARTESIAN_POINT('Ctrl Pts',(0.455872005174335,-1.,-1.92753067150461));
#27791=CARTESIAN_POINT('Ctrl Pts',(0.459081234547931,-1.,-1.93269066517936));
#27792=CARTESIAN_POINT('Ctrl Pts',(0.462340031009087,-1.,-1.93781486640834));
#27793=CARTESIAN_POINT('Ctrl Pts',(0.465645462026064,-1.,-1.94289794196205));
#27794=CARTESIAN_POINT('Ctrl Pts',(0.468997482913158,-1.,-1.94794381136524));
#27795=CARTESIAN_POINT('Ctrl Pts',(0.472397672264079,-1.,-1.95296148278136));
#27796=CARTESIAN_POINT('Ctrl Pts',(0.475848034683171,-1.,-1.95796111148175));
#27797=CARTESIAN_POINT('Ctrl Pts',(0.479349583074846,-1.,-1.96294933055938));
#27798=CARTESIAN_POINT('Ctrl Pts',(0.482901662120686,-1.,-1.96792703422358));
#27799=CARTESIAN_POINT('Ctrl Pts',(0.486502692907661,-1.,-1.97289186263272));
#27800=CARTESIAN_POINT('Ctrl Pts',(0.490150627860955,-1.,-1.97783973019229));
#27801=CARTESIAN_POINT('Ctrl Pts',(0.493843476541492,-1.,-1.9827665876182));
#27802=CARTESIAN_POINT('Ctrl Pts',(0.497579909545564,-1.,-1.98767044752929));
#27803=CARTESIAN_POINT('Ctrl Pts',(0.501359287727129,-1.,-1.9925514912615));
#27804=CARTESIAN_POINT('Ctrl Pts',(0.505181361323011,-1.,-1.99741107463567));
#27805=CARTESIAN_POINT('Ctrl Pts',(0.509046069886152,-1.,-2.00225107134733));
#27806=CARTESIAN_POINT('Ctrl Pts',(0.512953306961813,-1.,-2.00707309946955));
#27807=CARTESIAN_POINT('Ctrl Pts',(0.516902681728733,-1.,-2.01187773939257));
#27808=CARTESIAN_POINT('Ctrl Pts',(0.520893590399428,-1.,-2.01666477917306));
#27809=CARTESIAN_POINT('Ctrl Pts',(0.524925318333518,-1.,-2.02143356304712));
#27810=CARTESIAN_POINT('Ctrl Pts',(0.52899712724191,-1.,-2.02618329083289));
#27811=CARTESIAN_POINT('Ctrl Pts',(0.533108355132905,-1.,-2.03091336214401));
#27812=CARTESIAN_POINT('Ctrl Pts',(0.537258489833134,-1.,-2.03562362953993));
#27813=CARTESIAN_POINT('Ctrl Pts',(0.54144712061552,-1.,-2.0403142269048));
#27814=CARTESIAN_POINT('Ctrl Pts',(0.545673903817348,-1.,-2.0449854471456));
#27815=CARTESIAN_POINT('Ctrl Pts',(0.549938525150342,-1.,-2.04963761077974));
#27816=CARTESIAN_POINT('Ctrl Pts',(0.554240657464109,-1.,-2.05427091604482));
#27817=CARTESIAN_POINT('Ctrl Pts',(0.558579940185467,-1.,-2.05888537756571));
#27818=CARTESIAN_POINT('Ctrl Pts',(0.562955993082574,-1.,-2.06348090160697));
#27819=CARTESIAN_POINT('Ctrl Pts',(0.567368421181229,-1.,-2.06805732997383));
#27820=CARTESIAN_POINT('Ctrl Pts',(0.571816823242411,-1.,-2.07261449292758));
#27821=CARTESIAN_POINT('Ctrl Pts',(0.576300797416274,-1.,-2.07715226767361));
#27822=CARTESIAN_POINT('Ctrl Pts',(0.580819952107256,-1.,-2.08167059018138));
#27823=CARTESIAN_POINT('Ctrl Pts',(0.585373918990895,-1.,-2.086169437277));
#27824=CARTESIAN_POINT('Ctrl Pts',(0.589962365403189,-1.,-2.09064881812053));
#27825=CARTESIAN_POINT('Ctrl Pts',(0.594585006052823,-1.,-2.09510876220501));
#27826=CARTESIAN_POINT('Ctrl Pts',(0.599241616422144,-1.,-2.09954930865331));
#27827=CARTESIAN_POINT('Ctrl Pts',(0.603932030738212,-1.,-2.10397049887709));
#27828=CARTESIAN_POINT('Ctrl Pts',(0.607711315456826,-1.,-2.10749199615859));
#27829=CARTESIAN_POINT('Ctrl Pts',(0.610560911691113,-1.,-2.11012443807661));
#27830=CARTESIAN_POINT('Ctrl Pts',(0.61246736556225,-1.,-2.11187554260142));
#27831=CARTESIAN_POINT('Ctrl Pts',(0.61342227326009,-1.,-2.11275013067528));
#27832=CARTESIAN_POINT('',(0.745574324794401,-1.,-2.0698113262342));
#27833=CARTESIAN_POINT('',(0.61342227326009,-1.,-2.11275013067528));
#27834=CARTESIAN_POINT('',(0.693717979106306,-1.,-1.60662857109684));
#27835=CARTESIAN_POINT('Ctrl Pts',(0.745574324794401,-1.,-2.0698113262342));
#27836=CARTESIAN_POINT('Ctrl Pts',(0.74583279137781,-1.,-2.06854248895575));
#27837=CARTESIAN_POINT('Ctrl Pts',(0.746345871542695,-1.,-2.06600523016401));
#27838=CARTESIAN_POINT('Ctrl Pts',(0.747103932785504,-1.,-2.06220058927162));
#27839=CARTESIAN_POINT('Ctrl Pts',(0.748091554181101,-1.,-2.05713023030263));
#27840=CARTESIAN_POINT('Ctrl Pts',(0.749287468663053,-1.,-2.05079645591606));
#27841=CARTESIAN_POINT('Ctrl Pts',(0.750444657874758,-1.,-2.04446689147754));
#27842=CARTESIAN_POINT('Ctrl Pts',(0.751562963361383,-1.,-2.03814160092173));
#27843=CARTESIAN_POINT('Ctrl Pts',(0.752642180488104,-1.,-2.03182068456467));
#27844=CARTESIAN_POINT('Ctrl Pts',(0.753682061113765,-1.,-2.02550428623587));
#27845=CARTESIAN_POINT('Ctrl Pts',(0.75468233072352,-1.,-2.01919259406003));
#27846=CARTESIAN_POINT('Ctrl Pts',(0.7556427049581,-1.,-2.01288584328149));
#27847=CARTESIAN_POINT('Ctrl Pts',(0.756562904646496,-1.,-2.00658431587682));
#27848=CARTESIAN_POINT('Ctrl Pts',(0.757442676862341,-1.,-2.00028834739072));
#27849=CARTESIAN_POINT('Ctrl Pts',(0.758281796766377,-1.,-1.9939983109871));
#27850=CARTESIAN_POINT('Ctrl Pts',(0.759080037802242,-1.,-1.98771456680806));
#27851=CARTESIAN_POINT('Ctrl Pts',(0.759837147452135,-1.,-1.98143741418156));
#27852=CARTESIAN_POINT('Ctrl Pts',(0.760552825409855,-1.,-1.97516705321521));
#27853=CARTESIAN_POINT('Ctrl Pts',(0.761226690483986,-1.,-1.96890351582545));
#27854=CARTESIAN_POINT('Ctrl Pts',(0.761858300014575,-1.,-1.96264672744229));
#27855=CARTESIAN_POINT('Ctrl Pts',(0.762447203806263,-1.,-1.95639665309893));
#27856=CARTESIAN_POINT('Ctrl Pts',(0.762992990878774,-1.,-1.95015342590025));
#27857=CARTESIAN_POINT('Ctrl Pts',(0.76349533353858,-1.,-1.94391746617626));
#27858=CARTESIAN_POINT('Ctrl Pts',(0.763954049121393,-1.,-1.93768964875867));
#27859=CARTESIAN_POINT('Ctrl Pts',(0.764369010673889,-1.,-1.93147105496367));
#27860=CARTESIAN_POINT('Ctrl Pts',(0.764740025488189,-1.,-1.92526263537041));
#27861=CARTESIAN_POINT('Ctrl Pts',(0.765066729667095,-1.,-1.91906491634197));
#27862=CARTESIAN_POINT('Ctrl Pts',(0.765348465884739,-1.,-1.91287765805174));
#27863=CARTESIAN_POINT('Ctrl Pts',(0.765584196937936,-1.,-1.90669961402362));
#27864=CARTESIAN_POINT('Ctrl Pts',(0.765772772593395,-1.,-1.90052930393599));
#27865=CARTESIAN_POINT('Ctrl Pts',(0.765913193856979,-1.,-1.89436577771389));
#27866=CARTESIAN_POINT('Ctrl Pts',(0.76600483706209,-1.,-1.88820926433409));
#27867=CARTESIAN_POINT('Ctrl Pts',(0.766047794851868,-1.,-1.88206215302561));
#27868=CARTESIAN_POINT('Ctrl Pts',(0.766042837036759,-1.,-1.87592888967886));
#27869=CARTESIAN_POINT('Ctrl Pts',(0.765990708546111,-1.,-1.86981398314345));
#27870=CARTESIAN_POINT('Ctrl Pts',(0.765891519092557,-1.,-1.86372027063315));
#27871=CARTESIAN_POINT('Ctrl Pts',(0.765744212909305,-1.,-1.85764741390391));
#27872=CARTESIAN_POINT('Ctrl Pts',(0.765545710619023,-1.,-1.85158945130054));
#27873=CARTESIAN_POINT('Ctrl Pts',(0.765291664861971,-1.,-1.84553698875911));
#27874=CARTESIAN_POINT('Ctrl Pts',(0.764978057881687,-1.,-1.83948181064823));
#27875=CARTESIAN_POINT('Ctrl Pts',(0.764602549687845,-1.,-1.8334207722714));
#27876=CARTESIAN_POINT('Ctrl Pts',(0.764165902606055,-1.,-1.8273599120008));
#27877=CARTESIAN_POINT('Ctrl Pts',(0.763673465462854,-1.,-1.82131873145297));
#27878=CARTESIAN_POINT('Ctrl Pts',(0.763132003836783,-1.,-1.81532118405566));
#27879=CARTESIAN_POINT('Ctrl Pts',(0.762546129464036,-1.,-1.80938551463989));
#27880=CARTESIAN_POINT('Ctrl Pts',(0.761915336443515,-1.,-1.80351583877334));
#27881=CARTESIAN_POINT('Ctrl Pts',(0.761229695230359,-1.,-1.79768986997735));
#27882=CARTESIAN_POINT('Ctrl Pts',(0.760469555880425,-1.,-1.79185815610802));
#27883=CARTESIAN_POINT('Ctrl Pts',(0.759614401109868,-1.,-1.78596964884527));
#27884=CARTESIAN_POINT('Ctrl Pts',(0.75865062667738,-1.,-1.77999411220912));
#27885=CARTESIAN_POINT('Ctrl Pts',(0.757578264077238,-1.,-1.77394167108342));
#27886=CARTESIAN_POINT('Ctrl Pts',(0.756421896028403,-1.,-1.76789396003141));
#27887=CARTESIAN_POINT('Ctrl Pts',(0.755220979975262,-1.,-1.7619781724032));
#27888=CARTESIAN_POINT('Ctrl Pts',(0.75400925402848,-1.,-1.75631083600175));
#27889=CARTESIAN_POINT('Ctrl Pts',(0.752797683531377,-1.,-1.75095139468809));
#27890=CARTESIAN_POINT('Ctrl Pts',(0.751555614163629,-1.,-1.74585086852298));
#27891=CARTESIAN_POINT('Ctrl Pts',(0.75019343597954,-1.,-1.74080458266705));
#27892=CARTESIAN_POINT('Ctrl Pts',(0.748582462954854,-1.,-1.73550351679848));
#27893=CARTESIAN_POINT('Ctrl Pts',(0.746574710096436,-1.,-1.72958533647399));
#27894=CARTESIAN_POINT('Ctrl Pts',(0.744021445433764,-1.,-1.7226822991693));
#27895=CARTESIAN_POINT('Ctrl Pts',(0.740795162032087,-1.,-1.71447789751927));
#27896=CARTESIAN_POINT('Ctrl Pts',(0.736799665724771,-1.,-1.70473309006121));
#27897=CARTESIAN_POINT('Ctrl Pts',(0.731963238697195,-1.,-1.69326921975743));
#27898=CARTESIAN_POINT('Ctrl Pts',(0.726235967997433,-1.,-1.67996158455503));
#27899=CARTESIAN_POINT('Ctrl Pts',(0.719585433804282,-1.,-1.6647288055568));
#27900=CARTESIAN_POINT('Ctrl Pts',(0.711993139355394,-1.,-1.64752408832016));
#27901=CARTESIAN_POINT('Ctrl Pts',(0.705159151988319,-1.,-1.63216541664676));
#27902=CARTESIAN_POINT('Ctrl Pts',(0.699605146405088,-1.,-1.61974673472612));
#27903=CARTESIAN_POINT('Ctrl Pts',(0.695712097881194,-1.,-1.61106790958151));
#27904=CARTESIAN_POINT('Ctrl Pts',(0.693717979106306,-1.,-1.60662857109684));
#27905=CARTESIAN_POINT('',(0.892032620296855,-1.,-1.5055822144029));
#27906=CARTESIAN_POINT('Origin',(0.,-1.,0.));
#27907=CARTESIAN_POINT('',(1.23627494547115,-1.,-1.81978687191668));
#27908=CARTESIAN_POINT('Ctrl Pts',(0.892032620296855,-1.,-1.5055822144029));
#27909=CARTESIAN_POINT('Ctrl Pts',(0.894452006964543,-1.,-1.50980486806688));
#27910=CARTESIAN_POINT('Ctrl Pts',(0.89918504748351,-1.,-1.51805569590094));
#27911=CARTESIAN_POINT('Ctrl Pts',(0.905967409625651,-1.,-1.52984849887993));
#27912=CARTESIAN_POINT('Ctrl Pts',(0.914375919026456,-1.,-1.54440491149498));
#27913=CARTESIAN_POINT('Ctrl Pts',(0.923832188944341,-1.,-1.56065988578893));
#27914=CARTESIAN_POINT('Ctrl Pts',(0.932246680108685,-1.,-1.57499388382243));
#27915=CARTESIAN_POINT('Ctrl Pts',(0.939646377893399,-1.,-1.58744937487176));
#27916=CARTESIAN_POINT('Ctrl Pts',(0.946078063315257,-1.,-1.59810042043673));
#27917=CARTESIAN_POINT('Ctrl Pts',(0.951613284356035,-1.,-1.60706069896936));
#27918=CARTESIAN_POINT('Ctrl Pts',(0.95635442292067,-1.,-1.61449324337085));
#27919=CARTESIAN_POINT('Ctrl Pts',(0.960438326101728,-1.,-1.62061638140221));
#27920=CARTESIAN_POINT('Ctrl Pts',(0.964046107040535,-1.,-1.62571930670187));
#27921=CARTESIAN_POINT('Ctrl Pts',(0.967387853230345,-1.,-1.63013849959462));
#27922=CARTESIAN_POINT('Ctrl Pts',(0.970669715997509,-1.,-1.63420665729798));
#27923=CARTESIAN_POINT('Ctrl Pts',(0.974066058287418,-1.,-1.63820952658144));
#27924=CARTESIAN_POINT('Ctrl Pts',(0.977689794119416,-1.,-1.64233990826687));
#27925=CARTESIAN_POINT('Ctrl Pts',(0.981562530939489,-1.,-1.64665139190656));
#27926=CARTESIAN_POINT('Ctrl Pts',(0.98564262292082,-1.,-1.65110016612638));
#27927=CARTESIAN_POINT('Ctrl Pts',(0.989855627854164,-1.,-1.65559044289699));
#27928=CARTESIAN_POINT('Ctrl Pts',(0.994121836661305,-1.,-1.66001553809947));
#27929=CARTESIAN_POINT('Ctrl Pts',(0.998389654952757,-1.,-1.66430758030376));
#27930=CARTESIAN_POINT('Ctrl Pts',(1.00265091003727,-1.,-1.66846059277303));
#27931=CARTESIAN_POINT('Ctrl Pts',(1.00692206696414,-1.,-1.67250335383293));
#27932=CARTESIAN_POINT('Ctrl Pts',(1.01123236493511,-1.,-1.67648246776464));
#27933=CARTESIAN_POINT('Ctrl Pts',(1.01561026162773,-1.,-1.68044289894798));
#27934=CARTESIAN_POINT('Ctrl Pts',(1.02006795074201,-1.,-1.68440578021706));
#27935=CARTESIAN_POINT('Ctrl Pts',(1.02460180535255,-1.,-1.68836910178447));
#27936=CARTESIAN_POINT('Ctrl Pts',(1.02919977579147,-1.,-1.69231840863458));
#27937=CARTESIAN_POINT('Ctrl Pts',(1.03384646003588,-1.,-1.69623414782771));
#27938=CARTESIAN_POINT('Ctrl Pts',(1.03852922490789,-1.,-1.70010052930962));
#27939=CARTESIAN_POINT('Ctrl Pts',(1.04324363334554,-1.,-1.70391338707982));
#27940=CARTESIAN_POINT('Ctrl Pts',(1.04799085404995,-1.,-1.70767646263649));
#27941=CARTESIAN_POINT('Ctrl Pts',(1.05277517202855,-1.,-1.71139783543989));
#27942=CARTESIAN_POINT('Ctrl Pts',(1.05760163192479,-1.,-1.7150865442702));
#27943=CARTESIAN_POINT('Ctrl Pts',(1.06247324680647,-1.,-1.71874858456904));
#27944=CARTESIAN_POINT('Ctrl Pts',(1.06738966975462,-1.,-1.72238500928453));
#27945=CARTESIAN_POINT('Ctrl Pts',(1.07234866990252,-1.,-1.72599406198488));
#27946=CARTESIAN_POINT('Ctrl Pts',(1.0773470373727,-1.,-1.72957248977424));
#27947=CARTESIAN_POINT('Ctrl Pts',(1.08238162784749,-1.,-1.73311705663407));
#27948=CARTESIAN_POINT('Ctrl Pts',(1.08745056285427,-1.,-1.73662628326091));
#27949=CARTESIAN_POINT('Ctrl Pts',(1.09255329056493,-1.,-1.74010053962247));
#27950=CARTESIAN_POINT('Ctrl Pts',(1.09768999241225,-1.,-1.74354119236208));
#27951=CARTESIAN_POINT('Ctrl Pts',(1.10286118991143,-1.,-1.74695004214923));
#27952=CARTESIAN_POINT('Ctrl Pts',(1.10806728183007,-1.,-1.7503286607592));
#27953=CARTESIAN_POINT('Ctrl Pts',(1.11330807582551,-1.,-1.7536777209463));
#27954=CARTESIAN_POINT('Ctrl Pts',(1.11858293216763,-1.,-1.75699720772105));
#27955=CARTESIAN_POINT('Ctrl Pts',(1.12389096855086,-1.,-1.76028671825096));
#27956=CARTESIAN_POINT('Ctrl Pts',(1.12923123555075,-1.,-1.7635457196617));
#27957=CARTESIAN_POINT('Ctrl Pts',(1.1346029180462,-1.,-1.76677384551862));
#27958=CARTESIAN_POINT('Ctrl Pts',(1.14000548336975,-1.,-1.76997111386769));
#27959=CARTESIAN_POINT('Ctrl Pts',(1.1454385822692,-1.,-1.77313777896194));
#27960=CARTESIAN_POINT('Ctrl Pts',(1.15090197841514,-1.,-1.7762742255701));
#27961=CARTESIAN_POINT('Ctrl Pts',(1.15639547194698,-1.,-1.77938085564275));
#27962=CARTESIAN_POINT('Ctrl Pts',(1.16191881298499,-1.,-1.78245795881009));
#27963=CARTESIAN_POINT('Ctrl Pts',(1.16747166312303,-1.,-1.78550566040443));
#27964=CARTESIAN_POINT('Ctrl Pts',(1.17305363177328,-1.,-1.78852398877617));
#27965=CARTESIAN_POINT('Ctrl Pts',(1.17866429440809,-1.,-1.79151291552689));
#27966=CARTESIAN_POINT('Ctrl Pts',(1.18430321697432,-1.,-1.79447240321515));
#27967=CARTESIAN_POINT('Ctrl Pts',(1.18996997934445,-1.,-1.79740245923478));
#27968=CARTESIAN_POINT('Ctrl Pts',(1.19566418930242,-1.,-1.80030314369879));
#27969=CARTESIAN_POINT('Ctrl Pts',(1.20138548938974,-1.,-1.80317454838603));
#27970=CARTESIAN_POINT('Ctrl Pts',(1.20713356605475,-1.,-1.80601678480707));
#27971=CARTESIAN_POINT('Ctrl Pts',(1.21290815708314,-1.,-1.80882996917129));
#27972=CARTESIAN_POINT('Ctrl Pts',(1.21870906103557,-1.,-1.81161420806656));
#27973=CARTESIAN_POINT('Ctrl Pts',(1.2245361330495,-1.,-1.81436959210434));
#27974=CARTESIAN_POINT('Ctrl Pts',(1.2292186489137,-1.,-1.8165508718364));
#27975=CARTESIAN_POINT('Ctrl Pts',(1.2327422452705,-1.,-1.81817389921279));
#27976=CARTESIAN_POINT('Ctrl Pts',(1.23509651170476,-1.,-1.81925017193666));
#27977=CARTESIAN_POINT('Ctrl Pts',(1.23627494547115,-1.,-1.81978687191668));
#27978=CARTESIAN_POINT('',(1.34869019493419,-1.,-1.73811241238545));
#27979=CARTESIAN_POINT('',(1.23627494547115,-1.,-1.81978687191668));
#27980=CARTESIAN_POINT('',(1.15624053661742,-1.,-1.31362392696032));
#27981=CARTESIAN_POINT('Ctrl Pts',(1.34869019493419,-1.,-1.73811241238545));
#27982=CARTESIAN_POINT('Ctrl Pts',(1.34854391898045,-1.,-1.73682580585691));
#27983=CARTESIAN_POINT('Ctrl Pts',(1.34824783112887,-1.,-1.73425417885907));
#27984=CARTESIAN_POINT('Ctrl Pts',(1.34779309152035,-1.,-1.7304014965394));
#27985=CARTESIAN_POINT('Ctrl Pts',(1.34716554819527,-1.,-1.72527410680674));
#27986=CARTESIAN_POINT('Ctrl Pts',(1.34634568653227,-1.,-1.7188807715049));
#27987=CARTESIAN_POINT('Ctrl Pts',(1.34549029589416,-1.,-1.71250340686822));
#27988=CARTESIAN_POINT('Ctrl Pts',(1.34459924533831,-1.,-1.70614212266738));
#27989=CARTESIAN_POINT('Ctrl Pts',(1.34367237124483,-1.,-1.69979707754427));
#27990=CARTESIAN_POINT('Ctrl Pts',(1.34270948206319,-1.,-1.6934684849687));
#27991=CARTESIAN_POINT('Ctrl Pts',(1.341710374848,-1.,-1.68715660868764));
#27992=CARTESIAN_POINT('Ctrl Pts',(1.34067485185203,-1.,-1.68086176030362));
#27993=CARTESIAN_POINT('Ctrl Pts',(1.3396027347034,-1.,-1.67458429426086));
#27994=CARTESIAN_POINT('Ctrl Pts',(1.33849388654388,-1.,-1.66832460783989));
#27995=CARTESIAN_POINT('Ctrl Pts',(1.33734820885262,-1.,-1.66208312541983));
#27996=CARTESIAN_POINT('Ctrl Pts',(1.33616559745172,-1.,-1.65586025952593));
#27997=CARTESIAN_POINT('Ctrl Pts',(1.33494590467993,-1.,-1.6496563728683));
#27998=CARTESIAN_POINT('Ctrl Pts',(1.33368890676572,-1.,-1.6434717485603));
#27999=CARTESIAN_POINT('Ctrl Pts',(1.33239425103724,-1.,-1.63730653475089));
#28000=CARTESIAN_POINT('Ctrl Pts',(1.33106149345645,-1.,-1.63116079730923));
#28001=CARTESIAN_POINT('Ctrl Pts',(1.3296901950568,-1.,-1.62503464209797));
#28002=CARTESIAN_POINT('Ctrl Pts',(1.32828000610449,-1.,-1.61892832270724));
#28003=CARTESIAN_POINT('Ctrl Pts',(1.32683074483356,-1.,-1.6128423401575));
#28004=CARTESIAN_POINT('Ctrl Pts',(1.32534250785782,-1.,-1.60677758290954));
#28005=CARTESIAN_POINT('Ctrl Pts',(1.32381550858256,-1.,-1.60073511858687));
#28006=CARTESIAN_POINT('Ctrl Pts',(1.32224985747682,-1.,-1.59471591079403));
#28007=CARTESIAN_POINT('Ctrl Pts',(1.32064537110892,-1.,-1.58872057258245));
#28008=CARTESIAN_POINT('Ctrl Pts',(1.31900135021432,-1.,-1.58274907898834));
#28009=CARTESIAN_POINT('Ctrl Pts',(1.31731642317187,-1.,-1.5768005650559));
#28010=CARTESIAN_POINT('Ctrl Pts',(1.31558903860016,-1.,-1.57087397835723));
#28011=CARTESIAN_POINT('Ctrl Pts',(1.31381795281002,-1.,-1.56496872402353));
#28012=CARTESIAN_POINT('Ctrl Pts',(1.31200264341696,-1.,-1.55908521254821));
#28013=CARTESIAN_POINT('Ctrl Pts',(1.31014393684222,-1.,-1.55322568759481));
#28014=CARTESIAN_POINT('Ctrl Pts',(1.30824393907473,-1.,-1.54739413957185));
#28015=CARTESIAN_POINT('Ctrl Pts',(1.30630475189556,-1.,-1.54159462645432));
#28016=CARTESIAN_POINT('Ctrl Pts',(1.30432735639489,-1.,-1.53582981268977));
#28017=CARTESIAN_POINT('Ctrl Pts',(1.30231064395568,-1.,-1.53009970283891));
#28018=CARTESIAN_POINT('Ctrl Pts',(1.30024984366328,-1.,-1.52439957861062));
#28019=CARTESIAN_POINT('Ctrl Pts',(1.29813791800747,-1.,-1.51872184912724));
#28020=CARTESIAN_POINT('Ctrl Pts',(1.29596850710509,-1.,-1.51305994241402));
#28021=CARTESIAN_POINT('Ctrl Pts',(1.29373841372842,-1.,-1.50741159078365));
#28022=CARTESIAN_POINT('Ctrl Pts',(1.29145022885181,-1.,-1.50178230149776));
#28023=CARTESIAN_POINT('Ctrl Pts',(1.28911506584254,-1.,-1.49618896881754));
#28024=CARTESIAN_POINT('Ctrl Pts',(1.2867467611644,-1.,-1.4906522831278));
#28025=CARTESIAN_POINT('Ctrl Pts',(1.28435533880201,-1.,-1.4851881711891));
#28026=CARTESIAN_POINT('Ctrl Pts',(1.28194158939517,-1.,-1.47980070347096));
#28027=CARTESIAN_POINT('Ctrl Pts',(1.2794891824849,-1.,-1.4744717526707));
#28028=CARTESIAN_POINT('Ctrl Pts',(1.27696414831089,-1.,-1.46916035917133));
#28029=CARTESIAN_POINT('Ctrl Pts',(1.27433119897822,-1.,-1.46382431332476));
#28030=CARTESIAN_POINT('Ctrl Pts',(1.27156805265289,-1.,-1.45843906294697));
#28031=CARTESIAN_POINT('Ctrl Pts',(1.2686778680489,-1.,-1.45301422764247));
#28032=CARTESIAN_POINT('Ctrl Pts',(1.26570925118868,-1.,-1.44761985001662));
#28033=CARTESIAN_POINT('Ctrl Pts',(1.26273903323858,-1.,-1.44236470511303));
#28034=CARTESIAN_POINT('Ctrl Pts',(1.25983531012005,-1.,-1.43734919180848));
#28035=CARTESIAN_POINT('Ctrl Pts',(1.25702687965755,-1.,-1.43262645609691));
#28036=CARTESIAN_POINT('Ctrl Pts',(1.25426945222639,-1.,-1.42815938799387));
#28037=CARTESIAN_POINT('Ctrl Pts',(1.2514145557001,-1.,-1.42378102115575));
#28038=CARTESIAN_POINT('Ctrl Pts',(1.24824430986571,-1.,-1.41923722596025));
#28039=CARTESIAN_POINT('Ctrl Pts',(1.24450600513056,-1.,-1.41422913175179));
#28040=CARTESIAN_POINT('Ctrl Pts',(1.23994455029534,-1.,-1.40845295531283));
#28041=CARTESIAN_POINT('Ctrl Pts',(1.23434087290423,-1.,-1.40164708206106));
#28042=CARTESIAN_POINT('Ctrl Pts',(1.22752961899387,-1.,-1.39361389568796));
#28043=CARTESIAN_POINT('Ctrl Pts',(1.21938737280852,-1.,-1.38420564527715));
#28044=CARTESIAN_POINT('Ctrl Pts',(1.20982812925645,-1.,-1.37331915607905));
#28045=CARTESIAN_POINT('Ctrl Pts',(1.1987959077932,-1.,-1.36088705043885));
#28046=CARTESIAN_POINT('Ctrl Pts',(1.18625865667441,-1.,-1.34687054001093));
#28047=CARTESIAN_POINT('Ctrl Pts',(1.17501305789857,-1.,-1.33437539347008));
#28048=CARTESIAN_POINT('Ctrl Pts',(1.16589330093588,-1.,-1.32428080721772));
#28049=CARTESIAN_POINT('Ctrl Pts',(1.15950888730809,-1.,-1.31722977216397));
#28050=CARTESIAN_POINT('Ctrl Pts',(1.15624053661742,-1.,-1.31362392696032));
#28051=CARTESIAN_POINT('',(1.31362392696032,-1.,-1.15624053661742));
#28052=CARTESIAN_POINT('Origin',(0.,-1.,0.));
#28053=CARTESIAN_POINT('',(1.73811241238545,-1.,-1.34869019493419));
#28054=CARTESIAN_POINT('Ctrl Pts',(1.31362392696032,-1.,-1.15624053661742));
#28055=CARTESIAN_POINT('Ctrl Pts',(1.3172297721596,-1.,-1.15950888730433));
#28056=CARTESIAN_POINT('Ctrl Pts',(1.32428080720544,-1.,-1.16589330092532));
#28057=CARTESIAN_POINT('Ctrl Pts',(1.33437539344842,-1.,-1.17501305787994));
#28058=CARTESIAN_POINT('Ctrl Pts',(1.34687053998157,-1.,-1.18625865664915));
#28059=CARTESIAN_POINT('Ctrl Pts',(1.36088705040677,-1.,-1.1987959077656));
#28060=CARTESIAN_POINT('Ctrl Pts',(1.37331915604962,-1.,-1.20982812923113));
#28061=CARTESIAN_POINT('Ctrl Pts',(1.38420564525391,-1.,-1.21938737278853));
#28062=CARTESIAN_POINT('Ctrl Pts',(1.39361389567257,-1.,-1.22752961898063));
#28063=CARTESIAN_POINT('Ctrl Pts',(1.40164708205345,-1.,-1.23434087289768));
#28064=CARTESIAN_POINT('Ctrl Pts',(1.40845295531151,-1.,-1.23994455029421));
#28065=CARTESIAN_POINT('Ctrl Pts',(1.41422913175437,-1.,-1.24450600513278));
#28066=CARTESIAN_POINT('Ctrl Pts',(1.41923722596421,-1.,-1.24824430986911));
#28067=CARTESIAN_POINT('Ctrl Pts',(1.42378102115911,-1.,-1.25141455570299));
#28068=CARTESIAN_POINT('Ctrl Pts',(1.42815938799555,-1.,-1.25426945222783));
#28069=CARTESIAN_POINT('Ctrl Pts',(1.43262645609679,-1.,-1.25702687965744));
#28070=CARTESIAN_POINT('Ctrl Pts',(1.43734919180719,-1.,-1.25983531011894));
#28071=CARTESIAN_POINT('Ctrl Pts',(1.44236470511145,-1.,-1.26273903323723));
#28072=CARTESIAN_POINT('Ctrl Pts',(1.44761985001544,-1.,-1.26570925118767));
#28073=CARTESIAN_POINT('Ctrl Pts',(1.45301422764205,-1.,-1.26867786804854));
#28074=CARTESIAN_POINT('Ctrl Pts',(1.45843906294725,-1.,-1.27156805265312));
#28075=CARTESIAN_POINT('Ctrl Pts',(1.4638243133254,-1.,-1.27433119897877));
#28076=CARTESIAN_POINT('Ctrl Pts',(1.46916035917197,-1.,-1.27696414831144));
#28077=CARTESIAN_POINT('Ctrl Pts',(1.4744717526711,-1.,-1.27948918248524));
#28078=CARTESIAN_POINT('Ctrl Pts',(1.47980070347102,-1.,-1.28194158939522));
#28079=CARTESIAN_POINT('Ctrl Pts',(1.48518817118891,-1.,-1.28435533880184));
#28080=CARTESIAN_POINT('Ctrl Pts',(1.4906522831275,-1.,-1.28674676116415));
#28081=CARTESIAN_POINT('Ctrl Pts',(1.49618896881729,-1.,-1.28911506584232));
#28082=CARTESIAN_POINT('Ctrl Pts',(1.50178230149764,-1.,-1.29145022885171));
#28083=CARTESIAN_POINT('Ctrl Pts',(1.50741159078367,-1.,-1.29373841372843));
#28084=CARTESIAN_POINT('Ctrl Pts',(1.51305994241412,-1.,-1.29596850710518));
#28085=CARTESIAN_POINT('Ctrl Pts',(1.51872184912735,-1.,-1.29813791800757));
#28086=CARTESIAN_POINT('Ctrl Pts',(1.5243995786107,-1.,-1.30024984366334));
#28087=CARTESIAN_POINT('Ctrl Pts',(1.53009970283893,-1.,-1.3023106439557));
#28088=CARTESIAN_POINT('Ctrl Pts',(1.53582981268976,-1.,-1.30432735639487));
#28089=CARTESIAN_POINT('Ctrl Pts',(1.54159462645428,-1.,-1.30630475189553));
#28090=CARTESIAN_POINT('Ctrl Pts',(1.54739413957183,-1.,-1.30824393907471));
#28091=CARTESIAN_POINT('Ctrl Pts',(1.55322568759481,-1.,-1.31014393684221));
#28092=CARTESIAN_POINT('Ctrl Pts',(1.55908521254822,-1.,-1.31200264341696));
#28093=CARTESIAN_POINT('Ctrl Pts',(1.56496872402352,-1.,-1.31381795281002));
#28094=CARTESIAN_POINT('Ctrl Pts',(1.57087397835721,-1.,-1.31558903860015));
#28095=CARTESIAN_POINT('Ctrl Pts',(1.57680056505585,-1.,-1.31731642317183));
#28096=CARTESIAN_POINT('Ctrl Pts',(1.58274907898829,-1.,-1.31900135021428));
#28097=CARTESIAN_POINT('Ctrl Pts',(1.58872057258244,-1.,-1.32064537110891));
#28098=CARTESIAN_POINT('Ctrl Pts',(1.59471591079408,-1.,-1.32224985747686));
#28099=CARTESIAN_POINT('Ctrl Pts',(1.600735118587,-1.,-1.32381550858266));
#28100=CARTESIAN_POINT('Ctrl Pts',(1.6067775829097,-1.,-1.32534250785794));
#28101=CARTESIAN_POINT('Ctrl Pts',(1.61284234015762,-1.,-1.32683074483365));
#28102=CARTESIAN_POINT('Ctrl Pts',(1.61892832270723,-1.,-1.32828000610448));
#28103=CARTESIAN_POINT('Ctrl Pts',(1.62503464209777,-1.,-1.32969019505665));
#28104=CARTESIAN_POINT('Ctrl Pts',(1.63116079730887,-1.,-1.33106149345618));
#28105=CARTESIAN_POINT('Ctrl Pts',(1.63730653475049,-1.,-1.33239425103694));
#28106=CARTESIAN_POINT('Ctrl Pts',(1.64347174856007,-1.,-1.33368890676554));
#28107=CARTESIAN_POINT('Ctrl Pts',(1.64965637286843,-1.,-1.33494590468003));
#28108=CARTESIAN_POINT('Ctrl Pts',(1.65586025952651,-1.,-1.33616559745217));
#28109=CARTESIAN_POINT('Ctrl Pts',(1.66208312542073,-1.,-1.33734820885331));
#28110=CARTESIAN_POINT('Ctrl Pts',(1.66832460784078,-1.,-1.33849388654458));
#28111=CARTESIAN_POINT('Ctrl Pts',(1.67458429426126,-1.,-1.33960273470372));
#28112=CARTESIAN_POINT('Ctrl Pts',(1.68086176030308,-1.,-1.3406748518516));
#28113=CARTESIAN_POINT('Ctrl Pts',(1.68715660868602,-1.,-1.34171037484673));
#28114=CARTESIAN_POINT('Ctrl Pts',(1.6934684849664,-1.,-1.34270948206139));
#28115=CARTESIAN_POINT('Ctrl Pts',(1.69979707754221,-1.,-1.34367237124322));
#28116=CARTESIAN_POINT('Ctrl Pts',(1.70614212266676,-1.,-1.34459924533783));
#28117=CARTESIAN_POINT('Ctrl Pts',(1.71250340687011,-1.,-1.34549029589563));
#28118=CARTESIAN_POINT('Ctrl Pts',(1.7188807715095,-1.,-1.34634568653586));
#28119=CARTESIAN_POINT('Ctrl Pts',(1.72527410681298,-1.,-1.34716554820013));
#28120=CARTESIAN_POINT('Ctrl Pts',(1.73040149654497,-1.,-1.3477930915247));
#28121=CARTESIAN_POINT('Ctrl Pts',(1.73425417886254,-1.,-1.34824783113158));
#28122=CARTESIAN_POINT('Ctrl Pts',(1.73682580585819,-1.,-1.34854391898145));
#28123=CARTESIAN_POINT('Ctrl Pts',(1.73811241238545,-1.,-1.34869019493419));
#28124=CARTESIAN_POINT('',(1.81978687191668,-1.,-1.23627494547115));
#28125=CARTESIAN_POINT('',(1.73811241238545,-1.,-1.34869019493419));
#28126=CARTESIAN_POINT('',(1.5055822144029,-1.,-0.892032620296855));
#28127=CARTESIAN_POINT('Ctrl Pts',(1.81978687191668,-1.,-1.23627494547115));
#28128=CARTESIAN_POINT('Ctrl Pts',(1.81925017193531,-1.,-1.23509651170384));
#28129=CARTESIAN_POINT('Ctrl Pts',(1.81817389920914,-1.,-1.23274224526804));
#28130=CARTESIAN_POINT('Ctrl Pts',(1.81655087183054,-1.,-1.22921864890975));
#28131=CARTESIAN_POINT('Ctrl Pts',(1.81436959209778,-1.,-1.22453613304507));
#28132=CARTESIAN_POINT('Ctrl Pts',(1.81161420806172,-1.,-1.2187090610323));
#28133=CARTESIAN_POINT('Ctrl Pts',(1.80882996916931,-1.,-1.2129081570818));
#28134=CARTESIAN_POINT('Ctrl Pts',(1.80601678480772,-1.,-1.20713356605519));
#28135=CARTESIAN_POINT('Ctrl Pts',(1.8031745483882,-1.,-1.2013854893912));
#28136=CARTESIAN_POINT('Ctrl Pts',(1.80030314370121,-1.,-1.19566418930405));
#28137=CARTESIAN_POINT('Ctrl Pts',(1.79740245923649,-1.,-1.1899699793456));
#28138=CARTESIAN_POINT('Ctrl Pts',(1.79447240321572,-1.,-1.18430321697471));
#28139=CARTESIAN_POINT('Ctrl Pts',(1.79151291552646,-1.,-1.17866429440781));
#28140=CARTESIAN_POINT('Ctrl Pts',(1.78852398877523,-1.,-1.17305363177265));
#28141=CARTESIAN_POINT('Ctrl Pts',(1.78550566040349,-1.,-1.16747166312239));
#28142=CARTESIAN_POINT('Ctrl Pts',(1.78245795880949,-1.,-1.16191881298458));
#28143=CARTESIAN_POINT('Ctrl Pts',(1.77938085564261,-1.,-1.15639547194689));
#28144=CARTESIAN_POINT('Ctrl Pts',(1.77627422557034,-1.,-1.15090197841531));
#28145=CARTESIAN_POINT('Ctrl Pts',(1.77313777896234,-1.,-1.14543858226948));
#28146=CARTESIAN_POINT('Ctrl Pts',(1.76997111386806,-1.,-1.14000548337));
#28147=CARTESIAN_POINT('Ctrl Pts',(1.76677384551883,-1.,-1.13460291804635));
#28148=CARTESIAN_POINT('Ctrl Pts',(1.76354571966171,-1.,-1.12923123555076));
#28149=CARTESIAN_POINT('Ctrl Pts',(1.76028671825084,-1.,-1.12389096855078));
#28150=CARTESIAN_POINT('Ctrl Pts',(1.75699720772089,-1.,-1.11858293216752));
#28151=CARTESIAN_POINT('Ctrl Pts',(1.75367772094617,-1.,-1.11330807582542));
#28152=CARTESIAN_POINT('Ctrl Pts',(1.75032866075914,-1.,-1.10806728183003));
#28153=CARTESIAN_POINT('Ctrl Pts',(1.74695004214924,-1.,-1.10286118991144));
#28154=CARTESIAN_POINT('Ctrl Pts',(1.74354119236212,-1.,-1.09768999241229));
#28155=CARTESIAN_POINT('Ctrl Pts',(1.74010053962252,-1.,-1.09255329056496));
#28156=CARTESIAN_POINT('Ctrl Pts',(1.73662628326093,-1.,-1.08745056285429));
#28157=CARTESIAN_POINT('Ctrl Pts',(1.73311705663407,-1.,-1.08238162784749));
#28158=CARTESIAN_POINT('Ctrl Pts',(1.72957248977424,-1.,-1.0773470373727));
#28159=CARTESIAN_POINT('Ctrl Pts',(1.72599406198489,-1.,-1.07234866990252));
#28160=CARTESIAN_POINT('Ctrl Pts',(1.72238500928456,-1.,-1.06738966975463));
#28161=CARTESIAN_POINT('Ctrl Pts',(1.71874858456908,-1.,-1.0624732468065));
#28162=CARTESIAN_POINT('Ctrl Pts',(1.71508654427022,-1.,-1.05760163192481));
#28163=CARTESIAN_POINT('Ctrl Pts',(1.71139783543986,-1.,-1.05277517202854));
#28164=CARTESIAN_POINT('Ctrl Pts',(1.70767646263641,-1.,-1.0479908540499));
#28165=CARTESIAN_POINT('Ctrl Pts',(1.70391338707969,-1.,-1.04324363334546));
#28166=CARTESIAN_POINT('Ctrl Pts',(1.70010052930951,-1.,-1.03852922490782));
#28167=CARTESIAN_POINT('Ctrl Pts',(1.69623414782769,-1.,-1.03384646003587));
#28168=CARTESIAN_POINT('Ctrl Pts',(1.69231840863471,-1.,-1.02919977579155));
#28169=CARTESIAN_POINT('Ctrl Pts',(1.68836910178475,-1.,-1.02460180535272));
#28170=CARTESIAN_POINT('Ctrl Pts',(1.68440578021739,-1.,-1.02006795074222));
#28171=CARTESIAN_POINT('Ctrl Pts',(1.6804428989482,-1.,-1.01561026162787));
#28172=CARTESIAN_POINT('Ctrl Pts',(1.67648246776457,-1.,-1.01123236493507));
#28173=CARTESIAN_POINT('Ctrl Pts',(1.67250335383248,-1.,-1.00692206696387));
#28174=CARTESIAN_POINT('Ctrl Pts',(1.66846059277231,-1.,-1.00265091003682));
#28175=CARTESIAN_POINT('Ctrl Pts',(1.66430758030304,-1.,-0.998389654952317));
#28176=CARTESIAN_POINT('Ctrl Pts',(1.66001553809916,-1.,-0.994121836661116));
#28177=CARTESIAN_POINT('Ctrl Pts',(1.65559044289746,-1.,-0.98985562785445));
#28178=CARTESIAN_POINT('Ctrl Pts',(1.6511001661277,-1.,-0.985642622921626));
#28179=CARTESIAN_POINT('Ctrl Pts',(1.64665139190834,-1.,-0.981562530940574));
#28180=CARTESIAN_POINT('Ctrl Pts',(1.64233990826831,-1.,-0.977689794120297));
#28181=CARTESIAN_POINT('Ctrl Pts',(1.63820952658157,-1.,-0.974066058287501));
#28182=CARTESIAN_POINT('Ctrl Pts',(1.63420665729609,-1.,-0.970669715996356));
#28183=CARTESIAN_POINT('Ctrl Pts',(1.63013849959083,-1.,-0.967387853228041));
#28184=CARTESIAN_POINT('Ctrl Pts',(1.6257193066974,-1.,-0.964046107037821));
#28185=CARTESIAN_POINT('Ctrl Pts',(1.62061638139929,-1.,-0.960438326099958));
#28186=CARTESIAN_POINT('Ctrl Pts',(1.61449324337233,-1.,-0.956354422921573));
#28187=CARTESIAN_POINT('Ctrl Pts',(1.60706069897794,-1.,-0.951613284361248));
#28188=CARTESIAN_POINT('Ctrl Pts',(1.59810042045408,-1.,-0.946078063325796));
#28189=CARTESIAN_POINT('Ctrl Pts',(1.58744937489796,-1.,-0.939646377909319));
#28190=CARTESIAN_POINT('Ctrl Pts',(1.57499388385561,-1.,-0.932246680128849));
#28191=CARTESIAN_POINT('Ctrl Pts',(1.56065988582509,-1.,-0.923832188966322));
#28192=CARTESIAN_POINT('Ctrl Pts',(1.54440491152807,-1.,-0.91437591904658));
#28193=CARTESIAN_POINT('Ctrl Pts',(1.52984849890434,-1.,-0.905967409640499));
#28194=CARTESIAN_POINT('Ctrl Pts',(1.51805569591479,-1.,-0.89918504749193));
#28195=CARTESIAN_POINT('Ctrl Pts',(1.50980486807181,-1.,-0.894452006967538));
#28196=CARTESIAN_POINT('Ctrl Pts',(1.5055822144029,-1.,-0.892032620296855));
#28197=CARTESIAN_POINT('',(1.60662857109684,-1.,-0.693717979106306));
#28198=CARTESIAN_POINT('Origin',(0.,-1.,0.));
#28199=CARTESIAN_POINT('',(2.0698113262342,-1.,-0.745574324794401));
#28200=CARTESIAN_POINT('Ctrl Pts',(1.60662857109684,-1.,-0.693717979106306));
#28201=CARTESIAN_POINT('Ctrl Pts',(1.61106790957619,-1.,-0.69571209787897));
#28202=CARTESIAN_POINT('Ctrl Pts',(1.61974673471117,-1.,-0.699605146398837));
#28203=CARTESIAN_POINT('Ctrl Pts',(1.6321654166204,-1.,-0.705159151977294));
#28204=CARTESIAN_POINT('Ctrl Pts',(1.64752408828442,-1.,-0.711993139340448));
#28205=CARTESIAN_POINT('Ctrl Pts',(1.66472880551777,-1.,-0.71958543378795));
#28206=CARTESIAN_POINT('Ctrl Pts',(1.67996158451922,-1.,-0.726235967982445));
#28207=CARTESIAN_POINT('Ctrl Pts',(1.69326921972915,-1.,-0.731963238685357));
#28208=CARTESIAN_POINT('Ctrl Pts',(1.70473309004249,-1.,-0.736799665716932));
#28209=CARTESIAN_POINT('Ctrl Pts',(1.71447789751001,-1.,-0.74079516202821));
#28210=CARTESIAN_POINT('Ctrl Pts',(1.72268229916769,-1.,-0.744021445433094));
#28211=CARTESIAN_POINT('Ctrl Pts',(1.72958533647714,-1.,-0.746574710097752));
#28212=CARTESIAN_POINT('Ctrl Pts',(1.7355035168033,-1.,-0.74858246295687));
#28213=CARTESIAN_POINT('Ctrl Pts',(1.74080458267114,-1.,-0.75019343598125));
#28214=CARTESIAN_POINT('Ctrl Pts',(1.74585086852502,-1.,-0.751555614164483));
#28215=CARTESIAN_POINT('Ctrl Pts',(1.75095139468794,-1.,-0.752797683531314));
#28216=CARTESIAN_POINT('Ctrl Pts',(1.75631083600019,-1.,-0.754009254027829));
#28217=CARTESIAN_POINT('Ctrl Pts',(1.76197817240128,-1.,-0.755220979974462));
#28218=CARTESIAN_POINT('Ctrl Pts',(1.76789396002998,-1.,-0.75642189602781));
#28219=CARTESIAN_POINT('Ctrl Pts',(1.77394167108292,-1.,-0.757578264077029));
#28220=CARTESIAN_POINT('Ctrl Pts',(1.77999411220945,-1.,-0.758650626677519));
#28221=CARTESIAN_POINT('Ctrl Pts',(1.78596964884604,-1.,-0.75961440111019));
#28222=CARTESIAN_POINT('Ctrl Pts',(1.7918581561088,-1.,-0.760469555880749));
#28223=CARTESIAN_POINT('Ctrl Pts',(1.79768986997783,-1.,-0.761229695230558));
#28224=CARTESIAN_POINT('Ctrl Pts',(1.80351583877342,-1.,-0.761915336443547));
#28225=CARTESIAN_POINT('Ctrl Pts',(1.80938551463965,-1.,-0.762546129463938));
#28226=CARTESIAN_POINT('Ctrl Pts',(1.8153211840553,-1.,-0.763132003836634));
#28227=CARTESIAN_POINT('Ctrl Pts',(1.82131873145266,-1.,-0.763673465462727));
#28228=CARTESIAN_POINT('Ctrl Pts',(1.82735991200065,-1.,-0.764165902605995));
#28229=CARTESIAN_POINT('Ctrl Pts',(1.83342077227142,-1.,-0.764602549687853));
#28230=CARTESIAN_POINT('Ctrl Pts',(1.83948181064835,-1.,-0.764978057881738));
#28231=CARTESIAN_POINT('Ctrl Pts',(1.84553698875924,-1.,-0.765291664862029));
#28232=CARTESIAN_POINT('Ctrl Pts',(1.85158945130063,-1.,-0.765545710619063));
#28233=CARTESIAN_POINT('Ctrl Pts',(1.85764741390394,-1.,-0.765744212909319));
#28234=CARTESIAN_POINT('Ctrl Pts',(1.86372027063312,-1.,-0.765891519092547));
#28235=CARTESIAN_POINT('Ctrl Pts',(1.86981398314341,-1.,-0.765990708546091));
#28236=CARTESIAN_POINT('Ctrl Pts',(1.87592888967883,-1.,-0.766042837036744));
#28237=CARTESIAN_POINT('Ctrl Pts',(1.88206215302561,-1.,-0.766047794851865));
#28238=CARTESIAN_POINT('Ctrl Pts',(1.88820926433409,-1.,-0.766004837062091));
#28239=CARTESIAN_POINT('Ctrl Pts',(1.89436577771388,-1.,-0.765913193856978));
#28240=CARTESIAN_POINT('Ctrl Pts',(1.90052930393596,-1.,-0.765772772593386));
#28241=CARTESIAN_POINT('Ctrl Pts',(1.90669961402356,-1.,-0.765584196937919));
#28242=CARTESIAN_POINT('Ctrl Pts',(1.91287765805169,-1.,-0.765348465884722));
#28243=CARTESIAN_POINT('Ctrl Pts',(1.91906491634196,-1.,-0.765066729667089));
#28244=CARTESIAN_POINT('Ctrl Pts',(1.92526263537048,-1.,-0.764740025488212));
#28245=CARTESIAN_POINT('Ctrl Pts',(1.93147105496382,-1.,-0.764369010673941));
#28246=CARTESIAN_POINT('Ctrl Pts',(1.93768964875886,-1.,-0.763954049121459));
#28247=CARTESIAN_POINT('Ctrl Pts',(1.9439174661764,-1.,-0.763495333538629));
#28248=CARTESIAN_POINT('Ctrl Pts',(1.95015342590024,-1.,-0.762992990878769));
#28249=CARTESIAN_POINT('Ctrl Pts',(1.95639665309869,-1.,-0.762447203806179));
#28250=CARTESIAN_POINT('Ctrl Pts',(1.96264672744186,-1.,-0.761858300014424));
#28251=CARTESIAN_POINT('Ctrl Pts',(1.96890351582499,-1.,-0.761226690483821));
#28252=CARTESIAN_POINT('Ctrl Pts',(1.97516705321494,-1.,-0.760552825409757));
#28253=CARTESIAN_POINT('Ctrl Pts',(1.98143741418172,-1.,-0.75983714745219));
#28254=CARTESIAN_POINT('Ctrl Pts',(1.98771456680874,-1.,-0.759080037802488));
#28255=CARTESIAN_POINT('Ctrl Pts',(1.99399831098817,-1.,-0.758281796766761));
#28256=CARTESIAN_POINT('Ctrl Pts',(2.00028834739178,-1.,-0.757442676862724));
#28257=CARTESIAN_POINT('Ctrl Pts',(2.0065843158773,-1.,-0.756562904646671));
#28258=CARTESIAN_POINT('Ctrl Pts',(2.01288584328084,-1.,-0.755642704957865));
#28259=CARTESIAN_POINT('Ctrl Pts',(2.01919259405809,-1.,-0.754682330722816));
#28260=CARTESIAN_POINT('Ctrl Pts',(2.02550428623313,-1.,-0.753682061112768));
#28261=CARTESIAN_POINT('Ctrl Pts',(2.03182068456221,-1.,-0.752642180487211));
#28262=CARTESIAN_POINT('Ctrl Pts',(2.03814160092099,-1.,-0.751562963361115));
#28263=CARTESIAN_POINT('Ctrl Pts',(2.04446689147979,-1.,-0.750444657875576));
#28264=CARTESIAN_POINT('Ctrl Pts',(2.05079645592154,-1.,-0.749287468665046));
#28265=CARTESIAN_POINT('Ctrl Pts',(2.05713023031006,-1.,-0.748091554183803));
#28266=CARTESIAN_POINT('Ctrl Pts',(2.06220058927826,-1.,-0.74710393278792));
#28267=CARTESIAN_POINT('Ctrl Pts',(2.06600523016815,-1.,-0.746345871544201));
#28268=CARTESIAN_POINT('Ctrl Pts',(2.06854248895728,-1.,-0.745832791378367));
#28269=CARTESIAN_POINT('Ctrl Pts',(2.0698113262342,-1.,-0.745574324794401));
#28270=CARTESIAN_POINT('',(2.11275013067528,-1.,-0.61342227326009));
#28271=CARTESIAN_POINT('',(2.0698113262342,-1.,-0.745574324794401));
#28272=CARTESIAN_POINT('',(1.7075470150345,-1.,-0.383122945602004));
#28273=CARTESIAN_POINT('Ctrl Pts',(2.11275013067528,-1.,-0.61342227326009));
#28274=CARTESIAN_POINT('Ctrl Pts',(2.11187554259986,-1.,-0.6124673655618));
#28275=CARTESIAN_POINT('Ctrl Pts',(2.11012443807238,-1.,-0.610560911689899));
#28276=CARTESIAN_POINT('Ctrl Pts',(2.1074919961518,-1.,-0.607711315454876));
#28277=CARTESIAN_POINT('Ctrl Pts',(2.10397049886949,-1.,-0.60393203073603));
#28278=CARTESIAN_POINT('Ctrl Pts',(2.0995493086477,-1.,-0.599241616420534));
#28279=CARTESIAN_POINT('Ctrl Pts',(2.0951087622027,-1.,-0.594585006052162));
#28280=CARTESIAN_POINT('Ctrl Pts',(2.09064881812129,-1.,-0.589962365403406));
#28281=CARTESIAN_POINT('Ctrl Pts',(2.08616943727951,-1.,-0.585373918991617));
#28282=CARTESIAN_POINT('Ctrl Pts',(2.08167059018418,-1.,-0.580819952108064));
#28283=CARTESIAN_POINT('Ctrl Pts',(2.07715226767559,-1.,-0.576300797416845));
#28284=CARTESIAN_POINT('Ctrl Pts',(2.07261449292824,-1.,-0.571816823242603));
#28285=CARTESIAN_POINT('Ctrl Pts',(2.06805732997334,-1.,-0.567368421181087));
#28286=CARTESIAN_POINT('Ctrl Pts',(2.06348090160589,-1.,-0.562955993082262));
#28287=CARTESIAN_POINT('Ctrl Pts',(2.05888537756462,-1.,-0.558579940185152));
#28288=CARTESIAN_POINT('Ctrl Pts',(2.05427091604413,-1.,-0.554240657463906));
#28289=CARTESIAN_POINT('Ctrl Pts',(2.04963761077958,-1.,-0.549938525150295));
#28290=CARTESIAN_POINT('Ctrl Pts',(2.04498544714588,-1.,-0.54567390381743));
#28291=CARTESIAN_POINT('Ctrl Pts',(2.04031422690527,-1.,-0.541447120615659));
#28292=CARTESIAN_POINT('Ctrl Pts',(2.03562362954037,-1.,-0.537258489833262));
#28293=CARTESIAN_POINT('Ctrl Pts',(2.03091336214426,-1.,-0.533108355132977));
#28294=CARTESIAN_POINT('Ctrl Pts',(2.0261832908329,-1.,-0.528997127241914));
#28295=CARTESIAN_POINT('Ctrl Pts',(2.02143356304698,-1.,-0.524925318333476));
#28296=CARTESIAN_POINT('Ctrl Pts',(2.01666477917286,-1.,-0.520893590399371));
#28297=CARTESIAN_POINT('Ctrl Pts',(2.01187773939242,-1.,-0.516902681728687));
#28298=CARTESIAN_POINT('Ctrl Pts',(2.00707309946949,-1.,-0.512953306961793));
#28299=CARTESIAN_POINT('Ctrl Pts',(2.00225107134734,-1.,-0.509046069886157));
#28300=CARTESIAN_POINT('Ctrl Pts',(1.99741107463572,-1.,-0.505181361323026));
#28301=CARTESIAN_POINT('Ctrl Pts',(1.99255149126155,-1.,-0.501359287727146));
#28302=CARTESIAN_POINT('Ctrl Pts',(1.98767044752932,-1.,-0.497579909545574));
#28303=CARTESIAN_POINT('Ctrl Pts',(1.98276658761821,-1.,-0.493843476541495));
#28304=CARTESIAN_POINT('Ctrl Pts',(1.97783973019229,-1.,-0.490150627860953));
#28305=CARTESIAN_POINT('Ctrl Pts',(1.97289186263272,-1.,-0.486502692907659));
#28306=CARTESIAN_POINT('Ctrl Pts',(1.96792703422362,-1.,-0.482901662120691));
#28307=CARTESIAN_POINT('Ctrl Pts',(1.96294933055943,-1.,-0.479349583074855));
#28308=CARTESIAN_POINT('Ctrl Pts',(1.95796111148177,-1.,-0.475848034683176));
#28309=CARTESIAN_POINT('Ctrl Pts',(1.95296148278133,-1.,-0.472397672264072));
#28310=CARTESIAN_POINT('Ctrl Pts',(1.94794381136514,-1.,-0.468997482913135));
#28311=CARTESIAN_POINT('Ctrl Pts',(1.9428979419619,-1.,-0.46564546202603));
#28312=CARTESIAN_POINT('Ctrl Pts',(1.93781486640821,-1.,-0.462340031009057));
#28313=CARTESIAN_POINT('Ctrl Pts',(1.93269066517934,-1.,-0.459081234547926));
#28314=CARTESIAN_POINT('Ctrl Pts',(1.92753067150476,-1.,-0.455872005174371));
#28315=CARTESIAN_POINT('Ctrl Pts',(1.92235380648502,-1.,-0.452719478359433));
#28316=CARTESIAN_POINT('Ctrl Pts',(1.91718342555755,-1.,-0.449632260106662));
#28317=CARTESIAN_POINT('Ctrl Pts',(1.9120369998112,-1.,-0.446617343485711));
#28318=CARTESIAN_POINT('Ctrl Pts',(1.90691756144898,-1.,-0.443677556849151));
#28319=CARTESIAN_POINT('Ctrl Pts',(1.90180124389086,-1.,-0.440807833704038));
#28320=CARTESIAN_POINT('Ctrl Pts',(1.89663648956466,-1.,-0.437995003948244));
#28321=CARTESIAN_POINT('Ctrl Pts',(1.89136993975504,-1.,-0.435225660963383));
#28322=CARTESIAN_POINT('Ctrl Pts',(1.88596913666793,-1.,-0.432493038548748));
#28323=CARTESIAN_POINT('Ctrl Pts',(1.88044229001832,-1.,-0.429803062482345));
#28324=CARTESIAN_POINT('Ctrl Pts',(1.87486989291484,-1.,-0.427183828519102));
#28325=CARTESIAN_POINT('Ctrl Pts',(1.86937803944323,-1.,-0.424678177291359));
#28326=CARTESIAN_POINT('Ctrl Pts',(1.86408083334028,-1.,-0.422327307418275));
#28327=CARTESIAN_POINT('Ctrl Pts',(1.85903281096686,-1.,-0.42015728797562));
#28328=CARTESIAN_POINT('Ctrl Pts',(1.85417632856234,-1.,-0.418164129143534));
#28329=CARTESIAN_POINT('Ctrl Pts',(1.84929312929882,-1.,-0.416300022038864));
#28330=CARTESIAN_POINT('Ctrl Pts',(1.8440575707371,-1.,-0.41448743825434));
#28331=CARTESIAN_POINT('Ctrl Pts',(1.83808953475839,-1.,-0.412633125322162));
#28332=CARTESIAN_POINT('Ctrl Pts',(1.83100408895216,-1.,-0.410641256301675));
#28333=CARTESIAN_POINT('Ctrl Pts',(1.8224702267854,-1.,-0.408428948108534));
#28334=CARTESIAN_POINT('Ctrl Pts',(1.81223801813988,-1.,-0.405933518411838));
#28335=CARTESIAN_POINT('Ctrl Pts',(1.80012077176221,-1.,-0.403107976170441));
#28336=CARTESIAN_POINT('Ctrl Pts',(1.78598826347533,-1.,-0.399919403783081));
#28337=CARTESIAN_POINT('Ctrl Pts',(1.7697556004756,-1.,-0.39634619612042));
#28338=CARTESIAN_POINT('Ctrl Pts',(1.75137405313962,-1.,-0.392375812294307));
#28339=CARTESIAN_POINT('Ctrl Pts',(1.7349317097561,-1.,-0.388877023509192));
#28340=CARTESIAN_POINT('Ctrl Pts',(1.72162022246158,-1.,-0.38607079032701));
#28341=CARTESIAN_POINT('Ctrl Pts',(1.71231062891958,-1.,-0.384119047315542));
#28342=CARTESIAN_POINT('Ctrl Pts',(1.7075470150345,-1.,-0.383122945602004));
#28343=CARTESIAN_POINT('',(1.74236521665491,-1.,-0.163289472382896));
#28344=CARTESIAN_POINT('Origin',(0.,-1.,0.));
#28345=CARTESIAN_POINT('',(2.19890268624765,-1.,-0.0694764450219582));
#28346=CARTESIAN_POINT('Ctrl Pts',(1.74236521665491,-1.,-0.163289472382896));
#28347=CARTESIAN_POINT('Ctrl Pts',(1.7472034950333,-1.,-0.163814161002002));
#28348=CARTESIAN_POINT('Ctrl Pts',(1.75666056638427,-1.,-0.164834765707159));
#28349=CARTESIAN_POINT('Ctrl Pts',(1.77018771684844,-1.,-0.1662793551464));
#28350=CARTESIAN_POINT('Ctrl Pts',(1.7869064998507,-1.,-0.168032772805197));
#28351=CARTESIAN_POINT('Ctrl Pts',(1.80561530629706,-1.,-0.169936923904608));
#28352=CARTESIAN_POINT('Ctrl Pts',(1.82215766811545,-1.,-0.171554770204119));
#28353=CARTESIAN_POINT('Ctrl Pts',(1.83658380527692,-1.,-0.1728894428919));
#28354=CARTESIAN_POINT('Ctrl Pts',(1.8489811319852,-1.,-0.173946627587732));
#28355=CARTESIAN_POINT('Ctrl Pts',(1.85948367088837,-1.,-0.17473525927603));
#28356=CARTESIAN_POINT('Ctrl Pts',(1.86828349694799,-1.,-0.175268337590758));
#28357=CARTESIAN_POINT('Ctrl Pts',(1.87563767773588,-1.,-0.175563480746485));
#28358=CARTESIAN_POINT('Ctrl Pts',(1.88188663145367,-1.,-0.175644148889699));
#28359=CARTESIAN_POINT('Ctrl Pts',(1.88742606273259,-1.,-0.175538155840648));
#28360=CARTESIAN_POINT('Ctrl Pts',(1.892646301985,-1.,-0.175274276190844));
#28361=CARTESIAN_POINT('Ctrl Pts',(1.89788101117132,-1.,-0.174879405091263));
#28362=CARTESIAN_POINT('Ctrl Pts',(1.90335253862834,-1.,-0.174375518661085));
#28363=CARTESIAN_POINT('Ctrl Pts',(1.90911693975267,-1.,-0.173776635257817));
#28364=CARTESIAN_POINT('Ctrl Pts',(1.91511429159527,-1.,-0.173090695383496));
#28365=CARTESIAN_POINT('Ctrl Pts',(1.9212233439798,-1.,-0.172321621259514));
#28366=CARTESIAN_POINT('Ctrl Pts',(1.92731093582036,-1.,-0.171471191532988));
#28367=CARTESIAN_POINT('Ctrl Pts',(1.93329183155539,-1.,-0.170541253116202));
#28368=CARTESIAN_POINT('Ctrl Pts',(1.93915639211581,-1.,-0.169534904817491));
#28369=CARTESIAN_POINT('Ctrl Pts',(1.94493757756931,-1.,-0.168455741607556));
#28370=CARTESIAN_POINT('Ctrl Pts',(1.95069027794294,-1.,-0.167307501784476));
#28371=CARTESIAN_POINT('Ctrl Pts',(1.9564675971873,-1.,-0.166093592002813));
#28372=CARTESIAN_POINT('Ctrl Pts',(1.96229379940136,-1.,-0.164816568920269));
#28373=CARTESIAN_POINT('Ctrl Pts',(1.96816512677967,-1.,-0.163478185457734));
#28374=CARTESIAN_POINT('Ctrl Pts',(1.97406280235188,-1.,-0.162079693556289));
#28375=CARTESIAN_POINT('Ctrl Pts',(1.97996195437559,-1.,-0.160622060784611));
#28376=CARTESIAN_POINT('Ctrl Pts',(1.98584238283292,-1.,-0.159106226437299));
#28377=CARTESIAN_POINT('Ctrl Pts',(1.99169810931908,-1.,-0.157533331459227));
#28378=CARTESIAN_POINT('Ctrl Pts',(1.99753284771497,-1.,-0.155904629548784));
#28379=CARTESIAN_POINT('Ctrl Pts',(2.00335565310543,-1.,-0.154221403049722));
#28380=CARTESIAN_POINT('Ctrl Pts',(2.00917680318424,-1.,-0.15248488362145));
#28381=CARTESIAN_POINT('Ctrl Pts',(2.01500291940238,-1.,-0.150696157673078));
#28382=CARTESIAN_POINT('Ctrl Pts',(2.02083464969894,-1.,-0.148856124775337));
#28383=CARTESIAN_POINT('Ctrl Pts',(2.02666926182017,-1.,-0.146965557332583));
#28384=CARTESIAN_POINT('Ctrl Pts',(2.03250223739942,-1.,-0.145025140186058));
#28385=CARTESIAN_POINT('Ctrl Pts',(2.03832911025912,-1.,-0.143035515058209));
#28386=CARTESIAN_POINT('Ctrl Pts',(2.04414757947916,-1.,-0.140997332152546));
#28387=CARTESIAN_POINT('Ctrl Pts',(2.04995762001328,-1.,-0.138911255368966));
#28388=CARTESIAN_POINT('Ctrl Pts',(2.05576044414264,-1.,-0.136777941218044));
#28389=CARTESIAN_POINT('Ctrl Pts',(2.06155781517842,-1.,-0.134598026192106));
#28390=CARTESIAN_POINT('Ctrl Pts',(2.06735123910326,-1.,-0.132372111547711));
#28391=CARTESIAN_POINT('Ctrl Pts',(2.07314114713063,-1.,-0.130100748328404));
#28392=CARTESIAN_POINT('Ctrl Pts',(2.07892715110987,-1.,-0.12778444527612));
#28393=CARTESIAN_POINT('Ctrl Pts',(2.08470840653643,-1.,-0.125423679412062));
#28394=CARTESIAN_POINT('Ctrl Pts',(2.09048392424825,-1.,-0.123018905621083));
#28395=CARTESIAN_POINT('Ctrl Pts',(2.0962529286773,-1.,-0.120570567965122));
#28396=CARTESIAN_POINT('Ctrl Pts',(2.102015121329,-1.,-0.118079107988356));
#28397=CARTESIAN_POINT('Ctrl Pts',(2.10777050261309,-1.,-0.115544957687927));
#28398=CARTESIAN_POINT('Ctrl Pts',(2.11351924490306,-1.,-0.112968534419737));
#28399=CARTESIAN_POINT('Ctrl Pts',(2.11926155590865,-1.,-0.110350236135025));
#28400=CARTESIAN_POINT('Ctrl Pts',(2.12499752307,-1.,-0.10769043523109));
#28401=CARTESIAN_POINT('Ctrl Pts',(2.13072704887293,-1.,-0.10498947915274));
#28402=CARTESIAN_POINT('Ctrl Pts',(2.13644992667165,-1.,-0.102247700556101));
#28403=CARTESIAN_POINT('Ctrl Pts',(2.14216588396025,-1.,-0.0994654261990917));
#28404=CARTESIAN_POINT('Ctrl Pts',(2.14787463531795,-1.,-0.096642985230546));
#28405=CARTESIAN_POINT('Ctrl Pts',(2.1535759397817,-1.,-0.0937807218867645));
#28406=CARTESIAN_POINT('Ctrl Pts',(2.15926961544516,-1.,-0.0908789888107267));
#28407=CARTESIAN_POINT('Ctrl Pts',(2.16495552645014,-1.,-0.0879381291386924));
#28408=CARTESIAN_POINT('Ctrl Pts',(2.17063357870952,-1.,-0.0849584620835374));
#28409=CARTESIAN_POINT('Ctrl Pts',(2.176303712113,-1.,-0.0819402680872767));
#28410=CARTESIAN_POINT('Ctrl Pts',(2.18196589448887,-1.,-0.0788837727685244));
#28411=CARTESIAN_POINT('Ctrl Pts',(2.1876201139953,-1.,-0.0757891465836149));
#28412=CARTESIAN_POINT('Ctrl Pts',(2.19213712013662,-1.,-0.0732830357306726));
#28413=CARTESIAN_POINT('Ctrl Pts',(2.19552129484002,-1.,-0.0713863779526155));
#28414=CARTESIAN_POINT('Ctrl Pts',(2.19777582085423,-1.,-0.0701143536325491));
#28415=CARTESIAN_POINT('Ctrl Pts',(2.19890268624765,-1.,-0.0694764450219582));
#28416=CARTESIAN_POINT('',(2.19890268624765,-1.,0.0694764450219582));
#28417=CARTESIAN_POINT('',(2.19890268624765,-1.,-0.0694764450219582));
#28418=CARTESIAN_POINT('',(1.74236521665491,-1.,0.163289472382896));
#28419=CARTESIAN_POINT('Ctrl Pts',(2.19890268624765,-1.,0.0694764450219582));
#28420=CARTESIAN_POINT('Ctrl Pts',(2.19777582085261,-1.,0.0701143536324925));
#28421=CARTESIAN_POINT('Ctrl Pts',(2.19552129483562,-1.,0.0713863779524626));
#28422=CARTESIAN_POINT('Ctrl Pts',(2.19213712012956,-1.,0.0732830357304275));
#28423=CARTESIAN_POINT('Ctrl Pts',(2.1876201139874,-1.,0.075789146583341));
#28424=CARTESIAN_POINT('Ctrl Pts',(2.18196589448304,-1.,0.0788837727683226));
#28425=CARTESIAN_POINT('Ctrl Pts',(2.1763037121106,-1.,0.0819402680871938));
#28426=CARTESIAN_POINT('Ctrl Pts',(2.17063357871031,-1.,0.0849584620835642));
#28427=CARTESIAN_POINT('Ctrl Pts',(2.16495552645275,-1.,0.0879381291387821));
#28428=CARTESIAN_POINT('Ctrl Pts',(2.15926961544808,-1.,0.0908789888108265));
#28429=CARTESIAN_POINT('Ctrl Pts',(2.15357593978377,-1.,0.0937807218868344));
#28430=CARTESIAN_POINT('Ctrl Pts',(2.14787463531864,-1.,0.0966429852305688));
#28431=CARTESIAN_POINT('Ctrl Pts',(2.14216588395974,-1.,0.0994654261990741));
#28432=CARTESIAN_POINT('Ctrl Pts',(2.13644992667052,-1.,0.102247700556063));
#28433=CARTESIAN_POINT('Ctrl Pts',(2.1307270488718,-1.,0.104989479152703));
#28434=CARTESIAN_POINT('Ctrl Pts',(2.12499752306927,-1.,0.107690435231068));
#28435=CARTESIAN_POINT('Ctrl Pts',(2.11926155590849,-1.,0.11035023613502));
#28436=CARTESIAN_POINT('Ctrl Pts',(2.11351924490335,-1.,0.112968534419746));
#28437=CARTESIAN_POINT('Ctrl Pts',(2.10777050261359,-1.,0.11554495768794));
#28438=CARTESIAN_POINT('Ctrl Pts',(2.10201512132945,-1.,0.118079107988368));
#28439=CARTESIAN_POINT('Ctrl Pts',(2.09625292867756,-1.,0.120570567965129));
#28440=CARTESIAN_POINT('Ctrl Pts',(2.09048392424826,-1.,0.123018905621083));
#28441=CARTESIAN_POINT('Ctrl Pts',(2.08470840653628,-1.,0.125423679412058));
#28442=CARTESIAN_POINT('Ctrl Pts',(2.07892715110967,-1.,0.127784445276116));
#28443=CARTESIAN_POINT('Ctrl Pts',(2.07314114713047,-1.,0.1301007483284));
#28444=CARTESIAN_POINT('Ctrl Pts',(2.06735123910319,-1.,0.132372111547709));
#28445=CARTESIAN_POINT('Ctrl Pts',(2.06155781517844,-1.,0.134598026192107));
#28446=CARTESIAN_POINT('Ctrl Pts',(2.0557604441427,-1.,0.136777941218044));
#28447=CARTESIAN_POINT('Ctrl Pts',(2.04995762001333,-1.,0.138911255368966));
#28448=CARTESIAN_POINT('Ctrl Pts',(2.04414757947919,-1.,0.140997332152545));
#28449=CARTESIAN_POINT('Ctrl Pts',(2.03832911025913,-1.,0.143035515058208));
#28450=CARTESIAN_POINT('Ctrl Pts',(2.03250223739941,-1.,0.145025140186058));
#28451=CARTESIAN_POINT('Ctrl Pts',(2.02666926182017,-1.,0.146965557332586));
#28452=CARTESIAN_POINT('Ctrl Pts',(2.02083464969897,-1.,0.148856124775342));
#28453=CARTESIAN_POINT('Ctrl Pts',(2.01500291940243,-1.,0.150696157673084));
#28454=CARTESIAN_POINT('Ctrl Pts',(2.00917680318426,-1.,0.152484883621452));
#28455=CARTESIAN_POINT('Ctrl Pts',(2.00335565310539,-1.,0.154221403049719));
#28456=CARTESIAN_POINT('Ctrl Pts',(1.99753284771487,-1.,0.155904629548774));
#28457=CARTESIAN_POINT('Ctrl Pts',(1.99169810931893,-1.,0.157533331459215));
#28458=CARTESIAN_POINT('Ctrl Pts',(1.98584238283279,-1.,0.159106226437288));
#28459=CARTESIAN_POINT('Ctrl Pts',(1.97996195437557,-1.,0.16062206078461));
#28460=CARTESIAN_POINT('Ctrl Pts',(1.97406280235204,-1.,0.162079693556302));
#28461=CARTESIAN_POINT('Ctrl Pts',(1.96816512678,-1.,0.16347818545776));
#28462=CARTESIAN_POINT('Ctrl Pts',(1.96229379940174,-1.,0.1648165689203));
#28463=CARTESIAN_POINT('Ctrl Pts',(1.95646759718755,-1.,0.166093592002832));
#28464=CARTESIAN_POINT('Ctrl Pts',(1.95069027794286,-1.,0.167307501784469));
#28465=CARTESIAN_POINT('Ctrl Pts',(1.94493757756879,-1.,0.168455741607515));
#28466=CARTESIAN_POINT('Ctrl Pts',(1.93915639211497,-1.,0.169534904817425));
#28467=CARTESIAN_POINT('Ctrl Pts',(1.93329183155455,-1.,0.170541253116136));
#28468=CARTESIAN_POINT('Ctrl Pts',(1.92731093582,-1.,0.17147119153296));
#28469=CARTESIAN_POINT('Ctrl Pts',(1.92122334398034,-1.,0.172321621259556));
#28470=CARTESIAN_POINT('Ctrl Pts',(1.91511429159681,-1.,0.173090695383619));
#28471=CARTESIAN_POINT('Ctrl Pts',(1.90911693975475,-1.,0.173776635257983));
#28472=CARTESIAN_POINT('Ctrl Pts',(1.90335253863003,-1.,0.174375518661222));
#28473=CARTESIAN_POINT('Ctrl Pts',(1.89788101117148,-1.,0.174879405091277));
#28474=CARTESIAN_POINT('Ctrl Pts',(1.89264630198279,-1.,0.175274276190664));
#28475=CARTESIAN_POINT('Ctrl Pts',(1.88742606272818,-1.,0.175538155840286));
#28476=CARTESIAN_POINT('Ctrl Pts',(1.88188663144846,-1.,0.175644148889271));
#28477=CARTESIAN_POINT('Ctrl Pts',(1.87563767773249,-1.,0.175563480746205));
#28478=CARTESIAN_POINT('Ctrl Pts',(1.86828349694972,-1.,0.1752683375909));
#28479=CARTESIAN_POINT('Ctrl Pts',(1.85948367089838,-1.,0.174735259276856));
#28480=CARTESIAN_POINT('Ctrl Pts',(1.84898113200543,-1.,0.173946627589401));
#28481=CARTESIAN_POINT('Ctrl Pts',(1.83658380530747,-1.,0.17288944289442));
#28482=CARTESIAN_POINT('Ctrl Pts',(1.82215766815414,-1.,0.171554770207306));
#28483=CARTESIAN_POINT('Ctrl Pts',(1.80561530633924,-1.,0.169936923908078));
#28484=CARTESIAN_POINT('Ctrl Pts',(1.78690649988931,-1.,0.16803277280837));
#28485=CARTESIAN_POINT('Ctrl Pts',(1.77018771687692,-1.,0.166279355148738));
#28486=CARTESIAN_POINT('Ctrl Pts',(1.75666056640041,-1.,0.164834765708484));
#28487=CARTESIAN_POINT('Ctrl Pts',(1.74720349503904,-1.,0.163814161002474));
#28488=CARTESIAN_POINT('Ctrl Pts',(1.74236521665491,-1.,0.163289472382896));
#28489=CARTESIAN_POINT('',(1.7075470150345,-1.,0.383122945602004));
#28490=CARTESIAN_POINT('Origin',(0.,-1.,0.));
#28491=CARTESIAN_POINT('',(2.11275013067528,-1.,0.613422273260091));
#28492=CARTESIAN_POINT('Ctrl Pts',(1.7075470150345,-1.,0.383122945602004));
#28493=CARTESIAN_POINT('Ctrl Pts',(1.71231062891398,-1.,0.384119047314215));
#28494=CARTESIAN_POINT('Ctrl Pts',(1.72162022244582,-1.,0.386070790323281));
#28495=CARTESIAN_POINT('Ctrl Pts',(1.73493170972829,-1.,0.388877023502615));
#28496=CARTESIAN_POINT('Ctrl Pts',(1.75137405310193,-1.,0.392375812285396));
#28497=CARTESIAN_POINT('Ctrl Pts',(1.76975560043442,-1.,0.396346196110688));
#28498=CARTESIAN_POINT('Ctrl Pts',(1.78598826343754,-1.,0.399919403774156));
#28499=CARTESIAN_POINT('Ctrl Pts',(1.80012077173238,-1.,0.403107976163396));
#28500=CARTESIAN_POINT('Ctrl Pts',(1.81223801812013,-1.,0.405933518407176));
#28501=CARTESIAN_POINT('Ctrl Pts',(1.82247022677562,-1.,0.408428948106228));
#28502=CARTESIAN_POINT('Ctrl Pts',(1.83100408895047,-1.,0.410641256301276));
#28503=CARTESIAN_POINT('Ctrl Pts',(1.8380895347617,-1.,0.412633125322945));
#28504=CARTESIAN_POINT('Ctrl Pts',(1.84405757074218,-1.,0.414487438255542));
#28505=CARTESIAN_POINT('Ctrl Pts',(1.84929312930314,-1.,0.416300022039885));
#28506=CARTESIAN_POINT('Ctrl Pts',(1.8541763285645,-1.,0.418164129144046));
#28507=CARTESIAN_POINT('Ctrl Pts',(1.8590328109667,-1.,0.420157287975583));
#28508=CARTESIAN_POINT('Ctrl Pts',(1.86408083333863,-1.,0.422327307417885));
#28509=CARTESIAN_POINT('Ctrl Pts',(1.8693780394412,-1.,0.424678177290876));
#28510=CARTESIAN_POINT('Ctrl Pts',(1.87486989291333,-1.,0.427183828518743));
#28511=CARTESIAN_POINT('Ctrl Pts',(1.88044229001778,-1.,0.429803062482217));
#28512=CARTESIAN_POINT('Ctrl Pts',(1.88596913666828,-1.,0.432493038548833));
#28513=CARTESIAN_POINT('Ctrl Pts',(1.89136993975585,-1.,0.43522566096358));
#28514=CARTESIAN_POINT('Ctrl Pts',(1.89663648956549,-1.,0.437995003948443));
#28515=CARTESIAN_POINT('Ctrl Pts',(1.90180124389137,-1.,0.440807833704161));
#28516=CARTESIAN_POINT('Ctrl Pts',(1.90691756144906,-1.,0.443677556849171));
#28517=CARTESIAN_POINT('Ctrl Pts',(1.91203699981095,-1.,0.446617343485651));
#28518=CARTESIAN_POINT('Ctrl Pts',(1.91718342555717,-1.,0.449632260106572));
#28519=CARTESIAN_POINT('Ctrl Pts',(1.9223538064847,-1.,0.452719478359356));
#28520=CARTESIAN_POINT('Ctrl Pts',(1.92753067150461,-1.,0.455872005174336));
#28521=CARTESIAN_POINT('Ctrl Pts',(1.93269066517936,-1.,0.459081234547932));
#28522=CARTESIAN_POINT('Ctrl Pts',(1.93781486640834,-1.,0.462340031009087));
#28523=CARTESIAN_POINT('Ctrl Pts',(1.94289794196205,-1.,0.465645462026065));
#28524=CARTESIAN_POINT('Ctrl Pts',(1.94794381136524,-1.,0.468997482913158));
#28525=CARTESIAN_POINT('Ctrl Pts',(1.95296148278136,-1.,0.47239767226408));
#28526=CARTESIAN_POINT('Ctrl Pts',(1.95796111148175,-1.,0.475848034683172));
#28527=CARTESIAN_POINT('Ctrl Pts',(1.96294933055938,-1.,0.479349583074846));
#28528=CARTESIAN_POINT('Ctrl Pts',(1.96792703422358,-1.,0.482901662120687));
#28529=CARTESIAN_POINT('Ctrl Pts',(1.97289186263272,-1.,0.486502692907661));
#28530=CARTESIAN_POINT('Ctrl Pts',(1.97783973019229,-1.,0.490150627860955));
#28531=CARTESIAN_POINT('Ctrl Pts',(1.9827665876182,-1.,0.493843476541493));
#28532=CARTESIAN_POINT('Ctrl Pts',(1.98767044752929,-1.,0.497579909545564));
#28533=CARTESIAN_POINT('Ctrl Pts',(1.9925514912615,-1.,0.501359287727129));
#28534=CARTESIAN_POINT('Ctrl Pts',(1.99741107463567,-1.,0.505181361323011));
#28535=CARTESIAN_POINT('Ctrl Pts',(2.00225107134733,-1.,0.509046069886152));
#28536=CARTESIAN_POINT('Ctrl Pts',(2.00707309946955,-1.,0.512953306961814));
#28537=CARTESIAN_POINT('Ctrl Pts',(2.01187773939257,-1.,0.516902681728733));
#28538=CARTESIAN_POINT('Ctrl Pts',(2.01666477917305,-1.,0.520893590399429));
#28539=CARTESIAN_POINT('Ctrl Pts',(2.02143356304712,-1.,0.524925318333519));
#28540=CARTESIAN_POINT('Ctrl Pts',(2.02618329083289,-1.,0.528997127241911));
#28541=CARTESIAN_POINT('Ctrl Pts',(2.03091336214401,-1.,0.533108355132905));
#28542=CARTESIAN_POINT('Ctrl Pts',(2.03562362953993,-1.,0.537258489833135));
#28543=CARTESIAN_POINT('Ctrl Pts',(2.0403142269048,-1.,0.54144712061552));
#28544=CARTESIAN_POINT('Ctrl Pts',(2.0449854471456,-1.,0.545673903817349));
#28545=CARTESIAN_POINT('Ctrl Pts',(2.04963761077974,-1.,0.549938525150342));
#28546=CARTESIAN_POINT('Ctrl Pts',(2.05427091604482,-1.,0.55424065746411));
#28547=CARTESIAN_POINT('Ctrl Pts',(2.05888537756571,-1.,0.558579940185468));
#28548=CARTESIAN_POINT('Ctrl Pts',(2.06348090160697,-1.,0.562955993082574));
#28549=CARTESIAN_POINT('Ctrl Pts',(2.06805732997383,-1.,0.56736842118123));
#28550=CARTESIAN_POINT('Ctrl Pts',(2.07261449292757,-1.,0.571816823242411));
#28551=CARTESIAN_POINT('Ctrl Pts',(2.07715226767361,-1.,0.576300797416275));
#28552=CARTESIAN_POINT('Ctrl Pts',(2.08167059018138,-1.,0.580819952107257));
#28553=CARTESIAN_POINT('Ctrl Pts',(2.086169437277,-1.,0.585373918990895));
#28554=CARTESIAN_POINT('Ctrl Pts',(2.09064881812053,-1.,0.58996236540319));
#28555=CARTESIAN_POINT('Ctrl Pts',(2.09510876220501,-1.,0.594585006052824));
#28556=CARTESIAN_POINT('Ctrl Pts',(2.09954930865331,-1.,0.599241616422144));
#28557=CARTESIAN_POINT('Ctrl Pts',(2.10397049887709,-1.,0.603932030738212));
#28558=CARTESIAN_POINT('Ctrl Pts',(2.10749199615859,-1.,0.607711315456826));
#28559=CARTESIAN_POINT('Ctrl Pts',(2.11012443807661,-1.,0.610560911691114));
#28560=CARTESIAN_POINT('Ctrl Pts',(2.11187554260142,-1.,0.61246736556225));
#28561=CARTESIAN_POINT('Ctrl Pts',(2.11275013067528,-1.,0.613422273260091));
#28562=CARTESIAN_POINT('',(2.0698113262342,-1.,0.745574324794401));
#28563=CARTESIAN_POINT('',(2.11275013067528,-1.,0.613422273260091));
#28564=CARTESIAN_POINT('Ctrl Pts',(2.0698113262342,-1.,0.745574324794401));
#28565=CARTESIAN_POINT('Ctrl Pts',(2.06854248895575,-1.,0.74583279137781));
#28566=CARTESIAN_POINT('Ctrl Pts',(2.06600523016401,-1.,0.746345871542696));
#28567=CARTESIAN_POINT('Ctrl Pts',(2.06220058927162,-1.,0.747103932785504));
#28568=CARTESIAN_POINT('Ctrl Pts',(2.05713023030263,-1.,0.748091554181101));
#28569=CARTESIAN_POINT('Ctrl Pts',(2.05079645591606,-1.,0.749287468663053));
#28570=CARTESIAN_POINT('Ctrl Pts',(2.04446689147754,-1.,0.750444657874758));
#28571=CARTESIAN_POINT('Ctrl Pts',(2.03814160092173,-1.,0.751562963361384));
#28572=CARTESIAN_POINT('Ctrl Pts',(2.03182068456467,-1.,0.752642180488104));
#28573=CARTESIAN_POINT('Ctrl Pts',(2.02550428623587,-1.,0.753682061113766));
#28574=CARTESIAN_POINT('Ctrl Pts',(2.01919259406003,-1.,0.75468233072352));
#28575=CARTESIAN_POINT('Ctrl Pts',(2.01288584328149,-1.,0.755642704958101));
#28576=CARTESIAN_POINT('Ctrl Pts',(2.00658431587682,-1.,0.756562904646496));
#28577=CARTESIAN_POINT('Ctrl Pts',(2.00028834739072,-1.,0.757442676862342));
#28578=CARTESIAN_POINT('Ctrl Pts',(1.9939983109871,-1.,0.758281796766377));
#28579=CARTESIAN_POINT('Ctrl Pts',(1.98771456680806,-1.,0.759080037802243));
#28580=CARTESIAN_POINT('Ctrl Pts',(1.98143741418156,-1.,0.759837147452135));
#28581=CARTESIAN_POINT('Ctrl Pts',(1.97516705321521,-1.,0.760552825409856));
#28582=CARTESIAN_POINT('Ctrl Pts',(1.96890351582545,-1.,0.761226690483986));
#28583=CARTESIAN_POINT('Ctrl Pts',(1.96264672744229,-1.,0.761858300014575));
#28584=CARTESIAN_POINT('Ctrl Pts',(1.95639665309893,-1.,0.762447203806264));
#28585=CARTESIAN_POINT('Ctrl Pts',(1.95015342590025,-1.,0.762992990878774));
#28586=CARTESIAN_POINT('Ctrl Pts',(1.94391746617626,-1.,0.763495333538581));
#28587=CARTESIAN_POINT('Ctrl Pts',(1.93768964875867,-1.,0.763954049121394));
#28588=CARTESIAN_POINT('Ctrl Pts',(1.93147105496367,-1.,0.76436901067389));
#28589=CARTESIAN_POINT('Ctrl Pts',(1.92526263537041,-1.,0.764740025488189));
#28590=CARTESIAN_POINT('Ctrl Pts',(1.91906491634197,-1.,0.765066729667095));
#28591=CARTESIAN_POINT('Ctrl Pts',(1.91287765805174,-1.,0.765348465884739));
#28592=CARTESIAN_POINT('Ctrl Pts',(1.90669961402362,-1.,0.765584196937937));
#28593=CARTESIAN_POINT('Ctrl Pts',(1.90052930393599,-1.,0.765772772593395));
#28594=CARTESIAN_POINT('Ctrl Pts',(1.89436577771389,-1.,0.765913193856979));
#28595=CARTESIAN_POINT('Ctrl Pts',(1.88820926433409,-1.,0.76600483706209));
#28596=CARTESIAN_POINT('Ctrl Pts',(1.88206215302561,-1.,0.766047794851869));
#28597=CARTESIAN_POINT('Ctrl Pts',(1.87592888967886,-1.,0.766042837036759));
#28598=CARTESIAN_POINT('Ctrl Pts',(1.86981398314345,-1.,0.765990708546112));
#28599=CARTESIAN_POINT('Ctrl Pts',(1.86372027063314,-1.,0.765891519092557));
#28600=CARTESIAN_POINT('Ctrl Pts',(1.85764741390391,-1.,0.765744212909305));
#28601=CARTESIAN_POINT('Ctrl Pts',(1.85158945130054,-1.,0.765545710619023));
#28602=CARTESIAN_POINT('Ctrl Pts',(1.8455369887591,-1.,0.765291664861972));
#28603=CARTESIAN_POINT('Ctrl Pts',(1.83948181064823,-1.,0.764978057881688));
#28604=CARTESIAN_POINT('Ctrl Pts',(1.8334207722714,-1.,0.764602549687846));
#28605=CARTESIAN_POINT('Ctrl Pts',(1.8273599120008,-1.,0.764165902606056));
#28606=CARTESIAN_POINT('Ctrl Pts',(1.82131873145297,-1.,0.763673465462854));
#28607=CARTESIAN_POINT('Ctrl Pts',(1.81532118405566,-1.,0.763132003836783));
#28608=CARTESIAN_POINT('Ctrl Pts',(1.80938551463989,-1.,0.762546129464036));
#28609=CARTESIAN_POINT('Ctrl Pts',(1.80351583877334,-1.,0.761915336443516));
#28610=CARTESIAN_POINT('Ctrl Pts',(1.79768986997735,-1.,0.761229695230359));
#28611=CARTESIAN_POINT('Ctrl Pts',(1.79185815610802,-1.,0.760469555880425));
#28612=CARTESIAN_POINT('Ctrl Pts',(1.78596964884526,-1.,0.759614401109868));
#28613=CARTESIAN_POINT('Ctrl Pts',(1.77999411220912,-1.,0.75865062667738));
#28614=CARTESIAN_POINT('Ctrl Pts',(1.77394167108342,-1.,0.757578264077238));
#28615=CARTESIAN_POINT('Ctrl Pts',(1.76789396003141,-1.,0.756421896028403));
#28616=CARTESIAN_POINT('Ctrl Pts',(1.7619781724032,-1.,0.755220979975262));
#28617=CARTESIAN_POINT('Ctrl Pts',(1.75631083600175,-1.,0.75400925402848));
#28618=CARTESIAN_POINT('Ctrl Pts',(1.75095139468809,-1.,0.752797683531377));
#28619=CARTESIAN_POINT('Ctrl Pts',(1.74585086852298,-1.,0.751555614163629));
#28620=CARTESIAN_POINT('Ctrl Pts',(1.74080458266705,-1.,0.750193435979541));
#28621=CARTESIAN_POINT('Ctrl Pts',(1.73550351679848,-1.,0.748582462954855));
#28622=CARTESIAN_POINT('Ctrl Pts',(1.72958533647399,-1.,0.746574710096437));
#28623=CARTESIAN_POINT('Ctrl Pts',(1.7226822991693,-1.,0.744021445433765));
#28624=CARTESIAN_POINT('Ctrl Pts',(1.71447789751927,-1.,0.740795162032088));
#28625=CARTESIAN_POINT('Ctrl Pts',(1.70473309006121,-1.,0.736799665724771));
#28626=CARTESIAN_POINT('Ctrl Pts',(1.69326921975743,-1.,0.731963238697195));
#28627=CARTESIAN_POINT('Ctrl Pts',(1.67996158455503,-1.,0.726235967997433));
#28628=CARTESIAN_POINT('Ctrl Pts',(1.6647288055568,-1.,0.719585433804282));
#28629=CARTESIAN_POINT('Ctrl Pts',(1.64752408832016,-1.,0.711993139355394));
#28630=CARTESIAN_POINT('Ctrl Pts',(1.63216541664676,-1.,0.705159151988319));
#28631=CARTESIAN_POINT('Ctrl Pts',(1.61974673472612,-1.,0.699605146405088));
#28632=CARTESIAN_POINT('Ctrl Pts',(1.61106790958151,-1.,0.695712097881194));
#28633=CARTESIAN_POINT('Ctrl Pts',(1.60662857109684,-1.,0.693717979106306));
#28634=CARTESIAN_POINT('Origin',(0.,-1.,0.));
#28635=CARTESIAN_POINT('Origin',(0.,0.,0.));
#28636=CARTESIAN_POINT('Origin',(0.,2.2,0.));
#28637=CARTESIAN_POINT('Origin',(0.,1.,0.));
#28638=CARTESIAN_POINT('',(-1.4,2.2,1.71450551880629E-16));
#28639=CARTESIAN_POINT('Origin',(0.,2.2,0.));
#28640=CARTESIAN_POINT('',(-1.4,1.,1.71450551880629E-16));
#28641=CARTESIAN_POINT('',(-1.4,1.,1.71450551880629E-16));
#28642=CARTESIAN_POINT('Origin',(0.,1.,0.));
#28643=CARTESIAN_POINT('Origin',(0.,2.2,0.));
#28644=CARTESIAN_POINT('Ctrl Pts',(2.11275013067528,-1.,0.613422273260091));
#28645=CARTESIAN_POINT('Ctrl Pts',(2.11275013067528,1.,0.613422273260091));
#28646=CARTESIAN_POINT('Ctrl Pts',(2.11187554260142,-1.,0.61246736556225));
#28647=CARTESIAN_POINT('Ctrl Pts',(2.11187554260142,1.,0.61246736556225));
#28648=CARTESIAN_POINT('Ctrl Pts',(2.11012443807661,-1.,0.610560911691114));
#28649=CARTESIAN_POINT('Ctrl Pts',(2.11012443807661,1.,0.610560911691114));
#28650=CARTESIAN_POINT('Ctrl Pts',(2.10749199615859,-1.,0.607711315456826));
#28651=CARTESIAN_POINT('Ctrl Pts',(2.10749199615859,1.,0.607711315456826));
#28652=CARTESIAN_POINT('Ctrl Pts',(2.10397049887709,-1.,0.603932030738212));
#28653=CARTESIAN_POINT('Ctrl Pts',(2.10397049887709,1.,0.603932030738212));
#28654=CARTESIAN_POINT('Ctrl Pts',(2.09954930865331,-1.,0.599241616422144));
#28655=CARTESIAN_POINT('Ctrl Pts',(2.09954930865331,1.,0.599241616422144));
#28656=CARTESIAN_POINT('Ctrl Pts',(2.09510876220501,-1.,0.594585006052824));
#28657=CARTESIAN_POINT('Ctrl Pts',(2.09510876220501,1.,0.594585006052824));
#28658=CARTESIAN_POINT('Ctrl Pts',(2.09064881812053,-1.,0.58996236540319));
#28659=CARTESIAN_POINT('Ctrl Pts',(2.09064881812053,1.,0.58996236540319));
#28660=CARTESIAN_POINT('Ctrl Pts',(2.086169437277,-1.,0.585373918990895));
#28661=CARTESIAN_POINT('Ctrl Pts',(2.086169437277,1.,0.585373918990895));
#28662=CARTESIAN_POINT('Ctrl Pts',(2.08167059018138,-1.,0.580819952107257));
#28663=CARTESIAN_POINT('Ctrl Pts',(2.08167059018138,1.,0.580819952107257));
#28664=CARTESIAN_POINT('Ctrl Pts',(2.07715226767361,-1.,0.576300797416275));
#28665=CARTESIAN_POINT('Ctrl Pts',(2.07715226767361,1.,0.576300797416275));
#28666=CARTESIAN_POINT('Ctrl Pts',(2.07261449292757,-1.,0.571816823242411));
#28667=CARTESIAN_POINT('Ctrl Pts',(2.07261449292757,1.,0.571816823242411));
#28668=CARTESIAN_POINT('Ctrl Pts',(2.06805732997383,-1.,0.56736842118123));
#28669=CARTESIAN_POINT('Ctrl Pts',(2.06805732997383,1.,0.56736842118123));
#28670=CARTESIAN_POINT('Ctrl Pts',(2.06348090160697,-1.,0.562955993082574));
#28671=CARTESIAN_POINT('Ctrl Pts',(2.06348090160697,1.,0.562955993082574));
#28672=CARTESIAN_POINT('Ctrl Pts',(2.05888537756571,-1.,0.558579940185468));
#28673=CARTESIAN_POINT('Ctrl Pts',(2.05888537756571,1.,0.558579940185468));
#28674=CARTESIAN_POINT('Ctrl Pts',(2.05427091604482,-1.,0.55424065746411));
#28675=CARTESIAN_POINT('Ctrl Pts',(2.05427091604482,1.,0.55424065746411));
#28676=CARTESIAN_POINT('Ctrl Pts',(2.04963761077974,-1.,0.549938525150342));
#28677=CARTESIAN_POINT('Ctrl Pts',(2.04963761077974,1.,0.549938525150342));
#28678=CARTESIAN_POINT('Ctrl Pts',(2.0449854471456,-1.,0.545673903817349));
#28679=CARTESIAN_POINT('Ctrl Pts',(2.0449854471456,1.,0.545673903817349));
#28680=CARTESIAN_POINT('Ctrl Pts',(2.0403142269048,-1.,0.54144712061552));
#28681=CARTESIAN_POINT('Ctrl Pts',(2.0403142269048,1.,0.54144712061552));
#28682=CARTESIAN_POINT('Ctrl Pts',(2.03562362953993,-1.,0.537258489833135));
#28683=CARTESIAN_POINT('Ctrl Pts',(2.03562362953993,1.,0.537258489833135));
#28684=CARTESIAN_POINT('Ctrl Pts',(2.03091336214401,-1.,0.533108355132905));
#28685=CARTESIAN_POINT('Ctrl Pts',(2.03091336214401,1.,0.533108355132905));
#28686=CARTESIAN_POINT('Ctrl Pts',(2.02618329083289,-1.,0.528997127241911));
#28687=CARTESIAN_POINT('Ctrl Pts',(2.02618329083289,1.,0.528997127241911));
#28688=CARTESIAN_POINT('Ctrl Pts',(2.02143356304712,-1.,0.524925318333519));
#28689=CARTESIAN_POINT('Ctrl Pts',(2.02143356304712,1.,0.524925318333519));
#28690=CARTESIAN_POINT('Ctrl Pts',(2.01666477917305,-1.,0.520893590399429));
#28691=CARTESIAN_POINT('Ctrl Pts',(2.01666477917305,1.,0.520893590399429));
#28692=CARTESIAN_POINT('Ctrl Pts',(2.01187773939257,-1.,0.516902681728733));
#28693=CARTESIAN_POINT('Ctrl Pts',(2.01187773939257,1.,0.516902681728733));
#28694=CARTESIAN_POINT('Ctrl Pts',(2.00707309946955,-1.,0.512953306961814));
#28695=CARTESIAN_POINT('Ctrl Pts',(2.00707309946955,1.,0.512953306961814));
#28696=CARTESIAN_POINT('Ctrl Pts',(2.00225107134733,-1.,0.509046069886152));
#28697=CARTESIAN_POINT('Ctrl Pts',(2.00225107134733,1.,0.509046069886152));
#28698=CARTESIAN_POINT('Ctrl Pts',(1.99741107463567,-1.,0.505181361323011));
#28699=CARTESIAN_POINT('Ctrl Pts',(1.99741107463567,1.,0.505181361323011));
#28700=CARTESIAN_POINT('Ctrl Pts',(1.9925514912615,-1.,0.501359287727129));
#28701=CARTESIAN_POINT('Ctrl Pts',(1.9925514912615,1.,0.501359287727129));
#28702=CARTESIAN_POINT('Ctrl Pts',(1.98767044752929,-1.,0.497579909545564));
#28703=CARTESIAN_POINT('Ctrl Pts',(1.98767044752929,1.,0.497579909545564));
#28704=CARTESIAN_POINT('Ctrl Pts',(1.9827665876182,-1.,0.493843476541493));
#28705=CARTESIAN_POINT('Ctrl Pts',(1.9827665876182,1.,0.493843476541493));
#28706=CARTESIAN_POINT('Ctrl Pts',(1.97783973019229,-1.,0.490150627860955));
#28707=CARTESIAN_POINT('Ctrl Pts',(1.97783973019229,1.,0.490150627860955));
#28708=CARTESIAN_POINT('Ctrl Pts',(1.97289186263272,-1.,0.486502692907661));
#28709=CARTESIAN_POINT('Ctrl Pts',(1.97289186263272,1.,0.486502692907661));
#28710=CARTESIAN_POINT('Ctrl Pts',(1.96792703422358,-1.,0.482901662120687));
#28711=CARTESIAN_POINT('Ctrl Pts',(1.96792703422358,1.,0.482901662120687));
#28712=CARTESIAN_POINT('Ctrl Pts',(1.96294933055938,-1.,0.479349583074846));
#28713=CARTESIAN_POINT('Ctrl Pts',(1.96294933055938,1.,0.479349583074846));
#28714=CARTESIAN_POINT('Ctrl Pts',(1.95796111148175,-1.,0.475848034683172));
#28715=CARTESIAN_POINT('Ctrl Pts',(1.95796111148175,1.,0.475848034683172));
#28716=CARTESIAN_POINT('Ctrl Pts',(1.95296148278136,-1.,0.47239767226408));
#28717=CARTESIAN_POINT('Ctrl Pts',(1.95296148278136,1.,0.47239767226408));
#28718=CARTESIAN_POINT('Ctrl Pts',(1.94794381136524,-1.,0.468997482913158));
#28719=CARTESIAN_POINT('Ctrl Pts',(1.94794381136524,1.,0.468997482913158));
#28720=CARTESIAN_POINT('Ctrl Pts',(1.94289794196205,-1.,0.465645462026065));
#28721=CARTESIAN_POINT('Ctrl Pts',(1.94289794196205,1.,0.465645462026065));
#28722=CARTESIAN_POINT('Ctrl Pts',(1.93781486640834,-1.,0.462340031009087));
#28723=CARTESIAN_POINT('Ctrl Pts',(1.93781486640834,1.,0.462340031009087));
#28724=CARTESIAN_POINT('Ctrl Pts',(1.93269066517936,-1.,0.459081234547932));
#28725=CARTESIAN_POINT('Ctrl Pts',(1.93269066517936,1.,0.459081234547932));
#28726=CARTESIAN_POINT('Ctrl Pts',(1.92753067150461,-1.,0.455872005174336));
#28727=CARTESIAN_POINT('Ctrl Pts',(1.92753067150461,1.,0.455872005174336));
#28728=CARTESIAN_POINT('Ctrl Pts',(1.9223538064847,-1.,0.452719478359356));
#28729=CARTESIAN_POINT('Ctrl Pts',(1.9223538064847,1.,0.452719478359356));
#28730=CARTESIAN_POINT('Ctrl Pts',(1.91718342555717,-1.,0.449632260106572));
#28731=CARTESIAN_POINT('Ctrl Pts',(1.91718342555717,1.,0.449632260106572));
#28732=CARTESIAN_POINT('Ctrl Pts',(1.91203699981095,-1.,0.446617343485651));
#28733=CARTESIAN_POINT('Ctrl Pts',(1.91203699981095,1.,0.446617343485651));
#28734=CARTESIAN_POINT('Ctrl Pts',(1.90691756144906,-1.,0.443677556849171));
#28735=CARTESIAN_POINT('Ctrl Pts',(1.90691756144906,1.,0.443677556849171));
#28736=CARTESIAN_POINT('Ctrl Pts',(1.90180124389137,-1.,0.440807833704161));
#28737=CARTESIAN_POINT('Ctrl Pts',(1.90180124389137,1.,0.440807833704161));
#28738=CARTESIAN_POINT('Ctrl Pts',(1.89663648956549,-1.,0.437995003948443));
#28739=CARTESIAN_POINT('Ctrl Pts',(1.89663648956549,1.,0.437995003948443));
#28740=CARTESIAN_POINT('Ctrl Pts',(1.89136993975585,-1.,0.43522566096358));
#28741=CARTESIAN_POINT('Ctrl Pts',(1.89136993975585,1.,0.43522566096358));
#28742=CARTESIAN_POINT('Ctrl Pts',(1.88596913666828,-1.,0.432493038548833));
#28743=CARTESIAN_POINT('Ctrl Pts',(1.88596913666828,1.,0.432493038548833));
#28744=CARTESIAN_POINT('Ctrl Pts',(1.88044229001778,-1.,0.429803062482217));
#28745=CARTESIAN_POINT('Ctrl Pts',(1.88044229001778,1.,0.429803062482217));
#28746=CARTESIAN_POINT('Ctrl Pts',(1.87486989291333,-1.,0.427183828518743));
#28747=CARTESIAN_POINT('Ctrl Pts',(1.87486989291333,1.,0.427183828518743));
#28748=CARTESIAN_POINT('Ctrl Pts',(1.8693780394412,-1.,0.424678177290876));
#28749=CARTESIAN_POINT('Ctrl Pts',(1.8693780394412,1.,0.424678177290876));
#28750=CARTESIAN_POINT('Ctrl Pts',(1.86408083333863,-1.,0.422327307417885));
#28751=CARTESIAN_POINT('Ctrl Pts',(1.86408083333863,1.,0.422327307417885));
#28752=CARTESIAN_POINT('Ctrl Pts',(1.8590328109667,-1.,0.420157287975583));
#28753=CARTESIAN_POINT('Ctrl Pts',(1.8590328109667,1.,0.420157287975583));
#28754=CARTESIAN_POINT('Ctrl Pts',(1.8541763285645,-1.,0.418164129144046));
#28755=CARTESIAN_POINT('Ctrl Pts',(1.8541763285645,1.,0.418164129144046));
#28756=CARTESIAN_POINT('Ctrl Pts',(1.84929312930314,-1.,0.416300022039885));
#28757=CARTESIAN_POINT('Ctrl Pts',(1.84929312930314,1.,0.416300022039885));
#28758=CARTESIAN_POINT('Ctrl Pts',(1.84405757074218,-1.,0.414487438255542));
#28759=CARTESIAN_POINT('Ctrl Pts',(1.84405757074218,1.,0.414487438255542));
#28760=CARTESIAN_POINT('Ctrl Pts',(1.8380895347617,-1.,0.412633125322945));
#28761=CARTESIAN_POINT('Ctrl Pts',(1.8380895347617,1.,0.412633125322945));
#28762=CARTESIAN_POINT('Ctrl Pts',(1.83100408895047,-1.,0.410641256301276));
#28763=CARTESIAN_POINT('Ctrl Pts',(1.83100408895047,1.,0.410641256301276));
#28764=CARTESIAN_POINT('Ctrl Pts',(1.82247022677562,-1.,0.408428948106228));
#28765=CARTESIAN_POINT('Ctrl Pts',(1.82247022677562,1.,0.408428948106228));
#28766=CARTESIAN_POINT('Ctrl Pts',(1.81223801812013,-1.,0.405933518407176));
#28767=CARTESIAN_POINT('Ctrl Pts',(1.81223801812013,1.,0.405933518407176));
#28768=CARTESIAN_POINT('Ctrl Pts',(1.80012077173238,-1.,0.403107976163396));
#28769=CARTESIAN_POINT('Ctrl Pts',(1.80012077173238,1.,0.403107976163396));
#28770=CARTESIAN_POINT('Ctrl Pts',(1.78598826343754,-1.,0.399919403774156));
#28771=CARTESIAN_POINT('Ctrl Pts',(1.78598826343754,1.,0.399919403774156));
#28772=CARTESIAN_POINT('Ctrl Pts',(1.76975560043442,-1.,0.396346196110688));
#28773=CARTESIAN_POINT('Ctrl Pts',(1.76975560043442,1.,0.396346196110688));
#28774=CARTESIAN_POINT('Ctrl Pts',(1.75137405310193,-1.,0.392375812285396));
#28775=CARTESIAN_POINT('Ctrl Pts',(1.75137405310193,1.,0.392375812285396));
#28776=CARTESIAN_POINT('Ctrl Pts',(1.73493170972829,-1.,0.388877023502615));
#28777=CARTESIAN_POINT('Ctrl Pts',(1.73493170972829,1.,0.388877023502615));
#28778=CARTESIAN_POINT('Ctrl Pts',(1.72162022244582,-1.,0.386070790323281));
#28779=CARTESIAN_POINT('Ctrl Pts',(1.72162022244582,1.,0.386070790323281));
#28780=CARTESIAN_POINT('Ctrl Pts',(1.71231062891398,-1.,0.384119047314215));
#28781=CARTESIAN_POINT('Ctrl Pts',(1.71231062891398,1.,0.384119047314215));
#28782=CARTESIAN_POINT('Ctrl Pts',(1.7075470150345,-1.,0.383122945602004));
#28783=CARTESIAN_POINT('Ctrl Pts',(1.7075470150345,1.,0.383122945602004));
#28784=CARTESIAN_POINT('',(1.7075470150345,1.,0.383122945602004));
#28785=CARTESIAN_POINT('',(1.7075470150345,0.,0.383122945602005));
#28786=CARTESIAN_POINT('',(2.11275013067528,1.,0.613422273260091));
#28787=CARTESIAN_POINT('Ctrl Pts',(2.11275013067528,1.,0.613422273260091));
#28788=CARTESIAN_POINT('Ctrl Pts',(2.11187554260142,1.,0.61246736556225));
#28789=CARTESIAN_POINT('Ctrl Pts',(2.11012443807661,1.,0.610560911691114));
#28790=CARTESIAN_POINT('Ctrl Pts',(2.10749199615859,1.,0.607711315456826));
#28791=CARTESIAN_POINT('Ctrl Pts',(2.10397049887709,1.,0.603932030738212));
#28792=CARTESIAN_POINT('Ctrl Pts',(2.09954930865331,1.,0.599241616422144));
#28793=CARTESIAN_POINT('Ctrl Pts',(2.09510876220501,1.,0.594585006052824));
#28794=CARTESIAN_POINT('Ctrl Pts',(2.09064881812053,1.,0.58996236540319));
#28795=CARTESIAN_POINT('Ctrl Pts',(2.086169437277,1.,0.585373918990895));
#28796=CARTESIAN_POINT('Ctrl Pts',(2.08167059018138,1.,0.580819952107257));
#28797=CARTESIAN_POINT('Ctrl Pts',(2.07715226767361,1.,0.576300797416275));
#28798=CARTESIAN_POINT('Ctrl Pts',(2.07261449292757,1.,0.571816823242411));
#28799=CARTESIAN_POINT('Ctrl Pts',(2.06805732997383,1.,0.56736842118123));
#28800=CARTESIAN_POINT('Ctrl Pts',(2.06348090160697,1.,0.562955993082574));
#28801=CARTESIAN_POINT('Ctrl Pts',(2.05888537756571,1.,0.558579940185468));
#28802=CARTESIAN_POINT('Ctrl Pts',(2.05427091604482,1.,0.55424065746411));
#28803=CARTESIAN_POINT('Ctrl Pts',(2.04963761077974,1.,0.549938525150342));
#28804=CARTESIAN_POINT('Ctrl Pts',(2.0449854471456,1.,0.545673903817349));
#28805=CARTESIAN_POINT('Ctrl Pts',(2.0403142269048,1.,0.54144712061552));
#28806=CARTESIAN_POINT('Ctrl Pts',(2.03562362953993,1.,0.537258489833135));
#28807=CARTESIAN_POINT('Ctrl Pts',(2.03091336214401,1.,0.533108355132905));
#28808=CARTESIAN_POINT('Ctrl Pts',(2.02618329083289,1.,0.528997127241911));
#28809=CARTESIAN_POINT('Ctrl Pts',(2.02143356304712,1.,0.524925318333519));
#28810=CARTESIAN_POINT('Ctrl Pts',(2.01666477917305,1.,0.520893590399429));
#28811=CARTESIAN_POINT('Ctrl Pts',(2.01187773939257,1.,0.516902681728733));
#28812=CARTESIAN_POINT('Ctrl Pts',(2.00707309946955,1.,0.512953306961814));
#28813=CARTESIAN_POINT('Ctrl Pts',(2.00225107134733,1.,0.509046069886152));
#28814=CARTESIAN_POINT('Ctrl Pts',(1.99741107463567,1.,0.505181361323011));
#28815=CARTESIAN_POINT('Ctrl Pts',(1.9925514912615,1.,0.501359287727129));
#28816=CARTESIAN_POINT('Ctrl Pts',(1.98767044752929,1.,0.497579909545564));
#28817=CARTESIAN_POINT('Ctrl Pts',(1.9827665876182,1.,0.493843476541493));
#28818=CARTESIAN_POINT('Ctrl Pts',(1.97783973019229,1.,0.490150627860955));
#28819=CARTESIAN_POINT('Ctrl Pts',(1.97289186263272,1.,0.486502692907661));
#28820=CARTESIAN_POINT('Ctrl Pts',(1.96792703422358,1.,0.482901662120687));
#28821=CARTESIAN_POINT('Ctrl Pts',(1.96294933055938,1.,0.479349583074846));
#28822=CARTESIAN_POINT('Ctrl Pts',(1.95796111148175,1.,0.475848034683172));
#28823=CARTESIAN_POINT('Ctrl Pts',(1.95296148278136,1.,0.47239767226408));
#28824=CARTESIAN_POINT('Ctrl Pts',(1.94794381136524,1.,0.468997482913158));
#28825=CARTESIAN_POINT('Ctrl Pts',(1.94289794196205,1.,0.465645462026065));
#28826=CARTESIAN_POINT('Ctrl Pts',(1.93781486640834,1.,0.462340031009087));
#28827=CARTESIAN_POINT('Ctrl Pts',(1.93269066517936,1.,0.459081234547932));
#28828=CARTESIAN_POINT('Ctrl Pts',(1.92753067150461,1.,0.455872005174336));
#28829=CARTESIAN_POINT('Ctrl Pts',(1.9223538064847,1.,0.452719478359356));
#28830=CARTESIAN_POINT('Ctrl Pts',(1.91718342555717,1.,0.449632260106572));
#28831=CARTESIAN_POINT('Ctrl Pts',(1.91203699981095,1.,0.446617343485651));
#28832=CARTESIAN_POINT('Ctrl Pts',(1.90691756144906,1.,0.443677556849171));
#28833=CARTESIAN_POINT('Ctrl Pts',(1.90180124389137,1.,0.440807833704161));
#28834=CARTESIAN_POINT('Ctrl Pts',(1.89663648956549,1.,0.437995003948443));
#28835=CARTESIAN_POINT('Ctrl Pts',(1.89136993975585,1.,0.43522566096358));
#28836=CARTESIAN_POINT('Ctrl Pts',(1.88596913666828,1.,0.432493038548833));
#28837=CARTESIAN_POINT('Ctrl Pts',(1.88044229001778,1.,0.429803062482217));
#28838=CARTESIAN_POINT('Ctrl Pts',(1.87486989291333,1.,0.427183828518743));
#28839=CARTESIAN_POINT('Ctrl Pts',(1.8693780394412,1.,0.424678177290876));
#28840=CARTESIAN_POINT('Ctrl Pts',(1.86408083333863,1.,0.422327307417885));
#28841=CARTESIAN_POINT('Ctrl Pts',(1.8590328109667,1.,0.420157287975583));
#28842=CARTESIAN_POINT('Ctrl Pts',(1.8541763285645,1.,0.418164129144046));
#28843=CARTESIAN_POINT('Ctrl Pts',(1.84929312930314,1.,0.416300022039885));
#28844=CARTESIAN_POINT('Ctrl Pts',(1.84405757074218,1.,0.414487438255542));
#28845=CARTESIAN_POINT('Ctrl Pts',(1.8380895347617,1.,0.412633125322945));
#28846=CARTESIAN_POINT('Ctrl Pts',(1.83100408895047,1.,0.410641256301276));
#28847=CARTESIAN_POINT('Ctrl Pts',(1.82247022677562,1.,0.408428948106228));
#28848=CARTESIAN_POINT('Ctrl Pts',(1.81223801812013,1.,0.405933518407176));
#28849=CARTESIAN_POINT('Ctrl Pts',(1.80012077173238,1.,0.403107976163396));
#28850=CARTESIAN_POINT('Ctrl Pts',(1.78598826343754,1.,0.399919403774156));
#28851=CARTESIAN_POINT('Ctrl Pts',(1.76975560043442,1.,0.396346196110688));
#28852=CARTESIAN_POINT('Ctrl Pts',(1.75137405310193,1.,0.392375812285396));
#28853=CARTESIAN_POINT('Ctrl Pts',(1.73493170972829,1.,0.388877023502615));
#28854=CARTESIAN_POINT('Ctrl Pts',(1.72162022244582,1.,0.386070790323281));
#28855=CARTESIAN_POINT('Ctrl Pts',(1.71231062891398,1.,0.384119047314215));
#28856=CARTESIAN_POINT('Ctrl Pts',(1.7075470150345,1.,0.383122945602004));
#28857=CARTESIAN_POINT('',(2.11275013067528,0.,0.613422273260091));
#28858=CARTESIAN_POINT('Origin',(2.0698113262342,0.,0.745574324794401));
#28859=CARTESIAN_POINT('',(2.0698113262342,1.,0.745574324794401));
#28860=CARTESIAN_POINT('',(2.11275013067528,1.,0.613422273260091));
#28861=CARTESIAN_POINT('',(2.0698113262342,0.,0.745574324794401));
#28862=CARTESIAN_POINT('Ctrl Pts',(1.60662857109684,-1.,0.693717979106306));
#28863=CARTESIAN_POINT('Ctrl Pts',(1.60662857109684,1.,0.693717979106306));
#28864=CARTESIAN_POINT('Ctrl Pts',(1.61106790958151,-1.,0.695712097881194));
#28865=CARTESIAN_POINT('Ctrl Pts',(1.61106790958151,1.,0.695712097881194));
#28866=CARTESIAN_POINT('Ctrl Pts',(1.61974673472612,-1.,0.699605146405088));
#28867=CARTESIAN_POINT('Ctrl Pts',(1.61974673472612,1.,0.699605146405088));
#28868=CARTESIAN_POINT('Ctrl Pts',(1.63216541664676,-1.,0.705159151988319));
#28869=CARTESIAN_POINT('Ctrl Pts',(1.63216541664676,1.,0.705159151988319));
#28870=CARTESIAN_POINT('Ctrl Pts',(1.64752408832016,-1.,0.711993139355394));
#28871=CARTESIAN_POINT('Ctrl Pts',(1.64752408832016,1.,0.711993139355394));
#28872=CARTESIAN_POINT('Ctrl Pts',(1.6647288055568,-1.,0.719585433804282));
#28873=CARTESIAN_POINT('Ctrl Pts',(1.6647288055568,1.,0.719585433804282));
#28874=CARTESIAN_POINT('Ctrl Pts',(1.67996158455503,-1.,0.726235967997433));
#28875=CARTESIAN_POINT('Ctrl Pts',(1.67996158455503,1.,0.726235967997433));
#28876=CARTESIAN_POINT('Ctrl Pts',(1.69326921975743,-1.,0.731963238697195));
#28877=CARTESIAN_POINT('Ctrl Pts',(1.69326921975743,1.,0.731963238697195));
#28878=CARTESIAN_POINT('Ctrl Pts',(1.70473309006121,-1.,0.736799665724771));
#28879=CARTESIAN_POINT('Ctrl Pts',(1.70473309006121,1.,0.736799665724771));
#28880=CARTESIAN_POINT('Ctrl Pts',(1.71447789751927,-1.,0.740795162032088));
#28881=CARTESIAN_POINT('Ctrl Pts',(1.71447789751927,1.,0.740795162032088));
#28882=CARTESIAN_POINT('Ctrl Pts',(1.7226822991693,-1.,0.744021445433765));
#28883=CARTESIAN_POINT('Ctrl Pts',(1.7226822991693,1.,0.744021445433765));
#28884=CARTESIAN_POINT('Ctrl Pts',(1.72958533647399,-1.,0.746574710096437));
#28885=CARTESIAN_POINT('Ctrl Pts',(1.72958533647399,1.,0.746574710096437));
#28886=CARTESIAN_POINT('Ctrl Pts',(1.73550351679848,-1.,0.748582462954855));
#28887=CARTESIAN_POINT('Ctrl Pts',(1.73550351679848,1.,0.748582462954855));
#28888=CARTESIAN_POINT('Ctrl Pts',(1.74080458266705,-1.,0.750193435979541));
#28889=CARTESIAN_POINT('Ctrl Pts',(1.74080458266705,1.,0.750193435979541));
#28890=CARTESIAN_POINT('Ctrl Pts',(1.74585086852298,-1.,0.751555614163629));
#28891=CARTESIAN_POINT('Ctrl Pts',(1.74585086852298,1.,0.751555614163629));
#28892=CARTESIAN_POINT('Ctrl Pts',(1.75095139468809,-1.,0.752797683531377));
#28893=CARTESIAN_POINT('Ctrl Pts',(1.75095139468809,1.,0.752797683531377));
#28894=CARTESIAN_POINT('Ctrl Pts',(1.75631083600175,-1.,0.75400925402848));
#28895=CARTESIAN_POINT('Ctrl Pts',(1.75631083600175,1.,0.75400925402848));
#28896=CARTESIAN_POINT('Ctrl Pts',(1.7619781724032,-1.,0.755220979975262));
#28897=CARTESIAN_POINT('Ctrl Pts',(1.7619781724032,1.,0.755220979975262));
#28898=CARTESIAN_POINT('Ctrl Pts',(1.76789396003141,-1.,0.756421896028403));
#28899=CARTESIAN_POINT('Ctrl Pts',(1.76789396003141,1.,0.756421896028403));
#28900=CARTESIAN_POINT('Ctrl Pts',(1.77394167108342,-1.,0.757578264077238));
#28901=CARTESIAN_POINT('Ctrl Pts',(1.77394167108342,1.,0.757578264077238));
#28902=CARTESIAN_POINT('Ctrl Pts',(1.77999411220912,-1.,0.75865062667738));
#28903=CARTESIAN_POINT('Ctrl Pts',(1.77999411220912,1.,0.75865062667738));
#28904=CARTESIAN_POINT('Ctrl Pts',(1.78596964884526,-1.,0.759614401109868));
#28905=CARTESIAN_POINT('Ctrl Pts',(1.78596964884526,1.,0.759614401109868));
#28906=CARTESIAN_POINT('Ctrl Pts',(1.79185815610802,-1.,0.760469555880425));
#28907=CARTESIAN_POINT('Ctrl Pts',(1.79185815610802,1.,0.760469555880425));
#28908=CARTESIAN_POINT('Ctrl Pts',(1.79768986997735,-1.,0.761229695230359));
#28909=CARTESIAN_POINT('Ctrl Pts',(1.79768986997735,1.,0.761229695230359));
#28910=CARTESIAN_POINT('Ctrl Pts',(1.80351583877334,-1.,0.761915336443516));
#28911=CARTESIAN_POINT('Ctrl Pts',(1.80351583877334,1.,0.761915336443516));
#28912=CARTESIAN_POINT('Ctrl Pts',(1.80938551463989,-1.,0.762546129464036));
#28913=CARTESIAN_POINT('Ctrl Pts',(1.80938551463989,1.,0.762546129464036));
#28914=CARTESIAN_POINT('Ctrl Pts',(1.81532118405566,-1.,0.763132003836783));
#28915=CARTESIAN_POINT('Ctrl Pts',(1.81532118405566,1.,0.763132003836783));
#28916=CARTESIAN_POINT('Ctrl Pts',(1.82131873145297,-1.,0.763673465462854));
#28917=CARTESIAN_POINT('Ctrl Pts',(1.82131873145297,1.,0.763673465462854));
#28918=CARTESIAN_POINT('Ctrl Pts',(1.8273599120008,-1.,0.764165902606056));
#28919=CARTESIAN_POINT('Ctrl Pts',(1.8273599120008,1.,0.764165902606056));
#28920=CARTESIAN_POINT('Ctrl Pts',(1.8334207722714,-1.,0.764602549687846));
#28921=CARTESIAN_POINT('Ctrl Pts',(1.8334207722714,1.,0.764602549687846));
#28922=CARTESIAN_POINT('Ctrl Pts',(1.83948181064823,-1.,0.764978057881688));
#28923=CARTESIAN_POINT('Ctrl Pts',(1.83948181064823,1.,0.764978057881688));
#28924=CARTESIAN_POINT('Ctrl Pts',(1.8455369887591,-1.,0.765291664861972));
#28925=CARTESIAN_POINT('Ctrl Pts',(1.8455369887591,1.,0.765291664861972));
#28926=CARTESIAN_POINT('Ctrl Pts',(1.85158945130054,-1.,0.765545710619023));
#28927=CARTESIAN_POINT('Ctrl Pts',(1.85158945130054,1.,0.765545710619023));
#28928=CARTESIAN_POINT('Ctrl Pts',(1.85764741390391,-1.,0.765744212909305));
#28929=CARTESIAN_POINT('Ctrl Pts',(1.85764741390391,1.,0.765744212909305));
#28930=CARTESIAN_POINT('Ctrl Pts',(1.86372027063314,-1.,0.765891519092557));
#28931=CARTESIAN_POINT('Ctrl Pts',(1.86372027063314,1.,0.765891519092557));
#28932=CARTESIAN_POINT('Ctrl Pts',(1.86981398314345,-1.,0.765990708546112));
#28933=CARTESIAN_POINT('Ctrl Pts',(1.86981398314345,1.,0.765990708546112));
#28934=CARTESIAN_POINT('Ctrl Pts',(1.87592888967886,-1.,0.766042837036759));
#28935=CARTESIAN_POINT('Ctrl Pts',(1.87592888967886,1.,0.766042837036759));
#28936=CARTESIAN_POINT('Ctrl Pts',(1.88206215302561,-1.,0.766047794851869));
#28937=CARTESIAN_POINT('Ctrl Pts',(1.88206215302561,1.,0.766047794851869));
#28938=CARTESIAN_POINT('Ctrl Pts',(1.88820926433409,-1.,0.76600483706209));
#28939=CARTESIAN_POINT('Ctrl Pts',(1.88820926433409,1.,0.76600483706209));
#28940=CARTESIAN_POINT('Ctrl Pts',(1.89436577771389,-1.,0.765913193856979));
#28941=CARTESIAN_POINT('Ctrl Pts',(1.89436577771389,1.,0.765913193856979));
#28942=CARTESIAN_POINT('Ctrl Pts',(1.90052930393599,-1.,0.765772772593395));
#28943=CARTESIAN_POINT('Ctrl Pts',(1.90052930393599,1.,0.765772772593395));
#28944=CARTESIAN_POINT('Ctrl Pts',(1.90669961402362,-1.,0.765584196937937));
#28945=CARTESIAN_POINT('Ctrl Pts',(1.90669961402362,1.,0.765584196937937));
#28946=CARTESIAN_POINT('Ctrl Pts',(1.91287765805174,-1.,0.765348465884739));
#28947=CARTESIAN_POINT('Ctrl Pts',(1.91287765805174,1.,0.765348465884739));
#28948=CARTESIAN_POINT('Ctrl Pts',(1.91906491634197,-1.,0.765066729667095));
#28949=CARTESIAN_POINT('Ctrl Pts',(1.91906491634197,1.,0.765066729667095));
#28950=CARTESIAN_POINT('Ctrl Pts',(1.92526263537041,-1.,0.764740025488189));
#28951=CARTESIAN_POINT('Ctrl Pts',(1.92526263537041,1.,0.764740025488189));
#28952=CARTESIAN_POINT('Ctrl Pts',(1.93147105496367,-1.,0.76436901067389));
#28953=CARTESIAN_POINT('Ctrl Pts',(1.93147105496367,1.,0.76436901067389));
#28954=CARTESIAN_POINT('Ctrl Pts',(1.93768964875867,-1.,0.763954049121394));
#28955=CARTESIAN_POINT('Ctrl Pts',(1.93768964875867,1.,0.763954049121394));
#28956=CARTESIAN_POINT('Ctrl Pts',(1.94391746617626,-1.,0.763495333538581));
#28957=CARTESIAN_POINT('Ctrl Pts',(1.94391746617626,1.,0.763495333538581));
#28958=CARTESIAN_POINT('Ctrl Pts',(1.95015342590025,-1.,0.762992990878774));
#28959=CARTESIAN_POINT('Ctrl Pts',(1.95015342590025,1.,0.762992990878774));
#28960=CARTESIAN_POINT('Ctrl Pts',(1.95639665309893,-1.,0.762447203806264));
#28961=CARTESIAN_POINT('Ctrl Pts',(1.95639665309893,1.,0.762447203806264));
#28962=CARTESIAN_POINT('Ctrl Pts',(1.96264672744229,-1.,0.761858300014575));
#28963=CARTESIAN_POINT('Ctrl Pts',(1.96264672744229,1.,0.761858300014575));
#28964=CARTESIAN_POINT('Ctrl Pts',(1.96890351582545,-1.,0.761226690483986));
#28965=CARTESIAN_POINT('Ctrl Pts',(1.96890351582545,1.,0.761226690483986));
#28966=CARTESIAN_POINT('Ctrl Pts',(1.97516705321521,-1.,0.760552825409856));
#28967=CARTESIAN_POINT('Ctrl Pts',(1.97516705321521,1.,0.760552825409856));
#28968=CARTESIAN_POINT('Ctrl Pts',(1.98143741418156,-1.,0.759837147452135));
#28969=CARTESIAN_POINT('Ctrl Pts',(1.98143741418156,1.,0.759837147452135));
#28970=CARTESIAN_POINT('Ctrl Pts',(1.98771456680806,-1.,0.759080037802243));
#28971=CARTESIAN_POINT('Ctrl Pts',(1.98771456680806,1.,0.759080037802243));
#28972=CARTESIAN_POINT('Ctrl Pts',(1.9939983109871,-1.,0.758281796766377));
#28973=CARTESIAN_POINT('Ctrl Pts',(1.9939983109871,1.,0.758281796766377));
#28974=CARTESIAN_POINT('Ctrl Pts',(2.00028834739072,-1.,0.757442676862342));
#28975=CARTESIAN_POINT('Ctrl Pts',(2.00028834739072,1.,0.757442676862342));
#28976=CARTESIAN_POINT('Ctrl Pts',(2.00658431587682,-1.,0.756562904646496));
#28977=CARTESIAN_POINT('Ctrl Pts',(2.00658431587682,1.,0.756562904646496));
#28978=CARTESIAN_POINT('Ctrl Pts',(2.01288584328149,-1.,0.755642704958101));
#28979=CARTESIAN_POINT('Ctrl Pts',(2.01288584328149,1.,0.755642704958101));
#28980=CARTESIAN_POINT('Ctrl Pts',(2.01919259406003,-1.,0.75468233072352));
#28981=CARTESIAN_POINT('Ctrl Pts',(2.01919259406003,1.,0.75468233072352));
#28982=CARTESIAN_POINT('Ctrl Pts',(2.02550428623587,-1.,0.753682061113766));
#28983=CARTESIAN_POINT('Ctrl Pts',(2.02550428623587,1.,0.753682061113766));
#28984=CARTESIAN_POINT('Ctrl Pts',(2.03182068456467,-1.,0.752642180488104));
#28985=CARTESIAN_POINT('Ctrl Pts',(2.03182068456467,1.,0.752642180488104));
#28986=CARTESIAN_POINT('Ctrl Pts',(2.03814160092173,-1.,0.751562963361384));
#28987=CARTESIAN_POINT('Ctrl Pts',(2.03814160092173,1.,0.751562963361384));
#28988=CARTESIAN_POINT('Ctrl Pts',(2.04446689147754,-1.,0.750444657874758));
#28989=CARTESIAN_POINT('Ctrl Pts',(2.04446689147754,1.,0.750444657874758));
#28990=CARTESIAN_POINT('Ctrl Pts',(2.05079645591606,-1.,0.749287468663053));
#28991=CARTESIAN_POINT('Ctrl Pts',(2.05079645591606,1.,0.749287468663053));
#28992=CARTESIAN_POINT('Ctrl Pts',(2.05713023030263,-1.,0.748091554181101));
#28993=CARTESIAN_POINT('Ctrl Pts',(2.05713023030263,1.,0.748091554181101));
#28994=CARTESIAN_POINT('Ctrl Pts',(2.06220058927162,-1.,0.747103932785504));
#28995=CARTESIAN_POINT('Ctrl Pts',(2.06220058927162,1.,0.747103932785504));
#28996=CARTESIAN_POINT('Ctrl Pts',(2.06600523016401,-1.,0.746345871542696));
#28997=CARTESIAN_POINT('Ctrl Pts',(2.06600523016401,1.,0.746345871542696));
#28998=CARTESIAN_POINT('Ctrl Pts',(2.06854248895575,-1.,0.74583279137781));
#28999=CARTESIAN_POINT('Ctrl Pts',(2.06854248895575,1.,0.74583279137781));
#29000=CARTESIAN_POINT('Ctrl Pts',(2.0698113262342,-1.,0.745574324794401));
#29001=CARTESIAN_POINT('Ctrl Pts',(2.0698113262342,1.,0.745574324794401));
#29002=CARTESIAN_POINT('',(1.60662857109684,1.,0.693717979106306));
#29003=CARTESIAN_POINT('Ctrl Pts',(1.60662857109684,1.,0.693717979106306));
#29004=CARTESIAN_POINT('Ctrl Pts',(1.61106790958151,1.,0.695712097881194));
#29005=CARTESIAN_POINT('Ctrl Pts',(1.61974673472612,1.,0.699605146405088));
#29006=CARTESIAN_POINT('Ctrl Pts',(1.63216541664676,1.,0.705159151988319));
#29007=CARTESIAN_POINT('Ctrl Pts',(1.64752408832016,1.,0.711993139355394));
#29008=CARTESIAN_POINT('Ctrl Pts',(1.6647288055568,1.,0.719585433804282));
#29009=CARTESIAN_POINT('Ctrl Pts',(1.67996158455503,1.,0.726235967997433));
#29010=CARTESIAN_POINT('Ctrl Pts',(1.69326921975743,1.,0.731963238697195));
#29011=CARTESIAN_POINT('Ctrl Pts',(1.70473309006121,1.,0.736799665724771));
#29012=CARTESIAN_POINT('Ctrl Pts',(1.71447789751927,1.,0.740795162032088));
#29013=CARTESIAN_POINT('Ctrl Pts',(1.7226822991693,1.,0.744021445433765));
#29014=CARTESIAN_POINT('Ctrl Pts',(1.72958533647399,1.,0.746574710096437));
#29015=CARTESIAN_POINT('Ctrl Pts',(1.73550351679848,1.,0.748582462954855));
#29016=CARTESIAN_POINT('Ctrl Pts',(1.74080458266705,1.,0.750193435979541));
#29017=CARTESIAN_POINT('Ctrl Pts',(1.74585086852298,1.,0.751555614163629));
#29018=CARTESIAN_POINT('Ctrl Pts',(1.75095139468809,1.,0.752797683531377));
#29019=CARTESIAN_POINT('Ctrl Pts',(1.75631083600175,1.,0.75400925402848));
#29020=CARTESIAN_POINT('Ctrl Pts',(1.7619781724032,1.,0.755220979975262));
#29021=CARTESIAN_POINT('Ctrl Pts',(1.76789396003141,1.,0.756421896028403));
#29022=CARTESIAN_POINT('Ctrl Pts',(1.77394167108342,1.,0.757578264077238));
#29023=CARTESIAN_POINT('Ctrl Pts',(1.77999411220912,1.,0.75865062667738));
#29024=CARTESIAN_POINT('Ctrl Pts',(1.78596964884526,1.,0.759614401109868));
#29025=CARTESIAN_POINT('Ctrl Pts',(1.79185815610802,1.,0.760469555880425));
#29026=CARTESIAN_POINT('Ctrl Pts',(1.79768986997735,1.,0.761229695230359));
#29027=CARTESIAN_POINT('Ctrl Pts',(1.80351583877334,1.,0.761915336443516));
#29028=CARTESIAN_POINT('Ctrl Pts',(1.80938551463989,1.,0.762546129464036));
#29029=CARTESIAN_POINT('Ctrl Pts',(1.81532118405566,1.,0.763132003836783));
#29030=CARTESIAN_POINT('Ctrl Pts',(1.82131873145297,1.,0.763673465462854));
#29031=CARTESIAN_POINT('Ctrl Pts',(1.8273599120008,1.,0.764165902606056));
#29032=CARTESIAN_POINT('Ctrl Pts',(1.8334207722714,1.,0.764602549687846));
#29033=CARTESIAN_POINT('Ctrl Pts',(1.83948181064823,1.,0.764978057881688));
#29034=CARTESIAN_POINT('Ctrl Pts',(1.8455369887591,1.,0.765291664861972));
#29035=CARTESIAN_POINT('Ctrl Pts',(1.85158945130054,1.,0.765545710619023));
#29036=CARTESIAN_POINT('Ctrl Pts',(1.85764741390391,1.,0.765744212909305));
#29037=CARTESIAN_POINT('Ctrl Pts',(1.86372027063314,1.,0.765891519092557));
#29038=CARTESIAN_POINT('Ctrl Pts',(1.86981398314345,1.,0.765990708546112));
#29039=CARTESIAN_POINT('Ctrl Pts',(1.87592888967886,1.,0.766042837036759));
#29040=CARTESIAN_POINT('Ctrl Pts',(1.88206215302561,1.,0.766047794851869));
#29041=CARTESIAN_POINT('Ctrl Pts',(1.88820926433409,1.,0.76600483706209));
#29042=CARTESIAN_POINT('Ctrl Pts',(1.89436577771389,1.,0.765913193856979));
#29043=CARTESIAN_POINT('Ctrl Pts',(1.90052930393599,1.,0.765772772593395));
#29044=CARTESIAN_POINT('Ctrl Pts',(1.90669961402362,1.,0.765584196937937));
#29045=CARTESIAN_POINT('Ctrl Pts',(1.91287765805174,1.,0.765348465884739));
#29046=CARTESIAN_POINT('Ctrl Pts',(1.91906491634197,1.,0.765066729667095));
#29047=CARTESIAN_POINT('Ctrl Pts',(1.92526263537041,1.,0.764740025488189));
#29048=CARTESIAN_POINT('Ctrl Pts',(1.93147105496367,1.,0.76436901067389));
#29049=CARTESIAN_POINT('Ctrl Pts',(1.93768964875867,1.,0.763954049121394));
#29050=CARTESIAN_POINT('Ctrl Pts',(1.94391746617626,1.,0.763495333538581));
#29051=CARTESIAN_POINT('Ctrl Pts',(1.95015342590025,1.,0.762992990878774));
#29052=CARTESIAN_POINT('Ctrl Pts',(1.95639665309893,1.,0.762447203806264));
#29053=CARTESIAN_POINT('Ctrl Pts',(1.96264672744229,1.,0.761858300014575));
#29054=CARTESIAN_POINT('Ctrl Pts',(1.96890351582545,1.,0.761226690483986));
#29055=CARTESIAN_POINT('Ctrl Pts',(1.97516705321521,1.,0.760552825409856));
#29056=CARTESIAN_POINT('Ctrl Pts',(1.98143741418156,1.,0.759837147452135));
#29057=CARTESIAN_POINT('Ctrl Pts',(1.98771456680806,1.,0.759080037802243));
#29058=CARTESIAN_POINT('Ctrl Pts',(1.9939983109871,1.,0.758281796766377));
#29059=CARTESIAN_POINT('Ctrl Pts',(2.00028834739072,1.,0.757442676862342));
#29060=CARTESIAN_POINT('Ctrl Pts',(2.00658431587682,1.,0.756562904646496));
#29061=CARTESIAN_POINT('Ctrl Pts',(2.01288584328149,1.,0.755642704958101));
#29062=CARTESIAN_POINT('Ctrl Pts',(2.01919259406003,1.,0.75468233072352));
#29063=CARTESIAN_POINT('Ctrl Pts',(2.02550428623587,1.,0.753682061113766));
#29064=CARTESIAN_POINT('Ctrl Pts',(2.03182068456467,1.,0.752642180488104));
#29065=CARTESIAN_POINT('Ctrl Pts',(2.03814160092173,1.,0.751562963361384));
#29066=CARTESIAN_POINT('Ctrl Pts',(2.04446689147754,1.,0.750444657874758));
#29067=CARTESIAN_POINT('Ctrl Pts',(2.05079645591606,1.,0.749287468663053));
#29068=CARTESIAN_POINT('Ctrl Pts',(2.05713023030263,1.,0.748091554181101));
#29069=CARTESIAN_POINT('Ctrl Pts',(2.06220058927162,1.,0.747103932785504));
#29070=CARTESIAN_POINT('Ctrl Pts',(2.06600523016401,1.,0.746345871542696));
#29071=CARTESIAN_POINT('Ctrl Pts',(2.06854248895575,1.,0.74583279137781));
#29072=CARTESIAN_POINT('Ctrl Pts',(2.0698113262342,1.,0.745574324794401));
#29073=CARTESIAN_POINT('',(1.60662857109684,0.,0.693717979106305));
#29074=CARTESIAN_POINT('Origin',(0.,0.,0.));
#29075=CARTESIAN_POINT('',(1.5055822144029,1.,0.892032620296856));
#29076=CARTESIAN_POINT('Origin',(0.,1.,0.));
#29077=CARTESIAN_POINT('',(1.5055822144029,0.,0.892032620296855));
#29078=CARTESIAN_POINT('Ctrl Pts',(1.81978687191668,-1.,1.23627494547115));
#29079=CARTESIAN_POINT('Ctrl Pts',(1.81978687191668,1.,1.23627494547115));
#29080=CARTESIAN_POINT('Ctrl Pts',(1.81925017193666,-1.,1.23509651170476));
#29081=CARTESIAN_POINT('Ctrl Pts',(1.81925017193666,1.,1.23509651170476));
#29082=CARTESIAN_POINT('Ctrl Pts',(1.81817389921279,-1.,1.2327422452705));
#29083=CARTESIAN_POINT('Ctrl Pts',(1.81817389921279,1.,1.2327422452705));
#29084=CARTESIAN_POINT('Ctrl Pts',(1.8165508718364,-1.,1.2292186489137));
#29085=CARTESIAN_POINT('Ctrl Pts',(1.8165508718364,1.,1.2292186489137));
#29086=CARTESIAN_POINT('Ctrl Pts',(1.81436959210434,-1.,1.2245361330495));
#29087=CARTESIAN_POINT('Ctrl Pts',(1.81436959210434,1.,1.2245361330495));
#29088=CARTESIAN_POINT('Ctrl Pts',(1.81161420806656,-1.,1.21870906103557));
#29089=CARTESIAN_POINT('Ctrl Pts',(1.81161420806656,1.,1.21870906103557));
#29090=CARTESIAN_POINT('Ctrl Pts',(1.80882996917129,-1.,1.21290815708314));
#29091=CARTESIAN_POINT('Ctrl Pts',(1.80882996917129,1.,1.21290815708314));
#29092=CARTESIAN_POINT('Ctrl Pts',(1.80601678480707,-1.,1.20713356605475));
#29093=CARTESIAN_POINT('Ctrl Pts',(1.80601678480707,1.,1.20713356605475));
#29094=CARTESIAN_POINT('Ctrl Pts',(1.80317454838603,-1.,1.20138548938974));
#29095=CARTESIAN_POINT('Ctrl Pts',(1.80317454838603,1.,1.20138548938974));
#29096=CARTESIAN_POINT('Ctrl Pts',(1.80030314369879,-1.,1.19566418930242));
#29097=CARTESIAN_POINT('Ctrl Pts',(1.80030314369879,1.,1.19566418930242));
#29098=CARTESIAN_POINT('Ctrl Pts',(1.79740245923478,-1.,1.18996997934445));
#29099=CARTESIAN_POINT('Ctrl Pts',(1.79740245923478,1.,1.18996997934445));
#29100=CARTESIAN_POINT('Ctrl Pts',(1.79447240321515,-1.,1.18430321697432));
#29101=CARTESIAN_POINT('Ctrl Pts',(1.79447240321515,1.,1.18430321697432));
#29102=CARTESIAN_POINT('Ctrl Pts',(1.79151291552689,-1.,1.17866429440809));
#29103=CARTESIAN_POINT('Ctrl Pts',(1.79151291552689,1.,1.17866429440809));
#29104=CARTESIAN_POINT('Ctrl Pts',(1.78852398877616,-1.,1.17305363177328));
#29105=CARTESIAN_POINT('Ctrl Pts',(1.78852398877616,1.,1.17305363177328));
#29106=CARTESIAN_POINT('Ctrl Pts',(1.78550566040443,-1.,1.16747166312303));
#29107=CARTESIAN_POINT('Ctrl Pts',(1.78550566040443,1.,1.16747166312303));
#29108=CARTESIAN_POINT('Ctrl Pts',(1.78245795881009,-1.,1.16191881298499));
#29109=CARTESIAN_POINT('Ctrl Pts',(1.78245795881009,1.,1.16191881298499));
#29110=CARTESIAN_POINT('Ctrl Pts',(1.77938085564275,-1.,1.15639547194698));
#29111=CARTESIAN_POINT('Ctrl Pts',(1.77938085564275,1.,1.15639547194698));
#29112=CARTESIAN_POINT('Ctrl Pts',(1.7762742255701,-1.,1.15090197841515));
#29113=CARTESIAN_POINT('Ctrl Pts',(1.7762742255701,1.,1.15090197841515));
#29114=CARTESIAN_POINT('Ctrl Pts',(1.77313777896194,-1.,1.1454385822692));
#29115=CARTESIAN_POINT('Ctrl Pts',(1.77313777896194,1.,1.1454385822692));
#29116=CARTESIAN_POINT('Ctrl Pts',(1.76997111386769,-1.,1.14000548336975));
#29117=CARTESIAN_POINT('Ctrl Pts',(1.76997111386769,1.,1.14000548336975));
#29118=CARTESIAN_POINT('Ctrl Pts',(1.76677384551862,-1.,1.1346029180462));
#29119=CARTESIAN_POINT('Ctrl Pts',(1.76677384551862,1.,1.1346029180462));
#29120=CARTESIAN_POINT('Ctrl Pts',(1.7635457196617,-1.,1.12923123555075));
#29121=CARTESIAN_POINT('Ctrl Pts',(1.7635457196617,1.,1.12923123555075));
#29122=CARTESIAN_POINT('Ctrl Pts',(1.76028671825096,-1.,1.12389096855086));
#29123=CARTESIAN_POINT('Ctrl Pts',(1.76028671825096,1.,1.12389096855086));
#29124=CARTESIAN_POINT('Ctrl Pts',(1.75699720772105,-1.,1.11858293216763));
#29125=CARTESIAN_POINT('Ctrl Pts',(1.75699720772105,1.,1.11858293216763));
#29126=CARTESIAN_POINT('Ctrl Pts',(1.7536777209463,-1.,1.11330807582551));
#29127=CARTESIAN_POINT('Ctrl Pts',(1.7536777209463,1.,1.11330807582551));
#29128=CARTESIAN_POINT('Ctrl Pts',(1.7503286607592,-1.,1.10806728183007));
#29129=CARTESIAN_POINT('Ctrl Pts',(1.7503286607592,1.,1.10806728183007));
#29130=CARTESIAN_POINT('Ctrl Pts',(1.74695004214923,-1.,1.10286118991143));
#29131=CARTESIAN_POINT('Ctrl Pts',(1.74695004214923,1.,1.10286118991143));
#29132=CARTESIAN_POINT('Ctrl Pts',(1.74354119236208,-1.,1.09768999241226));
#29133=CARTESIAN_POINT('Ctrl Pts',(1.74354119236208,1.,1.09768999241226));
#29134=CARTESIAN_POINT('Ctrl Pts',(1.74010053962247,-1.,1.09255329056493));
#29135=CARTESIAN_POINT('Ctrl Pts',(1.74010053962247,1.,1.09255329056493));
#29136=CARTESIAN_POINT('Ctrl Pts',(1.73662628326091,-1.,1.08745056285427));
#29137=CARTESIAN_POINT('Ctrl Pts',(1.73662628326091,1.,1.08745056285427));
#29138=CARTESIAN_POINT('Ctrl Pts',(1.73311705663407,-1.,1.08238162784749));
#29139=CARTESIAN_POINT('Ctrl Pts',(1.73311705663407,1.,1.08238162784749));
#29140=CARTESIAN_POINT('Ctrl Pts',(1.72957248977424,-1.,1.0773470373727));
#29141=CARTESIAN_POINT('Ctrl Pts',(1.72957248977424,1.,1.0773470373727));
#29142=CARTESIAN_POINT('Ctrl Pts',(1.72599406198488,-1.,1.07234866990252));
#29143=CARTESIAN_POINT('Ctrl Pts',(1.72599406198488,1.,1.07234866990252));
#29144=CARTESIAN_POINT('Ctrl Pts',(1.72238500928453,-1.,1.06738966975462));
#29145=CARTESIAN_POINT('Ctrl Pts',(1.72238500928453,1.,1.06738966975462));
#29146=CARTESIAN_POINT('Ctrl Pts',(1.71874858456904,-1.,1.06247324680647));
#29147=CARTESIAN_POINT('Ctrl Pts',(1.71874858456904,1.,1.06247324680647));
#29148=CARTESIAN_POINT('Ctrl Pts',(1.7150865442702,-1.,1.05760163192479));
#29149=CARTESIAN_POINT('Ctrl Pts',(1.7150865442702,1.,1.05760163192479));
#29150=CARTESIAN_POINT('Ctrl Pts',(1.71139783543989,-1.,1.05277517202855));
#29151=CARTESIAN_POINT('Ctrl Pts',(1.71139783543989,1.,1.05277517202855));
#29152=CARTESIAN_POINT('Ctrl Pts',(1.70767646263649,-1.,1.04799085404995));
#29153=CARTESIAN_POINT('Ctrl Pts',(1.70767646263649,1.,1.04799085404995));
#29154=CARTESIAN_POINT('Ctrl Pts',(1.70391338707982,-1.,1.04324363334554));
#29155=CARTESIAN_POINT('Ctrl Pts',(1.70391338707982,1.,1.04324363334554));
#29156=CARTESIAN_POINT('Ctrl Pts',(1.70010052930962,-1.,1.03852922490789));
#29157=CARTESIAN_POINT('Ctrl Pts',(1.70010052930962,1.,1.03852922490789));
#29158=CARTESIAN_POINT('Ctrl Pts',(1.69623414782771,-1.,1.03384646003588));
#29159=CARTESIAN_POINT('Ctrl Pts',(1.69623414782771,1.,1.03384646003588));
#29160=CARTESIAN_POINT('Ctrl Pts',(1.69231840863458,-1.,1.02919977579147));
#29161=CARTESIAN_POINT('Ctrl Pts',(1.69231840863458,1.,1.02919977579147));
#29162=CARTESIAN_POINT('Ctrl Pts',(1.68836910178447,-1.,1.02460180535255));
#29163=CARTESIAN_POINT('Ctrl Pts',(1.68836910178447,1.,1.02460180535255));
#29164=CARTESIAN_POINT('Ctrl Pts',(1.68440578021706,-1.,1.02006795074201));
#29165=CARTESIAN_POINT('Ctrl Pts',(1.68440578021706,1.,1.02006795074201));
#29166=CARTESIAN_POINT('Ctrl Pts',(1.68044289894798,-1.,1.01561026162773));
#29167=CARTESIAN_POINT('Ctrl Pts',(1.68044289894798,1.,1.01561026162773));
#29168=CARTESIAN_POINT('Ctrl Pts',(1.67648246776464,-1.,1.01123236493511));
#29169=CARTESIAN_POINT('Ctrl Pts',(1.67648246776464,1.,1.01123236493511));
#29170=CARTESIAN_POINT('Ctrl Pts',(1.67250335383293,-1.,1.00692206696414));
#29171=CARTESIAN_POINT('Ctrl Pts',(1.67250335383293,1.,1.00692206696414));
#29172=CARTESIAN_POINT('Ctrl Pts',(1.66846059277303,-1.,1.00265091003727));
#29173=CARTESIAN_POINT('Ctrl Pts',(1.66846059277303,1.,1.00265091003727));
#29174=CARTESIAN_POINT('Ctrl Pts',(1.66430758030376,-1.,0.998389654952758));
#29175=CARTESIAN_POINT('Ctrl Pts',(1.66430758030376,1.,0.998389654952758));
#29176=CARTESIAN_POINT('Ctrl Pts',(1.66001553809947,-1.,0.994121836661306));
#29177=CARTESIAN_POINT('Ctrl Pts',(1.66001553809947,1.,0.994121836661306));
#29178=CARTESIAN_POINT('Ctrl Pts',(1.65559044289699,-1.,0.989855627854165));
#29179=CARTESIAN_POINT('Ctrl Pts',(1.65559044289699,1.,0.989855627854165));
#29180=CARTESIAN_POINT('Ctrl Pts',(1.65110016612638,-1.,0.985642622920821));
#29181=CARTESIAN_POINT('Ctrl Pts',(1.65110016612638,1.,0.985642622920821));
#29182=CARTESIAN_POINT('Ctrl Pts',(1.64665139190656,-1.,0.981562530939489));
#29183=CARTESIAN_POINT('Ctrl Pts',(1.64665139190656,1.,0.981562530939489));
#29184=CARTESIAN_POINT('Ctrl Pts',(1.64233990826687,-1.,0.977689794119417));
#29185=CARTESIAN_POINT('Ctrl Pts',(1.64233990826687,1.,0.977689794119417));
#29186=CARTESIAN_POINT('Ctrl Pts',(1.63820952658144,-1.,0.974066058287419));
#29187=CARTESIAN_POINT('Ctrl Pts',(1.63820952658144,1.,0.974066058287419));
#29188=CARTESIAN_POINT('Ctrl Pts',(1.63420665729798,-1.,0.970669715997509));
#29189=CARTESIAN_POINT('Ctrl Pts',(1.63420665729798,1.,0.970669715997509));
#29190=CARTESIAN_POINT('Ctrl Pts',(1.63013849959461,-1.,0.967387853230345));
#29191=CARTESIAN_POINT('Ctrl Pts',(1.63013849959461,1.,0.967387853230345));
#29192=CARTESIAN_POINT('Ctrl Pts',(1.62571930670187,-1.,0.964046107040536));
#29193=CARTESIAN_POINT('Ctrl Pts',(1.62571930670187,1.,0.964046107040536));
#29194=CARTESIAN_POINT('Ctrl Pts',(1.62061638140221,-1.,0.960438326101729));
#29195=CARTESIAN_POINT('Ctrl Pts',(1.62061638140221,1.,0.960438326101729));
#29196=CARTESIAN_POINT('Ctrl Pts',(1.61449324337085,-1.,0.956354422920671));
#29197=CARTESIAN_POINT('Ctrl Pts',(1.61449324337085,1.,0.956354422920671));
#29198=CARTESIAN_POINT('Ctrl Pts',(1.60706069896936,-1.,0.951613284356035));
#29199=CARTESIAN_POINT('Ctrl Pts',(1.60706069896936,1.,0.951613284356035));
#29200=CARTESIAN_POINT('Ctrl Pts',(1.59810042043673,-1.,0.946078063315257));
#29201=CARTESIAN_POINT('Ctrl Pts',(1.59810042043673,1.,0.946078063315257));
#29202=CARTESIAN_POINT('Ctrl Pts',(1.58744937487176,-1.,0.939646377893399));
#29203=CARTESIAN_POINT('Ctrl Pts',(1.58744937487176,1.,0.939646377893399));
#29204=CARTESIAN_POINT('Ctrl Pts',(1.57499388382243,-1.,0.932246680108685));
#29205=CARTESIAN_POINT('Ctrl Pts',(1.57499388382243,1.,0.932246680108685));
#29206=CARTESIAN_POINT('Ctrl Pts',(1.56065988578893,-1.,0.923832188944341));
#29207=CARTESIAN_POINT('Ctrl Pts',(1.56065988578893,1.,0.923832188944341));
#29208=CARTESIAN_POINT('Ctrl Pts',(1.54440491149498,-1.,0.914375919026456));
#29209=CARTESIAN_POINT('Ctrl Pts',(1.54440491149498,1.,0.914375919026456));
#29210=CARTESIAN_POINT('Ctrl Pts',(1.52984849887993,-1.,0.905967409625651));
#29211=CARTESIAN_POINT('Ctrl Pts',(1.52984849887993,1.,0.905967409625651));
#29212=CARTESIAN_POINT('Ctrl Pts',(1.51805569590094,-1.,0.899185047483511));
#29213=CARTESIAN_POINT('Ctrl Pts',(1.51805569590094,1.,0.899185047483511));
#29214=CARTESIAN_POINT('Ctrl Pts',(1.50980486806688,-1.,0.894452006964544));
#29215=CARTESIAN_POINT('Ctrl Pts',(1.50980486806688,1.,0.894452006964544));
#29216=CARTESIAN_POINT('Ctrl Pts',(1.5055822144029,-1.,0.892032620296856));
#29217=CARTESIAN_POINT('Ctrl Pts',(1.5055822144029,1.,0.892032620296856));
#29218=CARTESIAN_POINT('',(1.81978687191668,1.,1.23627494547115));
#29219=CARTESIAN_POINT('Ctrl Pts',(1.81978687191668,1.,1.23627494547115));
#29220=CARTESIAN_POINT('Ctrl Pts',(1.81925017193666,1.,1.23509651170476));
#29221=CARTESIAN_POINT('Ctrl Pts',(1.81817389921279,1.,1.2327422452705));
#29222=CARTESIAN_POINT('Ctrl Pts',(1.8165508718364,1.,1.2292186489137));
#29223=CARTESIAN_POINT('Ctrl Pts',(1.81436959210434,1.,1.2245361330495));
#29224=CARTESIAN_POINT('Ctrl Pts',(1.81161420806656,1.,1.21870906103557));
#29225=CARTESIAN_POINT('Ctrl Pts',(1.80882996917129,1.,1.21290815708314));
#29226=CARTESIAN_POINT('Ctrl Pts',(1.80601678480707,1.,1.20713356605475));
#29227=CARTESIAN_POINT('Ctrl Pts',(1.80317454838603,1.,1.20138548938974));
#29228=CARTESIAN_POINT('Ctrl Pts',(1.80030314369879,1.,1.19566418930242));
#29229=CARTESIAN_POINT('Ctrl Pts',(1.79740245923478,1.,1.18996997934445));
#29230=CARTESIAN_POINT('Ctrl Pts',(1.79447240321515,1.,1.18430321697432));
#29231=CARTESIAN_POINT('Ctrl Pts',(1.79151291552689,1.,1.17866429440809));
#29232=CARTESIAN_POINT('Ctrl Pts',(1.78852398877616,1.,1.17305363177328));
#29233=CARTESIAN_POINT('Ctrl Pts',(1.78550566040443,1.,1.16747166312303));
#29234=CARTESIAN_POINT('Ctrl Pts',(1.78245795881009,1.,1.16191881298499));
#29235=CARTESIAN_POINT('Ctrl Pts',(1.77938085564275,1.,1.15639547194698));
#29236=CARTESIAN_POINT('Ctrl Pts',(1.7762742255701,1.,1.15090197841515));
#29237=CARTESIAN_POINT('Ctrl Pts',(1.77313777896194,1.,1.1454385822692));
#29238=CARTESIAN_POINT('Ctrl Pts',(1.76997111386769,1.,1.14000548336975));
#29239=CARTESIAN_POINT('Ctrl Pts',(1.76677384551862,1.,1.1346029180462));
#29240=CARTESIAN_POINT('Ctrl Pts',(1.7635457196617,1.,1.12923123555075));
#29241=CARTESIAN_POINT('Ctrl Pts',(1.76028671825096,1.,1.12389096855086));
#29242=CARTESIAN_POINT('Ctrl Pts',(1.75699720772105,1.,1.11858293216763));
#29243=CARTESIAN_POINT('Ctrl Pts',(1.7536777209463,1.,1.11330807582551));
#29244=CARTESIAN_POINT('Ctrl Pts',(1.7503286607592,1.,1.10806728183007));
#29245=CARTESIAN_POINT('Ctrl Pts',(1.74695004214923,1.,1.10286118991143));
#29246=CARTESIAN_POINT('Ctrl Pts',(1.74354119236208,1.,1.09768999241226));
#29247=CARTESIAN_POINT('Ctrl Pts',(1.74010053962247,1.,1.09255329056493));
#29248=CARTESIAN_POINT('Ctrl Pts',(1.73662628326091,1.,1.08745056285427));
#29249=CARTESIAN_POINT('Ctrl Pts',(1.73311705663407,1.,1.08238162784749));
#29250=CARTESIAN_POINT('Ctrl Pts',(1.72957248977424,1.,1.0773470373727));
#29251=CARTESIAN_POINT('Ctrl Pts',(1.72599406198488,1.,1.07234866990252));
#29252=CARTESIAN_POINT('Ctrl Pts',(1.72238500928453,1.,1.06738966975462));
#29253=CARTESIAN_POINT('Ctrl Pts',(1.71874858456904,1.,1.06247324680647));
#29254=CARTESIAN_POINT('Ctrl Pts',(1.7150865442702,1.,1.05760163192479));
#29255=CARTESIAN_POINT('Ctrl Pts',(1.71139783543989,1.,1.05277517202855));
#29256=CARTESIAN_POINT('Ctrl Pts',(1.70767646263649,1.,1.04799085404995));
#29257=CARTESIAN_POINT('Ctrl Pts',(1.70391338707982,1.,1.04324363334554));
#29258=CARTESIAN_POINT('Ctrl Pts',(1.70010052930962,1.,1.03852922490789));
#29259=CARTESIAN_POINT('Ctrl Pts',(1.69623414782771,1.,1.03384646003588));
#29260=CARTESIAN_POINT('Ctrl Pts',(1.69231840863458,1.,1.02919977579147));
#29261=CARTESIAN_POINT('Ctrl Pts',(1.68836910178447,1.,1.02460180535255));
#29262=CARTESIAN_POINT('Ctrl Pts',(1.68440578021706,1.,1.02006795074201));
#29263=CARTESIAN_POINT('Ctrl Pts',(1.68044289894798,1.,1.01561026162773));
#29264=CARTESIAN_POINT('Ctrl Pts',(1.67648246776464,1.,1.01123236493511));
#29265=CARTESIAN_POINT('Ctrl Pts',(1.67250335383293,1.,1.00692206696414));
#29266=CARTESIAN_POINT('Ctrl Pts',(1.66846059277303,1.,1.00265091003727));
#29267=CARTESIAN_POINT('Ctrl Pts',(1.66430758030376,1.,0.998389654952758));
#29268=CARTESIAN_POINT('Ctrl Pts',(1.66001553809947,1.,0.994121836661306));
#29269=CARTESIAN_POINT('Ctrl Pts',(1.65559044289699,1.,0.989855627854165));
#29270=CARTESIAN_POINT('Ctrl Pts',(1.65110016612638,1.,0.985642622920821));
#29271=CARTESIAN_POINT('Ctrl Pts',(1.64665139190656,1.,0.981562530939489));
#29272=CARTESIAN_POINT('Ctrl Pts',(1.64233990826687,1.,0.977689794119417));
#29273=CARTESIAN_POINT('Ctrl Pts',(1.63820952658144,1.,0.974066058287419));
#29274=CARTESIAN_POINT('Ctrl Pts',(1.63420665729798,1.,0.970669715997509));
#29275=CARTESIAN_POINT('Ctrl Pts',(1.63013849959461,1.,0.967387853230345));
#29276=CARTESIAN_POINT('Ctrl Pts',(1.62571930670187,1.,0.964046107040536));
#29277=CARTESIAN_POINT('Ctrl Pts',(1.62061638140221,1.,0.960438326101729));
#29278=CARTESIAN_POINT('Ctrl Pts',(1.61449324337085,1.,0.956354422920671));
#29279=CARTESIAN_POINT('Ctrl Pts',(1.60706069896936,1.,0.951613284356035));
#29280=CARTESIAN_POINT('Ctrl Pts',(1.59810042043673,1.,0.946078063315257));
#29281=CARTESIAN_POINT('Ctrl Pts',(1.58744937487176,1.,0.939646377893399));
#29282=CARTESIAN_POINT('Ctrl Pts',(1.57499388382243,1.,0.932246680108685));
#29283=CARTESIAN_POINT('Ctrl Pts',(1.56065988578893,1.,0.923832188944341));
#29284=CARTESIAN_POINT('Ctrl Pts',(1.54440491149498,1.,0.914375919026456));
#29285=CARTESIAN_POINT('Ctrl Pts',(1.52984849887993,1.,0.905967409625651));
#29286=CARTESIAN_POINT('Ctrl Pts',(1.51805569590094,1.,0.899185047483511));
#29287=CARTESIAN_POINT('Ctrl Pts',(1.50980486806688,1.,0.894452006964544));
#29288=CARTESIAN_POINT('Ctrl Pts',(1.5055822144029,1.,0.892032620296856));
#29289=CARTESIAN_POINT('',(1.81978687191668,0.,1.23627494547115));
#29290=CARTESIAN_POINT('Origin',(1.73811241238545,0.,1.34869019493419));
#29291=CARTESIAN_POINT('',(1.73811241238545,1.,1.34869019493419));
#29292=CARTESIAN_POINT('',(1.81978687191668,1.,1.23627494547115));
#29293=CARTESIAN_POINT('',(1.73811241238545,0.,1.34869019493419));
#29294=CARTESIAN_POINT('Ctrl Pts',(1.31362392696032,-1.,1.15624053661742));
#29295=CARTESIAN_POINT('Ctrl Pts',(1.31362392696032,1.,1.15624053661742));
#29296=CARTESIAN_POINT('Ctrl Pts',(1.31722977216397,-1.,1.15950888730809));
#29297=CARTESIAN_POINT('Ctrl Pts',(1.31722977216397,1.,1.15950888730809));
#29298=CARTESIAN_POINT('Ctrl Pts',(1.32428080721772,-1.,1.16589330093588));
#29299=CARTESIAN_POINT('Ctrl Pts',(1.32428080721772,1.,1.16589330093588));
#29300=CARTESIAN_POINT('Ctrl Pts',(1.33437539347008,-1.,1.17501305789857));
#29301=CARTESIAN_POINT('Ctrl Pts',(1.33437539347008,1.,1.17501305789857));
#29302=CARTESIAN_POINT('Ctrl Pts',(1.34687054001093,-1.,1.18625865667441));
#29303=CARTESIAN_POINT('Ctrl Pts',(1.34687054001093,1.,1.18625865667441));
#29304=CARTESIAN_POINT('Ctrl Pts',(1.36088705043885,-1.,1.1987959077932));
#29305=CARTESIAN_POINT('Ctrl Pts',(1.36088705043885,1.,1.1987959077932));
#29306=CARTESIAN_POINT('Ctrl Pts',(1.37331915607905,-1.,1.20982812925645));
#29307=CARTESIAN_POINT('Ctrl Pts',(1.37331915607905,1.,1.20982812925645));
#29308=CARTESIAN_POINT('Ctrl Pts',(1.38420564527715,-1.,1.21938737280852));
#29309=CARTESIAN_POINT('Ctrl Pts',(1.38420564527715,1.,1.21938737280852));
#29310=CARTESIAN_POINT('Ctrl Pts',(1.39361389568796,-1.,1.22752961899387));
#29311=CARTESIAN_POINT('Ctrl Pts',(1.39361389568796,1.,1.22752961899387));
#29312=CARTESIAN_POINT('Ctrl Pts',(1.40164708206106,-1.,1.23434087290423));
#29313=CARTESIAN_POINT('Ctrl Pts',(1.40164708206106,1.,1.23434087290423));
#29314=CARTESIAN_POINT('Ctrl Pts',(1.40845295531283,-1.,1.23994455029534));
#29315=CARTESIAN_POINT('Ctrl Pts',(1.40845295531283,1.,1.23994455029534));
#29316=CARTESIAN_POINT('Ctrl Pts',(1.41422913175179,-1.,1.24450600513056));
#29317=CARTESIAN_POINT('Ctrl Pts',(1.41422913175179,1.,1.24450600513056));
#29318=CARTESIAN_POINT('Ctrl Pts',(1.41923722596025,-1.,1.24824430986571));
#29319=CARTESIAN_POINT('Ctrl Pts',(1.41923722596025,1.,1.24824430986571));
#29320=CARTESIAN_POINT('Ctrl Pts',(1.42378102115575,-1.,1.2514145557001));
#29321=CARTESIAN_POINT('Ctrl Pts',(1.42378102115575,1.,1.2514145557001));
#29322=CARTESIAN_POINT('Ctrl Pts',(1.42815938799387,-1.,1.25426945222639));
#29323=CARTESIAN_POINT('Ctrl Pts',(1.42815938799387,1.,1.25426945222639));
#29324=CARTESIAN_POINT('Ctrl Pts',(1.43262645609691,-1.,1.25702687965755));
#29325=CARTESIAN_POINT('Ctrl Pts',(1.43262645609691,1.,1.25702687965755));
#29326=CARTESIAN_POINT('Ctrl Pts',(1.43734919180847,-1.,1.25983531012005));
#29327=CARTESIAN_POINT('Ctrl Pts',(1.43734919180847,1.,1.25983531012005));
#29328=CARTESIAN_POINT('Ctrl Pts',(1.44236470511303,-1.,1.26273903323859));
#29329=CARTESIAN_POINT('Ctrl Pts',(1.44236470511303,1.,1.26273903323859));
#29330=CARTESIAN_POINT('Ctrl Pts',(1.44761985001662,-1.,1.26570925118868));
#29331=CARTESIAN_POINT('Ctrl Pts',(1.44761985001662,1.,1.26570925118868));
#29332=CARTESIAN_POINT('Ctrl Pts',(1.45301422764247,-1.,1.2686778680489));
#29333=CARTESIAN_POINT('Ctrl Pts',(1.45301422764247,1.,1.2686778680489));
#29334=CARTESIAN_POINT('Ctrl Pts',(1.45843906294697,-1.,1.27156805265289));
#29335=CARTESIAN_POINT('Ctrl Pts',(1.45843906294697,1.,1.27156805265289));
#29336=CARTESIAN_POINT('Ctrl Pts',(1.46382431332476,-1.,1.27433119897822));
#29337=CARTESIAN_POINT('Ctrl Pts',(1.46382431332476,1.,1.27433119897822));
#29338=CARTESIAN_POINT('Ctrl Pts',(1.46916035917133,-1.,1.2769641483109));
#29339=CARTESIAN_POINT('Ctrl Pts',(1.46916035917133,1.,1.2769641483109));
#29340=CARTESIAN_POINT('Ctrl Pts',(1.4744717526707,-1.,1.2794891824849));
#29341=CARTESIAN_POINT('Ctrl Pts',(1.4744717526707,1.,1.2794891824849));
#29342=CARTESIAN_POINT('Ctrl Pts',(1.47980070347095,-1.,1.28194158939517));
#29343=CARTESIAN_POINT('Ctrl Pts',(1.47980070347095,1.,1.28194158939517));
#29344=CARTESIAN_POINT('Ctrl Pts',(1.4851881711891,-1.,1.28435533880201));
#29345=CARTESIAN_POINT('Ctrl Pts',(1.4851881711891,1.,1.28435533880201));
#29346=CARTESIAN_POINT('Ctrl Pts',(1.4906522831278,-1.,1.2867467611644));
#29347=CARTESIAN_POINT('Ctrl Pts',(1.4906522831278,1.,1.2867467611644));
#29348=CARTESIAN_POINT('Ctrl Pts',(1.49618896881754,-1.,1.28911506584254));
#29349=CARTESIAN_POINT('Ctrl Pts',(1.49618896881754,1.,1.28911506584254));
#29350=CARTESIAN_POINT('Ctrl Pts',(1.50178230149776,-1.,1.29145022885181));
#29351=CARTESIAN_POINT('Ctrl Pts',(1.50178230149776,1.,1.29145022885181));
#29352=CARTESIAN_POINT('Ctrl Pts',(1.50741159078365,-1.,1.29373841372842));
#29353=CARTESIAN_POINT('Ctrl Pts',(1.50741159078365,1.,1.29373841372842));
#29354=CARTESIAN_POINT('Ctrl Pts',(1.51305994241402,-1.,1.29596850710509));
#29355=CARTESIAN_POINT('Ctrl Pts',(1.51305994241402,1.,1.29596850710509));
#29356=CARTESIAN_POINT('Ctrl Pts',(1.51872184912724,-1.,1.29813791800747));
#29357=CARTESIAN_POINT('Ctrl Pts',(1.51872184912724,1.,1.29813791800747));
#29358=CARTESIAN_POINT('Ctrl Pts',(1.52439957861062,-1.,1.30024984366328));
#29359=CARTESIAN_POINT('Ctrl Pts',(1.52439957861062,1.,1.30024984366328));
#29360=CARTESIAN_POINT('Ctrl Pts',(1.53009970283891,-1.,1.30231064395568));
#29361=CARTESIAN_POINT('Ctrl Pts',(1.53009970283891,1.,1.30231064395568));
#29362=CARTESIAN_POINT('Ctrl Pts',(1.53582981268977,-1.,1.30432735639489));
#29363=CARTESIAN_POINT('Ctrl Pts',(1.53582981268977,1.,1.30432735639489));
#29364=CARTESIAN_POINT('Ctrl Pts',(1.54159462645432,-1.,1.30630475189556));
#29365=CARTESIAN_POINT('Ctrl Pts',(1.54159462645432,1.,1.30630475189556));
#29366=CARTESIAN_POINT('Ctrl Pts',(1.54739413957185,-1.,1.30824393907473));
#29367=CARTESIAN_POINT('Ctrl Pts',(1.54739413957185,1.,1.30824393907473));
#29368=CARTESIAN_POINT('Ctrl Pts',(1.55322568759481,-1.,1.31014393684222));
#29369=CARTESIAN_POINT('Ctrl Pts',(1.55322568759481,1.,1.31014393684222));
#29370=CARTESIAN_POINT('Ctrl Pts',(1.55908521254821,-1.,1.31200264341696));
#29371=CARTESIAN_POINT('Ctrl Pts',(1.55908521254821,1.,1.31200264341696));
#29372=CARTESIAN_POINT('Ctrl Pts',(1.56496872402353,-1.,1.31381795281002));
#29373=CARTESIAN_POINT('Ctrl Pts',(1.56496872402353,1.,1.31381795281002));
#29374=CARTESIAN_POINT('Ctrl Pts',(1.57087397835723,-1.,1.31558903860016));
#29375=CARTESIAN_POINT('Ctrl Pts',(1.57087397835723,1.,1.31558903860016));
#29376=CARTESIAN_POINT('Ctrl Pts',(1.5768005650559,-1.,1.31731642317187));
#29377=CARTESIAN_POINT('Ctrl Pts',(1.5768005650559,1.,1.31731642317187));
#29378=CARTESIAN_POINT('Ctrl Pts',(1.58274907898834,-1.,1.31900135021432));
#29379=CARTESIAN_POINT('Ctrl Pts',(1.58274907898834,1.,1.31900135021432));
#29380=CARTESIAN_POINT('Ctrl Pts',(1.58872057258245,-1.,1.32064537110892));
#29381=CARTESIAN_POINT('Ctrl Pts',(1.58872057258245,1.,1.32064537110892));
#29382=CARTESIAN_POINT('Ctrl Pts',(1.59471591079403,-1.,1.32224985747682));
#29383=CARTESIAN_POINT('Ctrl Pts',(1.59471591079403,1.,1.32224985747682));
#29384=CARTESIAN_POINT('Ctrl Pts',(1.60073511858687,-1.,1.32381550858256));
#29385=CARTESIAN_POINT('Ctrl Pts',(1.60073511858687,1.,1.32381550858256));
#29386=CARTESIAN_POINT('Ctrl Pts',(1.60677758290954,-1.,1.32534250785782));
#29387=CARTESIAN_POINT('Ctrl Pts',(1.60677758290954,1.,1.32534250785782));
#29388=CARTESIAN_POINT('Ctrl Pts',(1.6128423401575,-1.,1.32683074483356));
#29389=CARTESIAN_POINT('Ctrl Pts',(1.6128423401575,1.,1.32683074483356));
#29390=CARTESIAN_POINT('Ctrl Pts',(1.61892832270724,-1.,1.32828000610449));
#29391=CARTESIAN_POINT('Ctrl Pts',(1.61892832270724,1.,1.32828000610449));
#29392=CARTESIAN_POINT('Ctrl Pts',(1.62503464209797,-1.,1.3296901950568));
#29393=CARTESIAN_POINT('Ctrl Pts',(1.62503464209797,1.,1.3296901950568));
#29394=CARTESIAN_POINT('Ctrl Pts',(1.63116079730923,-1.,1.33106149345645));
#29395=CARTESIAN_POINT('Ctrl Pts',(1.63116079730923,1.,1.33106149345645));
#29396=CARTESIAN_POINT('Ctrl Pts',(1.63730653475089,-1.,1.33239425103724));
#29397=CARTESIAN_POINT('Ctrl Pts',(1.63730653475089,1.,1.33239425103724));
#29398=CARTESIAN_POINT('Ctrl Pts',(1.6434717485603,-1.,1.33368890676572));
#29399=CARTESIAN_POINT('Ctrl Pts',(1.6434717485603,1.,1.33368890676572));
#29400=CARTESIAN_POINT('Ctrl Pts',(1.6496563728683,-1.,1.33494590467993));
#29401=CARTESIAN_POINT('Ctrl Pts',(1.6496563728683,1.,1.33494590467993));
#29402=CARTESIAN_POINT('Ctrl Pts',(1.65586025952593,-1.,1.33616559745172));
#29403=CARTESIAN_POINT('Ctrl Pts',(1.65586025952593,1.,1.33616559745172));
#29404=CARTESIAN_POINT('Ctrl Pts',(1.66208312541983,-1.,1.33734820885262));
#29405=CARTESIAN_POINT('Ctrl Pts',(1.66208312541983,1.,1.33734820885262));
#29406=CARTESIAN_POINT('Ctrl Pts',(1.66832460783989,-1.,1.33849388654388));
#29407=CARTESIAN_POINT('Ctrl Pts',(1.66832460783989,1.,1.33849388654388));
#29408=CARTESIAN_POINT('Ctrl Pts',(1.67458429426086,-1.,1.3396027347034));
#29409=CARTESIAN_POINT('Ctrl Pts',(1.67458429426086,1.,1.3396027347034));
#29410=CARTESIAN_POINT('Ctrl Pts',(1.68086176030362,-1.,1.34067485185203));
#29411=CARTESIAN_POINT('Ctrl Pts',(1.68086176030362,1.,1.34067485185203));
#29412=CARTESIAN_POINT('Ctrl Pts',(1.68715660868764,-1.,1.341710374848));
#29413=CARTESIAN_POINT('Ctrl Pts',(1.68715660868764,1.,1.341710374848));
#29414=CARTESIAN_POINT('Ctrl Pts',(1.6934684849687,-1.,1.34270948206319));
#29415=CARTESIAN_POINT('Ctrl Pts',(1.6934684849687,1.,1.34270948206319));
#29416=CARTESIAN_POINT('Ctrl Pts',(1.69979707754427,-1.,1.34367237124483));
#29417=CARTESIAN_POINT('Ctrl Pts',(1.69979707754427,1.,1.34367237124483));
#29418=CARTESIAN_POINT('Ctrl Pts',(1.70614212266738,-1.,1.34459924533831));
#29419=CARTESIAN_POINT('Ctrl Pts',(1.70614212266738,1.,1.34459924533831));
#29420=CARTESIAN_POINT('Ctrl Pts',(1.71250340686822,-1.,1.34549029589416));
#29421=CARTESIAN_POINT('Ctrl Pts',(1.71250340686822,1.,1.34549029589416));
#29422=CARTESIAN_POINT('Ctrl Pts',(1.7188807715049,-1.,1.34634568653227));
#29423=CARTESIAN_POINT('Ctrl Pts',(1.7188807715049,1.,1.34634568653227));
#29424=CARTESIAN_POINT('Ctrl Pts',(1.72527410680674,-1.,1.34716554819527));
#29425=CARTESIAN_POINT('Ctrl Pts',(1.72527410680674,1.,1.34716554819527));
#29426=CARTESIAN_POINT('Ctrl Pts',(1.7304014965394,-1.,1.34779309152035));
#29427=CARTESIAN_POINT('Ctrl Pts',(1.7304014965394,1.,1.34779309152035));
#29428=CARTESIAN_POINT('Ctrl Pts',(1.73425417885907,-1.,1.34824783112887));
#29429=CARTESIAN_POINT('Ctrl Pts',(1.73425417885907,1.,1.34824783112887));
#29430=CARTESIAN_POINT('Ctrl Pts',(1.73682580585691,-1.,1.34854391898045));
#29431=CARTESIAN_POINT('Ctrl Pts',(1.73682580585691,1.,1.34854391898045));
#29432=CARTESIAN_POINT('Ctrl Pts',(1.73811241238545,-1.,1.34869019493419));
#29433=CARTESIAN_POINT('Ctrl Pts',(1.73811241238545,1.,1.34869019493419));
#29434=CARTESIAN_POINT('',(1.31362392696032,1.,1.15624053661742));
#29435=CARTESIAN_POINT('Ctrl Pts',(1.31362392696032,1.,1.15624053661742));
#29436=CARTESIAN_POINT('Ctrl Pts',(1.31722977216397,1.,1.15950888730809));
#29437=CARTESIAN_POINT('Ctrl Pts',(1.32428080721772,1.,1.16589330093588));
#29438=CARTESIAN_POINT('Ctrl Pts',(1.33437539347008,1.,1.17501305789857));
#29439=CARTESIAN_POINT('Ctrl Pts',(1.34687054001093,1.,1.18625865667441));
#29440=CARTESIAN_POINT('Ctrl Pts',(1.36088705043885,1.,1.1987959077932));
#29441=CARTESIAN_POINT('Ctrl Pts',(1.37331915607905,1.,1.20982812925645));
#29442=CARTESIAN_POINT('Ctrl Pts',(1.38420564527715,1.,1.21938737280852));
#29443=CARTESIAN_POINT('Ctrl Pts',(1.39361389568796,1.,1.22752961899387));
#29444=CARTESIAN_POINT('Ctrl Pts',(1.40164708206106,1.,1.23434087290423));
#29445=CARTESIAN_POINT('Ctrl Pts',(1.40845295531283,1.,1.23994455029534));
#29446=CARTESIAN_POINT('Ctrl Pts',(1.41422913175179,1.,1.24450600513056));
#29447=CARTESIAN_POINT('Ctrl Pts',(1.41923722596025,1.,1.24824430986571));
#29448=CARTESIAN_POINT('Ctrl Pts',(1.42378102115575,1.,1.2514145557001));
#29449=CARTESIAN_POINT('Ctrl Pts',(1.42815938799387,1.,1.25426945222639));
#29450=CARTESIAN_POINT('Ctrl Pts',(1.43262645609691,1.,1.25702687965755));
#29451=CARTESIAN_POINT('Ctrl Pts',(1.43734919180847,1.,1.25983531012005));
#29452=CARTESIAN_POINT('Ctrl Pts',(1.44236470511303,1.,1.26273903323859));
#29453=CARTESIAN_POINT('Ctrl Pts',(1.44761985001662,1.,1.26570925118868));
#29454=CARTESIAN_POINT('Ctrl Pts',(1.45301422764247,1.,1.2686778680489));
#29455=CARTESIAN_POINT('Ctrl Pts',(1.45843906294697,1.,1.27156805265289));
#29456=CARTESIAN_POINT('Ctrl Pts',(1.46382431332476,1.,1.27433119897822));
#29457=CARTESIAN_POINT('Ctrl Pts',(1.46916035917133,1.,1.2769641483109));
#29458=CARTESIAN_POINT('Ctrl Pts',(1.4744717526707,1.,1.2794891824849));
#29459=CARTESIAN_POINT('Ctrl Pts',(1.47980070347095,1.,1.28194158939517));
#29460=CARTESIAN_POINT('Ctrl Pts',(1.4851881711891,1.,1.28435533880201));
#29461=CARTESIAN_POINT('Ctrl Pts',(1.4906522831278,1.,1.2867467611644));
#29462=CARTESIAN_POINT('Ctrl Pts',(1.49618896881754,1.,1.28911506584254));
#29463=CARTESIAN_POINT('Ctrl Pts',(1.50178230149776,1.,1.29145022885181));
#29464=CARTESIAN_POINT('Ctrl Pts',(1.50741159078365,1.,1.29373841372842));
#29465=CARTESIAN_POINT('Ctrl Pts',(1.51305994241402,1.,1.29596850710509));
#29466=CARTESIAN_POINT('Ctrl Pts',(1.51872184912724,1.,1.29813791800747));
#29467=CARTESIAN_POINT('Ctrl Pts',(1.52439957861062,1.,1.30024984366328));
#29468=CARTESIAN_POINT('Ctrl Pts',(1.53009970283891,1.,1.30231064395568));
#29469=CARTESIAN_POINT('Ctrl Pts',(1.53582981268977,1.,1.30432735639489));
#29470=CARTESIAN_POINT('Ctrl Pts',(1.54159462645432,1.,1.30630475189556));
#29471=CARTESIAN_POINT('Ctrl Pts',(1.54739413957185,1.,1.30824393907473));
#29472=CARTESIAN_POINT('Ctrl Pts',(1.55322568759481,1.,1.31014393684222));
#29473=CARTESIAN_POINT('Ctrl Pts',(1.55908521254821,1.,1.31200264341696));
#29474=CARTESIAN_POINT('Ctrl Pts',(1.56496872402353,1.,1.31381795281002));
#29475=CARTESIAN_POINT('Ctrl Pts',(1.57087397835723,1.,1.31558903860016));
#29476=CARTESIAN_POINT('Ctrl Pts',(1.5768005650559,1.,1.31731642317187));
#29477=CARTESIAN_POINT('Ctrl Pts',(1.58274907898834,1.,1.31900135021432));
#29478=CARTESIAN_POINT('Ctrl Pts',(1.58872057258245,1.,1.32064537110892));
#29479=CARTESIAN_POINT('Ctrl Pts',(1.59471591079403,1.,1.32224985747682));
#29480=CARTESIAN_POINT('Ctrl Pts',(1.60073511858687,1.,1.32381550858256));
#29481=CARTESIAN_POINT('Ctrl Pts',(1.60677758290954,1.,1.32534250785782));
#29482=CARTESIAN_POINT('Ctrl Pts',(1.6128423401575,1.,1.32683074483356));
#29483=CARTESIAN_POINT('Ctrl Pts',(1.61892832270724,1.,1.32828000610449));
#29484=CARTESIAN_POINT('Ctrl Pts',(1.62503464209797,1.,1.3296901950568));
#29485=CARTESIAN_POINT('Ctrl Pts',(1.63116079730923,1.,1.33106149345645));
#29486=CARTESIAN_POINT('Ctrl Pts',(1.63730653475089,1.,1.33239425103724));
#29487=CARTESIAN_POINT('Ctrl Pts',(1.6434717485603,1.,1.33368890676572));
#29488=CARTESIAN_POINT('Ctrl Pts',(1.6496563728683,1.,1.33494590467993));
#29489=CARTESIAN_POINT('Ctrl Pts',(1.65586025952593,1.,1.33616559745172));
#29490=CARTESIAN_POINT('Ctrl Pts',(1.66208312541983,1.,1.33734820885262));
#29491=CARTESIAN_POINT('Ctrl Pts',(1.66832460783989,1.,1.33849388654388));
#29492=CARTESIAN_POINT('Ctrl Pts',(1.67458429426086,1.,1.3396027347034));
#29493=CARTESIAN_POINT('Ctrl Pts',(1.68086176030362,1.,1.34067485185203));
#29494=CARTESIAN_POINT('Ctrl Pts',(1.68715660868764,1.,1.341710374848));
#29495=CARTESIAN_POINT('Ctrl Pts',(1.6934684849687,1.,1.34270948206319));
#29496=CARTESIAN_POINT('Ctrl Pts',(1.69979707754427,1.,1.34367237124483));
#29497=CARTESIAN_POINT('Ctrl Pts',(1.70614212266738,1.,1.34459924533831));
#29498=CARTESIAN_POINT('Ctrl Pts',(1.71250340686822,1.,1.34549029589416));
#29499=CARTESIAN_POINT('Ctrl Pts',(1.7188807715049,1.,1.34634568653227));
#29500=CARTESIAN_POINT('Ctrl Pts',(1.72527410680674,1.,1.34716554819527));
#29501=CARTESIAN_POINT('Ctrl Pts',(1.7304014965394,1.,1.34779309152035));
#29502=CARTESIAN_POINT('Ctrl Pts',(1.73425417885907,1.,1.34824783112887));
#29503=CARTESIAN_POINT('Ctrl Pts',(1.73682580585691,1.,1.34854391898045));
#29504=CARTESIAN_POINT('Ctrl Pts',(1.73811241238545,1.,1.34869019493419));
#29505=CARTESIAN_POINT('',(1.31362392696032,0.,1.15624053661742));
#29506=CARTESIAN_POINT('Origin',(0.,0.,0.));
#29507=CARTESIAN_POINT('',(1.15624053661742,1.,1.31362392696033));
#29508=CARTESIAN_POINT('Origin',(0.,1.,0.));
#29509=CARTESIAN_POINT('',(1.15624053661742,0.,1.31362392696032));
#29510=CARTESIAN_POINT('Ctrl Pts',(1.34869019493419,-1.,1.73811241238545));
#29511=CARTESIAN_POINT('Ctrl Pts',(1.34869019493419,1.,1.73811241238545));
#29512=CARTESIAN_POINT('Ctrl Pts',(1.34854391898145,-1.,1.73682580585819));
#29513=CARTESIAN_POINT('Ctrl Pts',(1.34854391898145,1.,1.73682580585819));
#29514=CARTESIAN_POINT('Ctrl Pts',(1.34824783113158,-1.,1.73425417886255));
#29515=CARTESIAN_POINT('Ctrl Pts',(1.34824783113158,1.,1.73425417886255));
#29516=CARTESIAN_POINT('Ctrl Pts',(1.3477930915247,-1.,1.73040149654497));
#29517=CARTESIAN_POINT('Ctrl Pts',(1.3477930915247,1.,1.73040149654497));
#29518=CARTESIAN_POINT('Ctrl Pts',(1.34716554820013,-1.,1.72527410681298));
#29519=CARTESIAN_POINT('Ctrl Pts',(1.34716554820013,1.,1.72527410681298));
#29520=CARTESIAN_POINT('Ctrl Pts',(1.34634568653586,-1.,1.7188807715095));
#29521=CARTESIAN_POINT('Ctrl Pts',(1.34634568653586,1.,1.7188807715095));
#29522=CARTESIAN_POINT('Ctrl Pts',(1.34549029589563,-1.,1.71250340687011));
#29523=CARTESIAN_POINT('Ctrl Pts',(1.34549029589563,1.,1.71250340687011));
#29524=CARTESIAN_POINT('Ctrl Pts',(1.34459924533783,-1.,1.70614212266676));
#29525=CARTESIAN_POINT('Ctrl Pts',(1.34459924533783,1.,1.70614212266676));
#29526=CARTESIAN_POINT('Ctrl Pts',(1.34367237124322,-1.,1.69979707754221));
#29527=CARTESIAN_POINT('Ctrl Pts',(1.34367237124322,1.,1.69979707754221));
#29528=CARTESIAN_POINT('Ctrl Pts',(1.34270948206139,-1.,1.6934684849664));
#29529=CARTESIAN_POINT('Ctrl Pts',(1.34270948206139,1.,1.6934684849664));
#29530=CARTESIAN_POINT('Ctrl Pts',(1.34171037484673,-1.,1.68715660868602));
#29531=CARTESIAN_POINT('Ctrl Pts',(1.34171037484673,1.,1.68715660868602));
#29532=CARTESIAN_POINT('Ctrl Pts',(1.3406748518516,-1.,1.68086176030308));
#29533=CARTESIAN_POINT('Ctrl Pts',(1.3406748518516,1.,1.68086176030308));
#29534=CARTESIAN_POINT('Ctrl Pts',(1.33960273470372,-1.,1.67458429426126));
#29535=CARTESIAN_POINT('Ctrl Pts',(1.33960273470372,1.,1.67458429426126));
#29536=CARTESIAN_POINT('Ctrl Pts',(1.33849388654458,-1.,1.66832460784078));
#29537=CARTESIAN_POINT('Ctrl Pts',(1.33849388654458,1.,1.66832460784078));
#29538=CARTESIAN_POINT('Ctrl Pts',(1.33734820885331,-1.,1.66208312542073));
#29539=CARTESIAN_POINT('Ctrl Pts',(1.33734820885331,1.,1.66208312542073));
#29540=CARTESIAN_POINT('Ctrl Pts',(1.33616559745217,-1.,1.65586025952651));
#29541=CARTESIAN_POINT('Ctrl Pts',(1.33616559745217,1.,1.65586025952651));
#29542=CARTESIAN_POINT('Ctrl Pts',(1.33494590468003,-1.,1.64965637286843));
#29543=CARTESIAN_POINT('Ctrl Pts',(1.33494590468003,1.,1.64965637286843));
#29544=CARTESIAN_POINT('Ctrl Pts',(1.33368890676554,-1.,1.64347174856007));
#29545=CARTESIAN_POINT('Ctrl Pts',(1.33368890676554,1.,1.64347174856007));
#29546=CARTESIAN_POINT('Ctrl Pts',(1.33239425103694,-1.,1.6373065347505));
#29547=CARTESIAN_POINT('Ctrl Pts',(1.33239425103694,1.,1.6373065347505));
#29548=CARTESIAN_POINT('Ctrl Pts',(1.33106149345618,-1.,1.63116079730887));
#29549=CARTESIAN_POINT('Ctrl Pts',(1.33106149345618,1.,1.63116079730887));
#29550=CARTESIAN_POINT('Ctrl Pts',(1.32969019505665,-1.,1.62503464209777));
#29551=CARTESIAN_POINT('Ctrl Pts',(1.32969019505665,1.,1.62503464209777));
#29552=CARTESIAN_POINT('Ctrl Pts',(1.32828000610448,-1.,1.61892832270723));
#29553=CARTESIAN_POINT('Ctrl Pts',(1.32828000610448,1.,1.61892832270723));
#29554=CARTESIAN_POINT('Ctrl Pts',(1.32683074483365,-1.,1.61284234015762));
#29555=CARTESIAN_POINT('Ctrl Pts',(1.32683074483365,1.,1.61284234015762));
#29556=CARTESIAN_POINT('Ctrl Pts',(1.32534250785794,-1.,1.6067775829097));
#29557=CARTESIAN_POINT('Ctrl Pts',(1.32534250785794,1.,1.6067775829097));
#29558=CARTESIAN_POINT('Ctrl Pts',(1.32381550858266,-1.,1.600735118587));
#29559=CARTESIAN_POINT('Ctrl Pts',(1.32381550858266,1.,1.600735118587));
#29560=CARTESIAN_POINT('Ctrl Pts',(1.32224985747686,-1.,1.59471591079408));
#29561=CARTESIAN_POINT('Ctrl Pts',(1.32224985747686,1.,1.59471591079408));
#29562=CARTESIAN_POINT('Ctrl Pts',(1.32064537110891,-1.,1.58872057258244));
#29563=CARTESIAN_POINT('Ctrl Pts',(1.32064537110891,1.,1.58872057258244));
#29564=CARTESIAN_POINT('Ctrl Pts',(1.31900135021428,-1.,1.58274907898829));
#29565=CARTESIAN_POINT('Ctrl Pts',(1.31900135021428,1.,1.58274907898829));
#29566=CARTESIAN_POINT('Ctrl Pts',(1.31731642317183,-1.,1.57680056505585));
#29567=CARTESIAN_POINT('Ctrl Pts',(1.31731642317183,1.,1.57680056505585));
#29568=CARTESIAN_POINT('Ctrl Pts',(1.31558903860015,-1.,1.57087397835721));
#29569=CARTESIAN_POINT('Ctrl Pts',(1.31558903860015,1.,1.57087397835721));
#29570=CARTESIAN_POINT('Ctrl Pts',(1.31381795281002,-1.,1.56496872402352));
#29571=CARTESIAN_POINT('Ctrl Pts',(1.31381795281002,1.,1.56496872402352));
#29572=CARTESIAN_POINT('Ctrl Pts',(1.31200264341696,-1.,1.55908521254822));
#29573=CARTESIAN_POINT('Ctrl Pts',(1.31200264341696,1.,1.55908521254822));
#29574=CARTESIAN_POINT('Ctrl Pts',(1.31014393684221,-1.,1.55322568759481));
#29575=CARTESIAN_POINT('Ctrl Pts',(1.31014393684221,1.,1.55322568759481));
#29576=CARTESIAN_POINT('Ctrl Pts',(1.30824393907471,-1.,1.54739413957183));
#29577=CARTESIAN_POINT('Ctrl Pts',(1.30824393907471,1.,1.54739413957183));
#29578=CARTESIAN_POINT('Ctrl Pts',(1.30630475189553,-1.,1.54159462645428));
#29579=CARTESIAN_POINT('Ctrl Pts',(1.30630475189553,1.,1.54159462645428));
#29580=CARTESIAN_POINT('Ctrl Pts',(1.30432735639487,-1.,1.53582981268976));
#29581=CARTESIAN_POINT('Ctrl Pts',(1.30432735639487,1.,1.53582981268976));
#29582=CARTESIAN_POINT('Ctrl Pts',(1.3023106439557,-1.,1.53009970283893));
#29583=CARTESIAN_POINT('Ctrl Pts',(1.3023106439557,1.,1.53009970283893));
#29584=CARTESIAN_POINT('Ctrl Pts',(1.30024984366334,-1.,1.5243995786107));
#29585=CARTESIAN_POINT('Ctrl Pts',(1.30024984366334,1.,1.5243995786107));
#29586=CARTESIAN_POINT('Ctrl Pts',(1.29813791800757,-1.,1.51872184912735));
#29587=CARTESIAN_POINT('Ctrl Pts',(1.29813791800757,1.,1.51872184912735));
#29588=CARTESIAN_POINT('Ctrl Pts',(1.29596850710518,-1.,1.51305994241412));
#29589=CARTESIAN_POINT('Ctrl Pts',(1.29596850710518,1.,1.51305994241412));
#29590=CARTESIAN_POINT('Ctrl Pts',(1.29373841372843,-1.,1.50741159078367));
#29591=CARTESIAN_POINT('Ctrl Pts',(1.29373841372843,1.,1.50741159078367));
#29592=CARTESIAN_POINT('Ctrl Pts',(1.29145022885171,-1.,1.50178230149764));
#29593=CARTESIAN_POINT('Ctrl Pts',(1.29145022885171,1.,1.50178230149764));
#29594=CARTESIAN_POINT('Ctrl Pts',(1.28911506584232,-1.,1.49618896881729));
#29595=CARTESIAN_POINT('Ctrl Pts',(1.28911506584232,1.,1.49618896881729));
#29596=CARTESIAN_POINT('Ctrl Pts',(1.28674676116415,-1.,1.4906522831275));
#29597=CARTESIAN_POINT('Ctrl Pts',(1.28674676116415,1.,1.4906522831275));
#29598=CARTESIAN_POINT('Ctrl Pts',(1.28435533880184,-1.,1.48518817118891));
#29599=CARTESIAN_POINT('Ctrl Pts',(1.28435533880184,1.,1.48518817118891));
#29600=CARTESIAN_POINT('Ctrl Pts',(1.28194158939522,-1.,1.47980070347102));
#29601=CARTESIAN_POINT('Ctrl Pts',(1.28194158939522,1.,1.47980070347102));
#29602=CARTESIAN_POINT('Ctrl Pts',(1.27948918248524,-1.,1.4744717526711));
#29603=CARTESIAN_POINT('Ctrl Pts',(1.27948918248524,1.,1.4744717526711));
#29604=CARTESIAN_POINT('Ctrl Pts',(1.27696414831144,-1.,1.46916035917197));
#29605=CARTESIAN_POINT('Ctrl Pts',(1.27696414831144,1.,1.46916035917197));
#29606=CARTESIAN_POINT('Ctrl Pts',(1.27433119897877,-1.,1.4638243133254));
#29607=CARTESIAN_POINT('Ctrl Pts',(1.27433119897877,1.,1.4638243133254));
#29608=CARTESIAN_POINT('Ctrl Pts',(1.27156805265312,-1.,1.45843906294725));
#29609=CARTESIAN_POINT('Ctrl Pts',(1.27156805265312,1.,1.45843906294725));
#29610=CARTESIAN_POINT('Ctrl Pts',(1.26867786804854,-1.,1.45301422764205));
#29611=CARTESIAN_POINT('Ctrl Pts',(1.26867786804854,1.,1.45301422764205));
#29612=CARTESIAN_POINT('Ctrl Pts',(1.26570925118767,-1.,1.44761985001544));
#29613=CARTESIAN_POINT('Ctrl Pts',(1.26570925118767,1.,1.44761985001544));
#29614=CARTESIAN_POINT('Ctrl Pts',(1.26273903323723,-1.,1.44236470511145));
#29615=CARTESIAN_POINT('Ctrl Pts',(1.26273903323723,1.,1.44236470511145));
#29616=CARTESIAN_POINT('Ctrl Pts',(1.25983531011894,-1.,1.43734919180719));
#29617=CARTESIAN_POINT('Ctrl Pts',(1.25983531011894,1.,1.43734919180719));
#29618=CARTESIAN_POINT('Ctrl Pts',(1.25702687965744,-1.,1.43262645609679));
#29619=CARTESIAN_POINT('Ctrl Pts',(1.25702687965744,1.,1.43262645609679));
#29620=CARTESIAN_POINT('Ctrl Pts',(1.25426945222783,-1.,1.42815938799555));
#29621=CARTESIAN_POINT('Ctrl Pts',(1.25426945222783,1.,1.42815938799555));
#29622=CARTESIAN_POINT('Ctrl Pts',(1.25141455570299,-1.,1.42378102115911));
#29623=CARTESIAN_POINT('Ctrl Pts',(1.25141455570299,1.,1.42378102115911));
#29624=CARTESIAN_POINT('Ctrl Pts',(1.24824430986911,-1.,1.41923722596421));
#29625=CARTESIAN_POINT('Ctrl Pts',(1.24824430986911,1.,1.41923722596421));
#29626=CARTESIAN_POINT('Ctrl Pts',(1.24450600513278,-1.,1.41422913175437));
#29627=CARTESIAN_POINT('Ctrl Pts',(1.24450600513278,1.,1.41422913175437));
#29628=CARTESIAN_POINT('Ctrl Pts',(1.23994455029421,-1.,1.40845295531151));
#29629=CARTESIAN_POINT('Ctrl Pts',(1.23994455029421,1.,1.40845295531151));
#29630=CARTESIAN_POINT('Ctrl Pts',(1.23434087289768,-1.,1.40164708205345));
#29631=CARTESIAN_POINT('Ctrl Pts',(1.23434087289768,1.,1.40164708205345));
#29632=CARTESIAN_POINT('Ctrl Pts',(1.22752961898063,-1.,1.39361389567257));
#29633=CARTESIAN_POINT('Ctrl Pts',(1.22752961898063,1.,1.39361389567257));
#29634=CARTESIAN_POINT('Ctrl Pts',(1.21938737278853,-1.,1.38420564525391));
#29635=CARTESIAN_POINT('Ctrl Pts',(1.21938737278853,1.,1.38420564525391));
#29636=CARTESIAN_POINT('Ctrl Pts',(1.20982812923113,-1.,1.37331915604962));
#29637=CARTESIAN_POINT('Ctrl Pts',(1.20982812923113,1.,1.37331915604962));
#29638=CARTESIAN_POINT('Ctrl Pts',(1.1987959077656,-1.,1.36088705040677));
#29639=CARTESIAN_POINT('Ctrl Pts',(1.1987959077656,1.,1.36088705040677));
#29640=CARTESIAN_POINT('Ctrl Pts',(1.18625865664915,-1.,1.34687053998157));
#29641=CARTESIAN_POINT('Ctrl Pts',(1.18625865664915,1.,1.34687053998157));
#29642=CARTESIAN_POINT('Ctrl Pts',(1.17501305787994,-1.,1.33437539344842));
#29643=CARTESIAN_POINT('Ctrl Pts',(1.17501305787994,1.,1.33437539344842));
#29644=CARTESIAN_POINT('Ctrl Pts',(1.16589330092532,-1.,1.32428080720544));
#29645=CARTESIAN_POINT('Ctrl Pts',(1.16589330092532,1.,1.32428080720544));
#29646=CARTESIAN_POINT('Ctrl Pts',(1.15950888730433,-1.,1.3172297721596));
#29647=CARTESIAN_POINT('Ctrl Pts',(1.15950888730433,1.,1.3172297721596));
#29648=CARTESIAN_POINT('Ctrl Pts',(1.15624053661742,-1.,1.31362392696033));
#29649=CARTESIAN_POINT('Ctrl Pts',(1.15624053661742,1.,1.31362392696033));
#29650=CARTESIAN_POINT('',(1.34869019493419,1.,1.73811241238545));
#29651=CARTESIAN_POINT('Ctrl Pts',(1.34869019493419,1.,1.73811241238545));
#29652=CARTESIAN_POINT('Ctrl Pts',(1.34854391898145,1.,1.73682580585819));
#29653=CARTESIAN_POINT('Ctrl Pts',(1.34824783113158,1.,1.73425417886255));
#29654=CARTESIAN_POINT('Ctrl Pts',(1.3477930915247,1.,1.73040149654497));
#29655=CARTESIAN_POINT('Ctrl Pts',(1.34716554820013,1.,1.72527410681298));
#29656=CARTESIAN_POINT('Ctrl Pts',(1.34634568653586,1.,1.7188807715095));
#29657=CARTESIAN_POINT('Ctrl Pts',(1.34549029589563,1.,1.71250340687011));
#29658=CARTESIAN_POINT('Ctrl Pts',(1.34459924533783,1.,1.70614212266676));
#29659=CARTESIAN_POINT('Ctrl Pts',(1.34367237124322,1.,1.69979707754221));
#29660=CARTESIAN_POINT('Ctrl Pts',(1.34270948206139,1.,1.6934684849664));
#29661=CARTESIAN_POINT('Ctrl Pts',(1.34171037484673,1.,1.68715660868602));
#29662=CARTESIAN_POINT('Ctrl Pts',(1.3406748518516,1.,1.68086176030308));
#29663=CARTESIAN_POINT('Ctrl Pts',(1.33960273470372,1.,1.67458429426126));
#29664=CARTESIAN_POINT('Ctrl Pts',(1.33849388654458,1.,1.66832460784078));
#29665=CARTESIAN_POINT('Ctrl Pts',(1.33734820885331,1.,1.66208312542073));
#29666=CARTESIAN_POINT('Ctrl Pts',(1.33616559745217,1.,1.65586025952651));
#29667=CARTESIAN_POINT('Ctrl Pts',(1.33494590468003,1.,1.64965637286843));
#29668=CARTESIAN_POINT('Ctrl Pts',(1.33368890676554,1.,1.64347174856007));
#29669=CARTESIAN_POINT('Ctrl Pts',(1.33239425103694,1.,1.6373065347505));
#29670=CARTESIAN_POINT('Ctrl Pts',(1.33106149345618,1.,1.63116079730887));
#29671=CARTESIAN_POINT('Ctrl Pts',(1.32969019505665,1.,1.62503464209777));
#29672=CARTESIAN_POINT('Ctrl Pts',(1.32828000610448,1.,1.61892832270723));
#29673=CARTESIAN_POINT('Ctrl Pts',(1.32683074483365,1.,1.61284234015762));
#29674=CARTESIAN_POINT('Ctrl Pts',(1.32534250785794,1.,1.6067775829097));
#29675=CARTESIAN_POINT('Ctrl Pts',(1.32381550858266,1.,1.600735118587));
#29676=CARTESIAN_POINT('Ctrl Pts',(1.32224985747686,1.,1.59471591079408));
#29677=CARTESIAN_POINT('Ctrl Pts',(1.32064537110891,1.,1.58872057258244));
#29678=CARTESIAN_POINT('Ctrl Pts',(1.31900135021428,1.,1.58274907898829));
#29679=CARTESIAN_POINT('Ctrl Pts',(1.31731642317183,1.,1.57680056505585));
#29680=CARTESIAN_POINT('Ctrl Pts',(1.31558903860015,1.,1.57087397835721));
#29681=CARTESIAN_POINT('Ctrl Pts',(1.31381795281002,1.,1.56496872402352));
#29682=CARTESIAN_POINT('Ctrl Pts',(1.31200264341696,1.,1.55908521254822));
#29683=CARTESIAN_POINT('Ctrl Pts',(1.31014393684221,1.,1.55322568759481));
#29684=CARTESIAN_POINT('Ctrl Pts',(1.30824393907471,1.,1.54739413957183));
#29685=CARTESIAN_POINT('Ctrl Pts',(1.30630475189553,1.,1.54159462645428));
#29686=CARTESIAN_POINT('Ctrl Pts',(1.30432735639487,1.,1.53582981268976));
#29687=CARTESIAN_POINT('Ctrl Pts',(1.3023106439557,1.,1.53009970283893));
#29688=CARTESIAN_POINT('Ctrl Pts',(1.30024984366334,1.,1.5243995786107));
#29689=CARTESIAN_POINT('Ctrl Pts',(1.29813791800757,1.,1.51872184912735));
#29690=CARTESIAN_POINT('Ctrl Pts',(1.29596850710518,1.,1.51305994241412));
#29691=CARTESIAN_POINT('Ctrl Pts',(1.29373841372843,1.,1.50741159078367));
#29692=CARTESIAN_POINT('Ctrl Pts',(1.29145022885171,1.,1.50178230149764));
#29693=CARTESIAN_POINT('Ctrl Pts',(1.28911506584232,1.,1.49618896881729));
#29694=CARTESIAN_POINT('Ctrl Pts',(1.28674676116415,1.,1.4906522831275));
#29695=CARTESIAN_POINT('Ctrl Pts',(1.28435533880184,1.,1.48518817118891));
#29696=CARTESIAN_POINT('Ctrl Pts',(1.28194158939522,1.,1.47980070347102));
#29697=CARTESIAN_POINT('Ctrl Pts',(1.27948918248524,1.,1.4744717526711));
#29698=CARTESIAN_POINT('Ctrl Pts',(1.27696414831144,1.,1.46916035917197));
#29699=CARTESIAN_POINT('Ctrl Pts',(1.27433119897877,1.,1.4638243133254));
#29700=CARTESIAN_POINT('Ctrl Pts',(1.27156805265312,1.,1.45843906294725));
#29701=CARTESIAN_POINT('Ctrl Pts',(1.26867786804854,1.,1.45301422764205));
#29702=CARTESIAN_POINT('Ctrl Pts',(1.26570925118767,1.,1.44761985001544));
#29703=CARTESIAN_POINT('Ctrl Pts',(1.26273903323723,1.,1.44236470511145));
#29704=CARTESIAN_POINT('Ctrl Pts',(1.25983531011894,1.,1.43734919180719));
#29705=CARTESIAN_POINT('Ctrl Pts',(1.25702687965744,1.,1.43262645609679));
#29706=CARTESIAN_POINT('Ctrl Pts',(1.25426945222783,1.,1.42815938799555));
#29707=CARTESIAN_POINT('Ctrl Pts',(1.25141455570299,1.,1.42378102115911));
#29708=CARTESIAN_POINT('Ctrl Pts',(1.24824430986911,1.,1.41923722596421));
#29709=CARTESIAN_POINT('Ctrl Pts',(1.24450600513278,1.,1.41422913175437));
#29710=CARTESIAN_POINT('Ctrl Pts',(1.23994455029421,1.,1.40845295531151));
#29711=CARTESIAN_POINT('Ctrl Pts',(1.23434087289768,1.,1.40164708205345));
#29712=CARTESIAN_POINT('Ctrl Pts',(1.22752961898063,1.,1.39361389567257));
#29713=CARTESIAN_POINT('Ctrl Pts',(1.21938737278853,1.,1.38420564525391));
#29714=CARTESIAN_POINT('Ctrl Pts',(1.20982812923113,1.,1.37331915604962));
#29715=CARTESIAN_POINT('Ctrl Pts',(1.1987959077656,1.,1.36088705040677));
#29716=CARTESIAN_POINT('Ctrl Pts',(1.18625865664915,1.,1.34687053998157));
#29717=CARTESIAN_POINT('Ctrl Pts',(1.17501305787994,1.,1.33437539344842));
#29718=CARTESIAN_POINT('Ctrl Pts',(1.16589330092532,1.,1.32428080720544));
#29719=CARTESIAN_POINT('Ctrl Pts',(1.15950888730433,1.,1.3172297721596));
#29720=CARTESIAN_POINT('Ctrl Pts',(1.15624053661742,1.,1.31362392696033));
#29721=CARTESIAN_POINT('',(1.34869019493419,0.,1.73811241238545));
#29722=CARTESIAN_POINT('Origin',(1.23627494547115,0.,1.81978687191668));
#29723=CARTESIAN_POINT('',(1.23627494547115,1.,1.81978687191668));
#29724=CARTESIAN_POINT('',(1.34869019493419,1.,1.73811241238545));
#29725=CARTESIAN_POINT('',(1.23627494547115,0.,1.81978687191668));
#29726=CARTESIAN_POINT('Ctrl Pts',(0.892032620296855,-1.,1.5055822144029));
#29727=CARTESIAN_POINT('Ctrl Pts',(0.892032620296855,1.,1.5055822144029));
#29728=CARTESIAN_POINT('Ctrl Pts',(0.894452006967538,-1.,1.50980486807181));
#29729=CARTESIAN_POINT('Ctrl Pts',(0.894452006967538,1.,1.50980486807181));
#29730=CARTESIAN_POINT('Ctrl Pts',(0.89918504749193,-1.,1.51805569591479));
#29731=CARTESIAN_POINT('Ctrl Pts',(0.89918504749193,1.,1.51805569591479));
#29732=CARTESIAN_POINT('Ctrl Pts',(0.905967409640498,-1.,1.52984849890434));
#29733=CARTESIAN_POINT('Ctrl Pts',(0.905967409640498,1.,1.52984849890434));
#29734=CARTESIAN_POINT('Ctrl Pts',(0.914375919046579,-1.,1.54440491152808));
#29735=CARTESIAN_POINT('Ctrl Pts',(0.914375919046579,1.,1.54440491152808));
#29736=CARTESIAN_POINT('Ctrl Pts',(0.923832188966322,-1.,1.56065988582509));
#29737=CARTESIAN_POINT('Ctrl Pts',(0.923832188966322,1.,1.56065988582509));
#29738=CARTESIAN_POINT('Ctrl Pts',(0.932246680128848,-1.,1.57499388385561));
#29739=CARTESIAN_POINT('Ctrl Pts',(0.932246680128848,1.,1.57499388385561));
#29740=CARTESIAN_POINT('Ctrl Pts',(0.939646377909319,-1.,1.58744937489796));
#29741=CARTESIAN_POINT('Ctrl Pts',(0.939646377909319,1.,1.58744937489796));
#29742=CARTESIAN_POINT('Ctrl Pts',(0.946078063325795,-1.,1.59810042045408));
#29743=CARTESIAN_POINT('Ctrl Pts',(0.946078063325795,1.,1.59810042045408));
#29744=CARTESIAN_POINT('Ctrl Pts',(0.951613284361247,-1.,1.60706069897794));
#29745=CARTESIAN_POINT('Ctrl Pts',(0.951613284361247,1.,1.60706069897794));
#29746=CARTESIAN_POINT('Ctrl Pts',(0.956354422921572,-1.,1.61449324337233));
#29747=CARTESIAN_POINT('Ctrl Pts',(0.956354422921572,1.,1.61449324337233));
#29748=CARTESIAN_POINT('Ctrl Pts',(0.960438326099958,-1.,1.62061638139929));
#29749=CARTESIAN_POINT('Ctrl Pts',(0.960438326099958,1.,1.62061638139929));
#29750=CARTESIAN_POINT('Ctrl Pts',(0.964046107037821,-1.,1.6257193066974));
#29751=CARTESIAN_POINT('Ctrl Pts',(0.964046107037821,1.,1.6257193066974));
#29752=CARTESIAN_POINT('Ctrl Pts',(0.967387853228041,-1.,1.63013849959083));
#29753=CARTESIAN_POINT('Ctrl Pts',(0.967387853228041,1.,1.63013849959083));
#29754=CARTESIAN_POINT('Ctrl Pts',(0.970669715996356,-1.,1.63420665729609));
#29755=CARTESIAN_POINT('Ctrl Pts',(0.970669715996356,1.,1.63420665729609));
#29756=CARTESIAN_POINT('Ctrl Pts',(0.974066058287501,-1.,1.63820952658157));
#29757=CARTESIAN_POINT('Ctrl Pts',(0.974066058287501,1.,1.63820952658157));
#29758=CARTESIAN_POINT('Ctrl Pts',(0.977689794120296,-1.,1.64233990826831));
#29759=CARTESIAN_POINT('Ctrl Pts',(0.977689794120296,1.,1.64233990826831));
#29760=CARTESIAN_POINT('Ctrl Pts',(0.981562530940574,-1.,1.64665139190834));
#29761=CARTESIAN_POINT('Ctrl Pts',(0.981562530940574,1.,1.64665139190834));
#29762=CARTESIAN_POINT('Ctrl Pts',(0.985642622921626,-1.,1.6511001661277));
#29763=CARTESIAN_POINT('Ctrl Pts',(0.985642622921626,1.,1.6511001661277));
#29764=CARTESIAN_POINT('Ctrl Pts',(0.98985562785445,-1.,1.65559044289746));
#29765=CARTESIAN_POINT('Ctrl Pts',(0.98985562785445,1.,1.65559044289746));
#29766=CARTESIAN_POINT('Ctrl Pts',(0.994121836661115,-1.,1.66001553809916));
#29767=CARTESIAN_POINT('Ctrl Pts',(0.994121836661115,1.,1.66001553809916));
#29768=CARTESIAN_POINT('Ctrl Pts',(0.998389654952317,-1.,1.66430758030304));
#29769=CARTESIAN_POINT('Ctrl Pts',(0.998389654952317,1.,1.66430758030304));
#29770=CARTESIAN_POINT('Ctrl Pts',(1.00265091003682,-1.,1.66846059277231));
#29771=CARTESIAN_POINT('Ctrl Pts',(1.00265091003682,1.,1.66846059277231));
#29772=CARTESIAN_POINT('Ctrl Pts',(1.00692206696387,-1.,1.67250335383248));
#29773=CARTESIAN_POINT('Ctrl Pts',(1.00692206696387,1.,1.67250335383248));
#29774=CARTESIAN_POINT('Ctrl Pts',(1.01123236493507,-1.,1.67648246776457));
#29775=CARTESIAN_POINT('Ctrl Pts',(1.01123236493507,1.,1.67648246776457));
#29776=CARTESIAN_POINT('Ctrl Pts',(1.01561026162786,-1.,1.6804428989482));
#29777=CARTESIAN_POINT('Ctrl Pts',(1.01561026162786,1.,1.6804428989482));
#29778=CARTESIAN_POINT('Ctrl Pts',(1.02006795074222,-1.,1.68440578021739));
#29779=CARTESIAN_POINT('Ctrl Pts',(1.02006795074222,1.,1.68440578021739));
#29780=CARTESIAN_POINT('Ctrl Pts',(1.02460180535272,-1.,1.68836910178475));
#29781=CARTESIAN_POINT('Ctrl Pts',(1.02460180535272,1.,1.68836910178475));
#29782=CARTESIAN_POINT('Ctrl Pts',(1.02919977579155,-1.,1.69231840863471));
#29783=CARTESIAN_POINT('Ctrl Pts',(1.02919977579155,1.,1.69231840863471));
#29784=CARTESIAN_POINT('Ctrl Pts',(1.03384646003587,-1.,1.69623414782769));
#29785=CARTESIAN_POINT('Ctrl Pts',(1.03384646003587,1.,1.69623414782769));
#29786=CARTESIAN_POINT('Ctrl Pts',(1.03852922490782,-1.,1.70010052930951));
#29787=CARTESIAN_POINT('Ctrl Pts',(1.03852922490782,1.,1.70010052930951));
#29788=CARTESIAN_POINT('Ctrl Pts',(1.04324363334546,-1.,1.70391338707969));
#29789=CARTESIAN_POINT('Ctrl Pts',(1.04324363334546,1.,1.70391338707969));
#29790=CARTESIAN_POINT('Ctrl Pts',(1.0479908540499,-1.,1.70767646263641));
#29791=CARTESIAN_POINT('Ctrl Pts',(1.0479908540499,1.,1.70767646263641));
#29792=CARTESIAN_POINT('Ctrl Pts',(1.05277517202853,-1.,1.71139783543986));
#29793=CARTESIAN_POINT('Ctrl Pts',(1.05277517202853,1.,1.71139783543986));
#29794=CARTESIAN_POINT('Ctrl Pts',(1.05760163192481,-1.,1.71508654427022));
#29795=CARTESIAN_POINT('Ctrl Pts',(1.05760163192481,1.,1.71508654427022));
#29796=CARTESIAN_POINT('Ctrl Pts',(1.06247324680649,-1.,1.71874858456908));
#29797=CARTESIAN_POINT('Ctrl Pts',(1.06247324680649,1.,1.71874858456908));
#29798=CARTESIAN_POINT('Ctrl Pts',(1.06738966975463,-1.,1.72238500928456));
#29799=CARTESIAN_POINT('Ctrl Pts',(1.06738966975463,1.,1.72238500928456));
#29800=CARTESIAN_POINT('Ctrl Pts',(1.07234866990252,-1.,1.72599406198489));
#29801=CARTESIAN_POINT('Ctrl Pts',(1.07234866990252,1.,1.72599406198489));
#29802=CARTESIAN_POINT('Ctrl Pts',(1.0773470373727,-1.,1.72957248977424));
#29803=CARTESIAN_POINT('Ctrl Pts',(1.0773470373727,1.,1.72957248977424));
#29804=CARTESIAN_POINT('Ctrl Pts',(1.08238162784749,-1.,1.73311705663407));
#29805=CARTESIAN_POINT('Ctrl Pts',(1.08238162784749,1.,1.73311705663407));
#29806=CARTESIAN_POINT('Ctrl Pts',(1.08745056285429,-1.,1.73662628326093));
#29807=CARTESIAN_POINT('Ctrl Pts',(1.08745056285429,1.,1.73662628326093));
#29808=CARTESIAN_POINT('Ctrl Pts',(1.09255329056496,-1.,1.74010053962252));
#29809=CARTESIAN_POINT('Ctrl Pts',(1.09255329056496,1.,1.74010053962252));
#29810=CARTESIAN_POINT('Ctrl Pts',(1.09768999241229,-1.,1.74354119236212));
#29811=CARTESIAN_POINT('Ctrl Pts',(1.09768999241229,1.,1.74354119236212));
#29812=CARTESIAN_POINT('Ctrl Pts',(1.10286118991144,-1.,1.74695004214924));
#29813=CARTESIAN_POINT('Ctrl Pts',(1.10286118991144,1.,1.74695004214924));
#29814=CARTESIAN_POINT('Ctrl Pts',(1.10806728183003,-1.,1.75032866075914));
#29815=CARTESIAN_POINT('Ctrl Pts',(1.10806728183003,1.,1.75032866075914));
#29816=CARTESIAN_POINT('Ctrl Pts',(1.11330807582542,-1.,1.75367772094617));
#29817=CARTESIAN_POINT('Ctrl Pts',(1.11330807582542,1.,1.75367772094617));
#29818=CARTESIAN_POINT('Ctrl Pts',(1.11858293216752,-1.,1.75699720772089));
#29819=CARTESIAN_POINT('Ctrl Pts',(1.11858293216752,1.,1.75699720772089));
#29820=CARTESIAN_POINT('Ctrl Pts',(1.12389096855078,-1.,1.76028671825084));
#29821=CARTESIAN_POINT('Ctrl Pts',(1.12389096855078,1.,1.76028671825084));
#29822=CARTESIAN_POINT('Ctrl Pts',(1.12923123555076,-1.,1.76354571966171));
#29823=CARTESIAN_POINT('Ctrl Pts',(1.12923123555076,1.,1.76354571966171));
#29824=CARTESIAN_POINT('Ctrl Pts',(1.13460291804634,-1.,1.76677384551883));
#29825=CARTESIAN_POINT('Ctrl Pts',(1.13460291804634,1.,1.76677384551883));
#29826=CARTESIAN_POINT('Ctrl Pts',(1.14000548337,-1.,1.76997111386806));
#29827=CARTESIAN_POINT('Ctrl Pts',(1.14000548337,1.,1.76997111386806));
#29828=CARTESIAN_POINT('Ctrl Pts',(1.14543858226948,-1.,1.77313777896234));
#29829=CARTESIAN_POINT('Ctrl Pts',(1.14543858226948,1.,1.77313777896234));
#29830=CARTESIAN_POINT('Ctrl Pts',(1.15090197841531,-1.,1.77627422557034));
#29831=CARTESIAN_POINT('Ctrl Pts',(1.15090197841531,1.,1.77627422557034));
#29832=CARTESIAN_POINT('Ctrl Pts',(1.15639547194689,-1.,1.77938085564261));
#29833=CARTESIAN_POINT('Ctrl Pts',(1.15639547194689,1.,1.77938085564261));
#29834=CARTESIAN_POINT('Ctrl Pts',(1.16191881298458,-1.,1.78245795880949));
#29835=CARTESIAN_POINT('Ctrl Pts',(1.16191881298458,1.,1.78245795880949));
#29836=CARTESIAN_POINT('Ctrl Pts',(1.16747166312239,-1.,1.78550566040349));
#29837=CARTESIAN_POINT('Ctrl Pts',(1.16747166312239,1.,1.78550566040349));
#29838=CARTESIAN_POINT('Ctrl Pts',(1.17305363177265,-1.,1.78852398877523));
#29839=CARTESIAN_POINT('Ctrl Pts',(1.17305363177265,1.,1.78852398877523));
#29840=CARTESIAN_POINT('Ctrl Pts',(1.17866429440781,-1.,1.79151291552646));
#29841=CARTESIAN_POINT('Ctrl Pts',(1.17866429440781,1.,1.79151291552646));
#29842=CARTESIAN_POINT('Ctrl Pts',(1.18430321697471,-1.,1.79447240321572));
#29843=CARTESIAN_POINT('Ctrl Pts',(1.18430321697471,1.,1.79447240321572));
#29844=CARTESIAN_POINT('Ctrl Pts',(1.1899699793456,-1.,1.79740245923649));
#29845=CARTESIAN_POINT('Ctrl Pts',(1.1899699793456,1.,1.79740245923649));
#29846=CARTESIAN_POINT('Ctrl Pts',(1.19566418930405,-1.,1.80030314370121));
#29847=CARTESIAN_POINT('Ctrl Pts',(1.19566418930405,1.,1.80030314370121));
#29848=CARTESIAN_POINT('Ctrl Pts',(1.2013854893912,-1.,1.8031745483882));
#29849=CARTESIAN_POINT('Ctrl Pts',(1.2013854893912,1.,1.8031745483882));
#29850=CARTESIAN_POINT('Ctrl Pts',(1.20713356605519,-1.,1.80601678480772));
#29851=CARTESIAN_POINT('Ctrl Pts',(1.20713356605519,1.,1.80601678480772));
#29852=CARTESIAN_POINT('Ctrl Pts',(1.2129081570818,-1.,1.80882996916931));
#29853=CARTESIAN_POINT('Ctrl Pts',(1.2129081570818,1.,1.80882996916931));
#29854=CARTESIAN_POINT('Ctrl Pts',(1.2187090610323,-1.,1.81161420806172));
#29855=CARTESIAN_POINT('Ctrl Pts',(1.2187090610323,1.,1.81161420806172));
#29856=CARTESIAN_POINT('Ctrl Pts',(1.22453613304507,-1.,1.81436959209778));
#29857=CARTESIAN_POINT('Ctrl Pts',(1.22453613304507,1.,1.81436959209778));
#29858=CARTESIAN_POINT('Ctrl Pts',(1.22921864890975,-1.,1.81655087183054));
#29859=CARTESIAN_POINT('Ctrl Pts',(1.22921864890975,1.,1.81655087183054));
#29860=CARTESIAN_POINT('Ctrl Pts',(1.23274224526804,-1.,1.81817389920914));
#29861=CARTESIAN_POINT('Ctrl Pts',(1.23274224526804,1.,1.81817389920914));
#29862=CARTESIAN_POINT('Ctrl Pts',(1.23509651170384,-1.,1.81925017193531));
#29863=CARTESIAN_POINT('Ctrl Pts',(1.23509651170384,1.,1.81925017193531));
#29864=CARTESIAN_POINT('Ctrl Pts',(1.23627494547115,-1.,1.81978687191668));
#29865=CARTESIAN_POINT('Ctrl Pts',(1.23627494547115,1.,1.81978687191668));
#29866=CARTESIAN_POINT('',(0.892032620296855,1.,1.5055822144029));
#29867=CARTESIAN_POINT('Ctrl Pts',(0.892032620296855,1.,1.5055822144029));
#29868=CARTESIAN_POINT('Ctrl Pts',(0.894452006967538,1.,1.50980486807181));
#29869=CARTESIAN_POINT('Ctrl Pts',(0.89918504749193,1.,1.51805569591479));
#29870=CARTESIAN_POINT('Ctrl Pts',(0.905967409640498,1.,1.52984849890434));
#29871=CARTESIAN_POINT('Ctrl Pts',(0.914375919046579,1.,1.54440491152808));
#29872=CARTESIAN_POINT('Ctrl Pts',(0.923832188966322,1.,1.56065988582509));
#29873=CARTESIAN_POINT('Ctrl Pts',(0.932246680128848,1.,1.57499388385561));
#29874=CARTESIAN_POINT('Ctrl Pts',(0.939646377909319,1.,1.58744937489796));
#29875=CARTESIAN_POINT('Ctrl Pts',(0.946078063325795,1.,1.59810042045408));
#29876=CARTESIAN_POINT('Ctrl Pts',(0.951613284361247,1.,1.60706069897794));
#29877=CARTESIAN_POINT('Ctrl Pts',(0.956354422921572,1.,1.61449324337233));
#29878=CARTESIAN_POINT('Ctrl Pts',(0.960438326099958,1.,1.62061638139929));
#29879=CARTESIAN_POINT('Ctrl Pts',(0.964046107037821,1.,1.6257193066974));
#29880=CARTESIAN_POINT('Ctrl Pts',(0.967387853228041,1.,1.63013849959083));
#29881=CARTESIAN_POINT('Ctrl Pts',(0.970669715996356,1.,1.63420665729609));
#29882=CARTESIAN_POINT('Ctrl Pts',(0.974066058287501,1.,1.63820952658157));
#29883=CARTESIAN_POINT('Ctrl Pts',(0.977689794120296,1.,1.64233990826831));
#29884=CARTESIAN_POINT('Ctrl Pts',(0.981562530940574,1.,1.64665139190834));
#29885=CARTESIAN_POINT('Ctrl Pts',(0.985642622921626,1.,1.6511001661277));
#29886=CARTESIAN_POINT('Ctrl Pts',(0.98985562785445,1.,1.65559044289746));
#29887=CARTESIAN_POINT('Ctrl Pts',(0.994121836661115,1.,1.66001553809916));
#29888=CARTESIAN_POINT('Ctrl Pts',(0.998389654952317,1.,1.66430758030304));
#29889=CARTESIAN_POINT('Ctrl Pts',(1.00265091003682,1.,1.66846059277231));
#29890=CARTESIAN_POINT('Ctrl Pts',(1.00692206696387,1.,1.67250335383248));
#29891=CARTESIAN_POINT('Ctrl Pts',(1.01123236493507,1.,1.67648246776457));
#29892=CARTESIAN_POINT('Ctrl Pts',(1.01561026162786,1.,1.6804428989482));
#29893=CARTESIAN_POINT('Ctrl Pts',(1.02006795074222,1.,1.68440578021739));
#29894=CARTESIAN_POINT('Ctrl Pts',(1.02460180535272,1.,1.68836910178475));
#29895=CARTESIAN_POINT('Ctrl Pts',(1.02919977579155,1.,1.69231840863471));
#29896=CARTESIAN_POINT('Ctrl Pts',(1.03384646003587,1.,1.69623414782769));
#29897=CARTESIAN_POINT('Ctrl Pts',(1.03852922490782,1.,1.70010052930951));
#29898=CARTESIAN_POINT('Ctrl Pts',(1.04324363334546,1.,1.70391338707969));
#29899=CARTESIAN_POINT('Ctrl Pts',(1.0479908540499,1.,1.70767646263641));
#29900=CARTESIAN_POINT('Ctrl Pts',(1.05277517202853,1.,1.71139783543986));
#29901=CARTESIAN_POINT('Ctrl Pts',(1.05760163192481,1.,1.71508654427022));
#29902=CARTESIAN_POINT('Ctrl Pts',(1.06247324680649,1.,1.71874858456908));
#29903=CARTESIAN_POINT('Ctrl Pts',(1.06738966975463,1.,1.72238500928456));
#29904=CARTESIAN_POINT('Ctrl Pts',(1.07234866990252,1.,1.72599406198489));
#29905=CARTESIAN_POINT('Ctrl Pts',(1.0773470373727,1.,1.72957248977424));
#29906=CARTESIAN_POINT('Ctrl Pts',(1.08238162784749,1.,1.73311705663407));
#29907=CARTESIAN_POINT('Ctrl Pts',(1.08745056285429,1.,1.73662628326093));
#29908=CARTESIAN_POINT('Ctrl Pts',(1.09255329056496,1.,1.74010053962252));
#29909=CARTESIAN_POINT('Ctrl Pts',(1.09768999241229,1.,1.74354119236212));
#29910=CARTESIAN_POINT('Ctrl Pts',(1.10286118991144,1.,1.74695004214924));
#29911=CARTESIAN_POINT('Ctrl Pts',(1.10806728183003,1.,1.75032866075914));
#29912=CARTESIAN_POINT('Ctrl Pts',(1.11330807582542,1.,1.75367772094617));
#29913=CARTESIAN_POINT('Ctrl Pts',(1.11858293216752,1.,1.75699720772089));
#29914=CARTESIAN_POINT('Ctrl Pts',(1.12389096855078,1.,1.76028671825084));
#29915=CARTESIAN_POINT('Ctrl Pts',(1.12923123555076,1.,1.76354571966171));
#29916=CARTESIAN_POINT('Ctrl Pts',(1.13460291804634,1.,1.76677384551883));
#29917=CARTESIAN_POINT('Ctrl Pts',(1.14000548337,1.,1.76997111386806));
#29918=CARTESIAN_POINT('Ctrl Pts',(1.14543858226948,1.,1.77313777896234));
#29919=CARTESIAN_POINT('Ctrl Pts',(1.15090197841531,1.,1.77627422557034));
#29920=CARTESIAN_POINT('Ctrl Pts',(1.15639547194689,1.,1.77938085564261));
#29921=CARTESIAN_POINT('Ctrl Pts',(1.16191881298458,1.,1.78245795880949));
#29922=CARTESIAN_POINT('Ctrl Pts',(1.16747166312239,1.,1.78550566040349));
#29923=CARTESIAN_POINT('Ctrl Pts',(1.17305363177265,1.,1.78852398877523));
#29924=CARTESIAN_POINT('Ctrl Pts',(1.17866429440781,1.,1.79151291552646));
#29925=CARTESIAN_POINT('Ctrl Pts',(1.18430321697471,1.,1.79447240321572));
#29926=CARTESIAN_POINT('Ctrl Pts',(1.1899699793456,1.,1.79740245923649));
#29927=CARTESIAN_POINT('Ctrl Pts',(1.19566418930405,1.,1.80030314370121));
#29928=CARTESIAN_POINT('Ctrl Pts',(1.2013854893912,1.,1.8031745483882));
#29929=CARTESIAN_POINT('Ctrl Pts',(1.20713356605519,1.,1.80601678480772));
#29930=CARTESIAN_POINT('Ctrl Pts',(1.2129081570818,1.,1.80882996916931));
#29931=CARTESIAN_POINT('Ctrl Pts',(1.2187090610323,1.,1.81161420806172));
#29932=CARTESIAN_POINT('Ctrl Pts',(1.22453613304507,1.,1.81436959209778));
#29933=CARTESIAN_POINT('Ctrl Pts',(1.22921864890975,1.,1.81655087183054));
#29934=CARTESIAN_POINT('Ctrl Pts',(1.23274224526804,1.,1.81817389920914));
#29935=CARTESIAN_POINT('Ctrl Pts',(1.23509651170384,1.,1.81925017193531));
#29936=CARTESIAN_POINT('Ctrl Pts',(1.23627494547115,1.,1.81978687191668));
#29937=CARTESIAN_POINT('',(0.892032620296854,0.,1.5055822144029));
#29938=CARTESIAN_POINT('Origin',(0.,0.,0.));
#29939=CARTESIAN_POINT('',(0.693717979106305,1.,1.60662857109684));
#29940=CARTESIAN_POINT('Origin',(0.,1.,0.));
#29941=CARTESIAN_POINT('',(0.693717979106305,0.,1.60662857109684));
#29942=CARTESIAN_POINT('Ctrl Pts',(0.7455743247944,-1.,2.0698113262342));
#29943=CARTESIAN_POINT('Ctrl Pts',(0.7455743247944,1.,2.0698113262342));
#29944=CARTESIAN_POINT('Ctrl Pts',(0.745832791378367,-1.,2.06854248895728));
#29945=CARTESIAN_POINT('Ctrl Pts',(0.745832791378367,1.,2.06854248895728));
#29946=CARTESIAN_POINT('Ctrl Pts',(0.7463458715442,-1.,2.06600523016815));
#29947=CARTESIAN_POINT('Ctrl Pts',(0.7463458715442,1.,2.06600523016815));
#29948=CARTESIAN_POINT('Ctrl Pts',(0.747103932787919,-1.,2.06220058927826));
#29949=CARTESIAN_POINT('Ctrl Pts',(0.747103932787919,1.,2.06220058927826));
#29950=CARTESIAN_POINT('Ctrl Pts',(0.748091554183802,-1.,2.05713023031007));
#29951=CARTESIAN_POINT('Ctrl Pts',(0.748091554183802,1.,2.05713023031007));
#29952=CARTESIAN_POINT('Ctrl Pts',(0.749287468665046,-1.,2.05079645592154));
#29953=CARTESIAN_POINT('Ctrl Pts',(0.749287468665046,1.,2.05079645592154));
#29954=CARTESIAN_POINT('Ctrl Pts',(0.750444657875575,-1.,2.04446689147979));
#29955=CARTESIAN_POINT('Ctrl Pts',(0.750444657875575,1.,2.04446689147979));
#29956=CARTESIAN_POINT('Ctrl Pts',(0.751562963361115,-1.,2.03814160092099));
#29957=CARTESIAN_POINT('Ctrl Pts',(0.751562963361115,1.,2.03814160092099));
#29958=CARTESIAN_POINT('Ctrl Pts',(0.75264218048721,-1.,2.03182068456221));
#29959=CARTESIAN_POINT('Ctrl Pts',(0.75264218048721,1.,2.03182068456221));
#29960=CARTESIAN_POINT('Ctrl Pts',(0.753682061112768,-1.,2.02550428623313));
#29961=CARTESIAN_POINT('Ctrl Pts',(0.753682061112768,1.,2.02550428623313));
#29962=CARTESIAN_POINT('Ctrl Pts',(0.754682330722816,-1.,2.01919259405809));
#29963=CARTESIAN_POINT('Ctrl Pts',(0.754682330722816,1.,2.01919259405809));
#29964=CARTESIAN_POINT('Ctrl Pts',(0.755642704957865,-1.,2.01288584328084));
#29965=CARTESIAN_POINT('Ctrl Pts',(0.755642704957865,1.,2.01288584328084));
#29966=CARTESIAN_POINT('Ctrl Pts',(0.75656290464667,-1.,2.0065843158773));
#29967=CARTESIAN_POINT('Ctrl Pts',(0.75656290464667,1.,2.0065843158773));
#29968=CARTESIAN_POINT('Ctrl Pts',(0.757442676862724,-1.,2.00028834739178));
#29969=CARTESIAN_POINT('Ctrl Pts',(0.757442676862724,1.,2.00028834739178));
#29970=CARTESIAN_POINT('Ctrl Pts',(0.758281796766761,-1.,1.99399831098817));
#29971=CARTESIAN_POINT('Ctrl Pts',(0.758281796766761,1.,1.99399831098817));
#29972=CARTESIAN_POINT('Ctrl Pts',(0.759080037802488,-1.,1.98771456680874));
#29973=CARTESIAN_POINT('Ctrl Pts',(0.759080037802488,1.,1.98771456680874));
#29974=CARTESIAN_POINT('Ctrl Pts',(0.75983714745219,-1.,1.98143741418172));
#29975=CARTESIAN_POINT('Ctrl Pts',(0.75983714745219,1.,1.98143741418172));
#29976=CARTESIAN_POINT('Ctrl Pts',(0.760552825409757,-1.,1.97516705321494));
#29977=CARTESIAN_POINT('Ctrl Pts',(0.760552825409757,1.,1.97516705321494));
#29978=CARTESIAN_POINT('Ctrl Pts',(0.76122669048382,-1.,1.96890351582499));
#29979=CARTESIAN_POINT('Ctrl Pts',(0.76122669048382,1.,1.96890351582499));
#29980=CARTESIAN_POINT('Ctrl Pts',(0.761858300014423,-1.,1.96264672744186));
#29981=CARTESIAN_POINT('Ctrl Pts',(0.761858300014423,1.,1.96264672744186));
#29982=CARTESIAN_POINT('Ctrl Pts',(0.762447203806178,-1.,1.95639665309869));
#29983=CARTESIAN_POINT('Ctrl Pts',(0.762447203806178,1.,1.95639665309869));
#29984=CARTESIAN_POINT('Ctrl Pts',(0.762992990878769,-1.,1.95015342590024));
#29985=CARTESIAN_POINT('Ctrl Pts',(0.762992990878769,1.,1.95015342590024));
#29986=CARTESIAN_POINT('Ctrl Pts',(0.763495333538629,-1.,1.9439174661764));
#29987=CARTESIAN_POINT('Ctrl Pts',(0.763495333538629,1.,1.9439174661764));
#29988=CARTESIAN_POINT('Ctrl Pts',(0.763954049121458,-1.,1.93768964875886));
#29989=CARTESIAN_POINT('Ctrl Pts',(0.763954049121458,1.,1.93768964875886));
#29990=CARTESIAN_POINT('Ctrl Pts',(0.76436901067394,-1.,1.93147105496382));
#29991=CARTESIAN_POINT('Ctrl Pts',(0.76436901067394,1.,1.93147105496382));
#29992=CARTESIAN_POINT('Ctrl Pts',(0.764740025488211,-1.,1.92526263537048));
#29993=CARTESIAN_POINT('Ctrl Pts',(0.764740025488211,1.,1.92526263537048));
#29994=CARTESIAN_POINT('Ctrl Pts',(0.765066729667088,-1.,1.91906491634196));
#29995=CARTESIAN_POINT('Ctrl Pts',(0.765066729667088,1.,1.91906491634196));
#29996=CARTESIAN_POINT('Ctrl Pts',(0.765348465884722,-1.,1.91287765805169));
#29997=CARTESIAN_POINT('Ctrl Pts',(0.765348465884722,1.,1.91287765805169));
#29998=CARTESIAN_POINT('Ctrl Pts',(0.765584196937919,-1.,1.90669961402356));
#29999=CARTESIAN_POINT('Ctrl Pts',(0.765584196937919,1.,1.90669961402356));
#30000=CARTESIAN_POINT('Ctrl Pts',(0.765772772593386,-1.,1.90052930393596));
#30001=CARTESIAN_POINT('Ctrl Pts',(0.765772772593386,1.,1.90052930393596));
#30002=CARTESIAN_POINT('Ctrl Pts',(0.765913193856978,-1.,1.89436577771388));
#30003=CARTESIAN_POINT('Ctrl Pts',(0.765913193856978,1.,1.89436577771388));
#30004=CARTESIAN_POINT('Ctrl Pts',(0.766004837062091,-1.,1.88820926433409));
#30005=CARTESIAN_POINT('Ctrl Pts',(0.766004837062091,1.,1.88820926433409));
#30006=CARTESIAN_POINT('Ctrl Pts',(0.766047794851864,-1.,1.88206215302561));
#30007=CARTESIAN_POINT('Ctrl Pts',(0.766047794851864,1.,1.88206215302561));
#30008=CARTESIAN_POINT('Ctrl Pts',(0.766042837036744,-1.,1.87592888967883));
#30009=CARTESIAN_POINT('Ctrl Pts',(0.766042837036744,1.,1.87592888967883));
#30010=CARTESIAN_POINT('Ctrl Pts',(0.765990708546091,-1.,1.86981398314341));
#30011=CARTESIAN_POINT('Ctrl Pts',(0.765990708546091,1.,1.86981398314341));
#30012=CARTESIAN_POINT('Ctrl Pts',(0.765891519092547,-1.,1.86372027063312));
#30013=CARTESIAN_POINT('Ctrl Pts',(0.765891519092547,1.,1.86372027063312));
#30014=CARTESIAN_POINT('Ctrl Pts',(0.765744212909318,-1.,1.85764741390394));
#30015=CARTESIAN_POINT('Ctrl Pts',(0.765744212909318,1.,1.85764741390394));
#30016=CARTESIAN_POINT('Ctrl Pts',(0.765545710619062,-1.,1.85158945130063));
#30017=CARTESIAN_POINT('Ctrl Pts',(0.765545710619062,1.,1.85158945130063));
#30018=CARTESIAN_POINT('Ctrl Pts',(0.765291664862029,-1.,1.84553698875924));
#30019=CARTESIAN_POINT('Ctrl Pts',(0.765291664862029,1.,1.84553698875924));
#30020=CARTESIAN_POINT('Ctrl Pts',(0.764978057881737,-1.,1.83948181064835));
#30021=CARTESIAN_POINT('Ctrl Pts',(0.764978057881737,1.,1.83948181064835));
#30022=CARTESIAN_POINT('Ctrl Pts',(0.764602549687853,-1.,1.83342077227142));
#30023=CARTESIAN_POINT('Ctrl Pts',(0.764602549687853,1.,1.83342077227142));
#30024=CARTESIAN_POINT('Ctrl Pts',(0.764165902605995,-1.,1.82735991200065));
#30025=CARTESIAN_POINT('Ctrl Pts',(0.764165902605995,1.,1.82735991200065));
#30026=CARTESIAN_POINT('Ctrl Pts',(0.763673465462726,-1.,1.82131873145266));
#30027=CARTESIAN_POINT('Ctrl Pts',(0.763673465462726,1.,1.82131873145266));
#30028=CARTESIAN_POINT('Ctrl Pts',(0.763132003836634,-1.,1.8153211840553));
#30029=CARTESIAN_POINT('Ctrl Pts',(0.763132003836634,1.,1.8153211840553));
#30030=CARTESIAN_POINT('Ctrl Pts',(0.762546129463938,-1.,1.80938551463965));
#30031=CARTESIAN_POINT('Ctrl Pts',(0.762546129463938,1.,1.80938551463965));
#30032=CARTESIAN_POINT('Ctrl Pts',(0.761915336443547,-1.,1.80351583877342));
#30033=CARTESIAN_POINT('Ctrl Pts',(0.761915336443547,1.,1.80351583877342));
#30034=CARTESIAN_POINT('Ctrl Pts',(0.761229695230558,-1.,1.79768986997783));
#30035=CARTESIAN_POINT('Ctrl Pts',(0.761229695230558,1.,1.79768986997783));
#30036=CARTESIAN_POINT('Ctrl Pts',(0.760469555880749,-1.,1.7918581561088));
#30037=CARTESIAN_POINT('Ctrl Pts',(0.760469555880749,1.,1.7918581561088));
#30038=CARTESIAN_POINT('Ctrl Pts',(0.759614401110189,-1.,1.78596964884604));
#30039=CARTESIAN_POINT('Ctrl Pts',(0.759614401110189,1.,1.78596964884604));
#30040=CARTESIAN_POINT('Ctrl Pts',(0.758650626677518,-1.,1.77999411220945));
#30041=CARTESIAN_POINT('Ctrl Pts',(0.758650626677518,1.,1.77999411220945));
#30042=CARTESIAN_POINT('Ctrl Pts',(0.757578264077028,-1.,1.77394167108292));
#30043=CARTESIAN_POINT('Ctrl Pts',(0.757578264077028,1.,1.77394167108292));
#30044=CARTESIAN_POINT('Ctrl Pts',(0.75642189602781,-1.,1.76789396002998));
#30045=CARTESIAN_POINT('Ctrl Pts',(0.75642189602781,1.,1.76789396002998));
#30046=CARTESIAN_POINT('Ctrl Pts',(0.755220979974461,-1.,1.76197817240128));
#30047=CARTESIAN_POINT('Ctrl Pts',(0.755220979974461,1.,1.76197817240128));
#30048=CARTESIAN_POINT('Ctrl Pts',(0.754009254027828,-1.,1.75631083600019));
#30049=CARTESIAN_POINT('Ctrl Pts',(0.754009254027828,1.,1.75631083600019));
#30050=CARTESIAN_POINT('Ctrl Pts',(0.752797683531314,-1.,1.75095139468794));
#30051=CARTESIAN_POINT('Ctrl Pts',(0.752797683531314,1.,1.75095139468794));
#30052=CARTESIAN_POINT('Ctrl Pts',(0.751555614164482,-1.,1.74585086852502));
#30053=CARTESIAN_POINT('Ctrl Pts',(0.751555614164482,1.,1.74585086852502));
#30054=CARTESIAN_POINT('Ctrl Pts',(0.750193435981249,-1.,1.74080458267114));
#30055=CARTESIAN_POINT('Ctrl Pts',(0.750193435981249,1.,1.74080458267114));
#30056=CARTESIAN_POINT('Ctrl Pts',(0.74858246295687,-1.,1.7355035168033));
#30057=CARTESIAN_POINT('Ctrl Pts',(0.74858246295687,1.,1.7355035168033));
#30058=CARTESIAN_POINT('Ctrl Pts',(0.746574710097752,-1.,1.72958533647714));
#30059=CARTESIAN_POINT('Ctrl Pts',(0.746574710097752,1.,1.72958533647714));
#30060=CARTESIAN_POINT('Ctrl Pts',(0.744021445433093,-1.,1.72268229916769));
#30061=CARTESIAN_POINT('Ctrl Pts',(0.744021445433093,1.,1.72268229916769));
#30062=CARTESIAN_POINT('Ctrl Pts',(0.74079516202821,-1.,1.71447789751001));
#30063=CARTESIAN_POINT('Ctrl Pts',(0.74079516202821,1.,1.71447789751001));
#30064=CARTESIAN_POINT('Ctrl Pts',(0.736799665716932,-1.,1.70473309004249));
#30065=CARTESIAN_POINT('Ctrl Pts',(0.736799665716932,1.,1.70473309004249));
#30066=CARTESIAN_POINT('Ctrl Pts',(0.731963238685357,-1.,1.69326921972915));
#30067=CARTESIAN_POINT('Ctrl Pts',(0.731963238685357,1.,1.69326921972915));
#30068=CARTESIAN_POINT('Ctrl Pts',(0.726235967982445,-1.,1.67996158451922));
#30069=CARTESIAN_POINT('Ctrl Pts',(0.726235967982445,1.,1.67996158451922));
#30070=CARTESIAN_POINT('Ctrl Pts',(0.719585433787949,-1.,1.66472880551777));
#30071=CARTESIAN_POINT('Ctrl Pts',(0.719585433787949,1.,1.66472880551777));
#30072=CARTESIAN_POINT('Ctrl Pts',(0.711993139340447,-1.,1.64752408828442));
#30073=CARTESIAN_POINT('Ctrl Pts',(0.711993139340447,1.,1.64752408828442));
#30074=CARTESIAN_POINT('Ctrl Pts',(0.705159151977294,-1.,1.6321654166204));
#30075=CARTESIAN_POINT('Ctrl Pts',(0.705159151977294,1.,1.6321654166204));
#30076=CARTESIAN_POINT('Ctrl Pts',(0.699605146398836,-1.,1.61974673471117));
#30077=CARTESIAN_POINT('Ctrl Pts',(0.699605146398836,1.,1.61974673471117));
#30078=CARTESIAN_POINT('Ctrl Pts',(0.69571209787897,-1.,1.61106790957619));
#30079=CARTESIAN_POINT('Ctrl Pts',(0.69571209787897,1.,1.61106790957619));
#30080=CARTESIAN_POINT('Ctrl Pts',(0.693717979106305,-1.,1.60662857109684));
#30081=CARTESIAN_POINT('Ctrl Pts',(0.693717979106305,1.,1.60662857109684));
#30082=CARTESIAN_POINT('',(0.7455743247944,1.,2.0698113262342));
#30083=CARTESIAN_POINT('Ctrl Pts',(0.7455743247944,1.,2.0698113262342));
#30084=CARTESIAN_POINT('Ctrl Pts',(0.745832791378367,1.,2.06854248895728));
#30085=CARTESIAN_POINT('Ctrl Pts',(0.7463458715442,1.,2.06600523016815));
#30086=CARTESIAN_POINT('Ctrl Pts',(0.747103932787919,1.,2.06220058927826));
#30087=CARTESIAN_POINT('Ctrl Pts',(0.748091554183802,1.,2.05713023031007));
#30088=CARTESIAN_POINT('Ctrl Pts',(0.749287468665046,1.,2.05079645592154));
#30089=CARTESIAN_POINT('Ctrl Pts',(0.750444657875575,1.,2.04446689147979));
#30090=CARTESIAN_POINT('Ctrl Pts',(0.751562963361115,1.,2.03814160092099));
#30091=CARTESIAN_POINT('Ctrl Pts',(0.75264218048721,1.,2.03182068456221));
#30092=CARTESIAN_POINT('Ctrl Pts',(0.753682061112768,1.,2.02550428623313));
#30093=CARTESIAN_POINT('Ctrl Pts',(0.754682330722816,1.,2.01919259405809));
#30094=CARTESIAN_POINT('Ctrl Pts',(0.755642704957865,1.,2.01288584328084));
#30095=CARTESIAN_POINT('Ctrl Pts',(0.75656290464667,1.,2.0065843158773));
#30096=CARTESIAN_POINT('Ctrl Pts',(0.757442676862724,1.,2.00028834739178));
#30097=CARTESIAN_POINT('Ctrl Pts',(0.758281796766761,1.,1.99399831098817));
#30098=CARTESIAN_POINT('Ctrl Pts',(0.759080037802488,1.,1.98771456680874));
#30099=CARTESIAN_POINT('Ctrl Pts',(0.75983714745219,1.,1.98143741418172));
#30100=CARTESIAN_POINT('Ctrl Pts',(0.760552825409757,1.,1.97516705321494));
#30101=CARTESIAN_POINT('Ctrl Pts',(0.76122669048382,1.,1.96890351582499));
#30102=CARTESIAN_POINT('Ctrl Pts',(0.761858300014423,1.,1.96264672744186));
#30103=CARTESIAN_POINT('Ctrl Pts',(0.762447203806178,1.,1.95639665309869));
#30104=CARTESIAN_POINT('Ctrl Pts',(0.762992990878769,1.,1.95015342590024));
#30105=CARTESIAN_POINT('Ctrl Pts',(0.763495333538629,1.,1.9439174661764));
#30106=CARTESIAN_POINT('Ctrl Pts',(0.763954049121458,1.,1.93768964875886));
#30107=CARTESIAN_POINT('Ctrl Pts',(0.76436901067394,1.,1.93147105496382));
#30108=CARTESIAN_POINT('Ctrl Pts',(0.764740025488211,1.,1.92526263537048));
#30109=CARTESIAN_POINT('Ctrl Pts',(0.765066729667088,1.,1.91906491634196));
#30110=CARTESIAN_POINT('Ctrl Pts',(0.765348465884722,1.,1.91287765805169));
#30111=CARTESIAN_POINT('Ctrl Pts',(0.765584196937919,1.,1.90669961402356));
#30112=CARTESIAN_POINT('Ctrl Pts',(0.765772772593386,1.,1.90052930393596));
#30113=CARTESIAN_POINT('Ctrl Pts',(0.765913193856978,1.,1.89436577771388));
#30114=CARTESIAN_POINT('Ctrl Pts',(0.766004837062091,1.,1.88820926433409));
#30115=CARTESIAN_POINT('Ctrl Pts',(0.766047794851864,1.,1.88206215302561));
#30116=CARTESIAN_POINT('Ctrl Pts',(0.766042837036744,1.,1.87592888967883));
#30117=CARTESIAN_POINT('Ctrl Pts',(0.765990708546091,1.,1.86981398314341));
#30118=CARTESIAN_POINT('Ctrl Pts',(0.765891519092547,1.,1.86372027063312));
#30119=CARTESIAN_POINT('Ctrl Pts',(0.765744212909318,1.,1.85764741390394));
#30120=CARTESIAN_POINT('Ctrl Pts',(0.765545710619062,1.,1.85158945130063));
#30121=CARTESIAN_POINT('Ctrl Pts',(0.765291664862029,1.,1.84553698875924));
#30122=CARTESIAN_POINT('Ctrl Pts',(0.764978057881737,1.,1.83948181064835));
#30123=CARTESIAN_POINT('Ctrl Pts',(0.764602549687853,1.,1.83342077227142));
#30124=CARTESIAN_POINT('Ctrl Pts',(0.764165902605995,1.,1.82735991200065));
#30125=CARTESIAN_POINT('Ctrl Pts',(0.763673465462726,1.,1.82131873145266));
#30126=CARTESIAN_POINT('Ctrl Pts',(0.763132003836634,1.,1.8153211840553));
#30127=CARTESIAN_POINT('Ctrl Pts',(0.762546129463938,1.,1.80938551463965));
#30128=CARTESIAN_POINT('Ctrl Pts',(0.761915336443547,1.,1.80351583877342));
#30129=CARTESIAN_POINT('Ctrl Pts',(0.761229695230558,1.,1.79768986997783));
#30130=CARTESIAN_POINT('Ctrl Pts',(0.760469555880749,1.,1.7918581561088));
#30131=CARTESIAN_POINT('Ctrl Pts',(0.759614401110189,1.,1.78596964884604));
#30132=CARTESIAN_POINT('Ctrl Pts',(0.758650626677518,1.,1.77999411220945));
#30133=CARTESIAN_POINT('Ctrl Pts',(0.757578264077028,1.,1.77394167108292));
#30134=CARTESIAN_POINT('Ctrl Pts',(0.75642189602781,1.,1.76789396002998));
#30135=CARTESIAN_POINT('Ctrl Pts',(0.755220979974461,1.,1.76197817240128));
#30136=CARTESIAN_POINT('Ctrl Pts',(0.754009254027828,1.,1.75631083600019));
#30137=CARTESIAN_POINT('Ctrl Pts',(0.752797683531314,1.,1.75095139468794));
#30138=CARTESIAN_POINT('Ctrl Pts',(0.751555614164482,1.,1.74585086852502));
#30139=CARTESIAN_POINT('Ctrl Pts',(0.750193435981249,1.,1.74080458267114));
#30140=CARTESIAN_POINT('Ctrl Pts',(0.74858246295687,1.,1.7355035168033));
#30141=CARTESIAN_POINT('Ctrl Pts',(0.746574710097752,1.,1.72958533647714));
#30142=CARTESIAN_POINT('Ctrl Pts',(0.744021445433093,1.,1.72268229916769));
#30143=CARTESIAN_POINT('Ctrl Pts',(0.74079516202821,1.,1.71447789751001));
#30144=CARTESIAN_POINT('Ctrl Pts',(0.736799665716932,1.,1.70473309004249));
#30145=CARTESIAN_POINT('Ctrl Pts',(0.731963238685357,1.,1.69326921972915));
#30146=CARTESIAN_POINT('Ctrl Pts',(0.726235967982445,1.,1.67996158451922));
#30147=CARTESIAN_POINT('Ctrl Pts',(0.719585433787949,1.,1.66472880551777));
#30148=CARTESIAN_POINT('Ctrl Pts',(0.711993139340447,1.,1.64752408828442));
#30149=CARTESIAN_POINT('Ctrl Pts',(0.705159151977294,1.,1.6321654166204));
#30150=CARTESIAN_POINT('Ctrl Pts',(0.699605146398836,1.,1.61974673471117));
#30151=CARTESIAN_POINT('Ctrl Pts',(0.69571209787897,1.,1.61106790957619));
#30152=CARTESIAN_POINT('Ctrl Pts',(0.693717979106305,1.,1.60662857109684));
#30153=CARTESIAN_POINT('',(0.7455743247944,0.,2.0698113262342));
#30154=CARTESIAN_POINT('Origin',(0.61342227326009,0.,2.11275013067528));
#30155=CARTESIAN_POINT('',(0.61342227326009,1.,2.11275013067528));
#30156=CARTESIAN_POINT('',(0.7455743247944,1.,2.0698113262342));
#30157=CARTESIAN_POINT('',(0.61342227326009,0.,2.11275013067528));
#30158=CARTESIAN_POINT('Ctrl Pts',(0.383122945602004,-1.,1.7075470150345));
#30159=CARTESIAN_POINT('Ctrl Pts',(0.383122945602004,1.,1.7075470150345));
#30160=CARTESIAN_POINT('Ctrl Pts',(0.384119047315541,-1.,1.71231062891958));
#30161=CARTESIAN_POINT('Ctrl Pts',(0.384119047315541,1.,1.71231062891958));
#30162=CARTESIAN_POINT('Ctrl Pts',(0.38607079032701,-1.,1.72162022246158));
#30163=CARTESIAN_POINT('Ctrl Pts',(0.38607079032701,1.,1.72162022246158));
#30164=CARTESIAN_POINT('Ctrl Pts',(0.388877023509191,-1.,1.7349317097561));
#30165=CARTESIAN_POINT('Ctrl Pts',(0.388877023509191,1.,1.7349317097561));
#30166=CARTESIAN_POINT('Ctrl Pts',(0.392375812294307,-1.,1.75137405313962));
#30167=CARTESIAN_POINT('Ctrl Pts',(0.392375812294307,1.,1.75137405313962));
#30168=CARTESIAN_POINT('Ctrl Pts',(0.39634619612042,-1.,1.7697556004756));
#30169=CARTESIAN_POINT('Ctrl Pts',(0.39634619612042,1.,1.7697556004756));
#30170=CARTESIAN_POINT('Ctrl Pts',(0.39991940378308,-1.,1.78598826347533));
#30171=CARTESIAN_POINT('Ctrl Pts',(0.39991940378308,1.,1.78598826347533));
#30172=CARTESIAN_POINT('Ctrl Pts',(0.403107976170441,-1.,1.80012077176221));
#30173=CARTESIAN_POINT('Ctrl Pts',(0.403107976170441,1.,1.80012077176221));
#30174=CARTESIAN_POINT('Ctrl Pts',(0.405933518411838,-1.,1.81223801813988));
#30175=CARTESIAN_POINT('Ctrl Pts',(0.405933518411838,1.,1.81223801813988));
#30176=CARTESIAN_POINT('Ctrl Pts',(0.408428948108533,-1.,1.8224702267854));
#30177=CARTESIAN_POINT('Ctrl Pts',(0.408428948108533,1.,1.8224702267854));
#30178=CARTESIAN_POINT('Ctrl Pts',(0.410641256301674,-1.,1.83100408895216));
#30179=CARTESIAN_POINT('Ctrl Pts',(0.410641256301674,1.,1.83100408895216));
#30180=CARTESIAN_POINT('Ctrl Pts',(0.412633125322161,-1.,1.83808953475839));
#30181=CARTESIAN_POINT('Ctrl Pts',(0.412633125322161,1.,1.83808953475839));
#30182=CARTESIAN_POINT('Ctrl Pts',(0.41448743825434,-1.,1.8440575707371));
#30183=CARTESIAN_POINT('Ctrl Pts',(0.41448743825434,1.,1.8440575707371));
#30184=CARTESIAN_POINT('Ctrl Pts',(0.416300022038864,-1.,1.84929312929882));
#30185=CARTESIAN_POINT('Ctrl Pts',(0.416300022038864,1.,1.84929312929882));
#30186=CARTESIAN_POINT('Ctrl Pts',(0.418164129143534,-1.,1.85417632856234));
#30187=CARTESIAN_POINT('Ctrl Pts',(0.418164129143534,1.,1.85417632856234));
#30188=CARTESIAN_POINT('Ctrl Pts',(0.420157287975619,-1.,1.85903281096686));
#30189=CARTESIAN_POINT('Ctrl Pts',(0.420157287975619,1.,1.85903281096686));
#30190=CARTESIAN_POINT('Ctrl Pts',(0.422327307418275,-1.,1.86408083334028));
#30191=CARTESIAN_POINT('Ctrl Pts',(0.422327307418275,1.,1.86408083334028));
#30192=CARTESIAN_POINT('Ctrl Pts',(0.424678177291358,-1.,1.86937803944323));
#30193=CARTESIAN_POINT('Ctrl Pts',(0.424678177291358,1.,1.86937803944323));
#30194=CARTESIAN_POINT('Ctrl Pts',(0.427183828519102,-1.,1.87486989291484));
#30195=CARTESIAN_POINT('Ctrl Pts',(0.427183828519102,1.,1.87486989291484));
#30196=CARTESIAN_POINT('Ctrl Pts',(0.429803062482344,-1.,1.88044229001832));
#30197=CARTESIAN_POINT('Ctrl Pts',(0.429803062482344,1.,1.88044229001832));
#30198=CARTESIAN_POINT('Ctrl Pts',(0.432493038548748,-1.,1.88596913666793));
#30199=CARTESIAN_POINT('Ctrl Pts',(0.432493038548748,1.,1.88596913666793));
#30200=CARTESIAN_POINT('Ctrl Pts',(0.435225660963383,-1.,1.89136993975504));
#30201=CARTESIAN_POINT('Ctrl Pts',(0.435225660963383,1.,1.89136993975504));
#30202=CARTESIAN_POINT('Ctrl Pts',(0.437995003948244,-1.,1.89663648956466));
#30203=CARTESIAN_POINT('Ctrl Pts',(0.437995003948244,1.,1.89663648956466));
#30204=CARTESIAN_POINT('Ctrl Pts',(0.440807833704038,-1.,1.90180124389086));
#30205=CARTESIAN_POINT('Ctrl Pts',(0.440807833704038,1.,1.90180124389086));
#30206=CARTESIAN_POINT('Ctrl Pts',(0.44367755684915,-1.,1.90691756144898));
#30207=CARTESIAN_POINT('Ctrl Pts',(0.44367755684915,1.,1.90691756144898));
#30208=CARTESIAN_POINT('Ctrl Pts',(0.446617343485711,-1.,1.9120369998112));
#30209=CARTESIAN_POINT('Ctrl Pts',(0.446617343485711,1.,1.9120369998112));
#30210=CARTESIAN_POINT('Ctrl Pts',(0.449632260106662,-1.,1.91718342555755));
#30211=CARTESIAN_POINT('Ctrl Pts',(0.449632260106662,1.,1.91718342555755));
#30212=CARTESIAN_POINT('Ctrl Pts',(0.452719478359432,-1.,1.92235380648502));
#30213=CARTESIAN_POINT('Ctrl Pts',(0.452719478359432,1.,1.92235380648502));
#30214=CARTESIAN_POINT('Ctrl Pts',(0.45587200517437,-1.,1.92753067150476));
#30215=CARTESIAN_POINT('Ctrl Pts',(0.45587200517437,1.,1.92753067150476));
#30216=CARTESIAN_POINT('Ctrl Pts',(0.459081234547926,-1.,1.93269066517934));
#30217=CARTESIAN_POINT('Ctrl Pts',(0.459081234547926,1.,1.93269066517934));
#30218=CARTESIAN_POINT('Ctrl Pts',(0.462340031009056,-1.,1.93781486640821));
#30219=CARTESIAN_POINT('Ctrl Pts',(0.462340031009056,1.,1.93781486640821));
#30220=CARTESIAN_POINT('Ctrl Pts',(0.46564546202603,-1.,1.9428979419619));
#30221=CARTESIAN_POINT('Ctrl Pts',(0.46564546202603,1.,1.9428979419619));
#30222=CARTESIAN_POINT('Ctrl Pts',(0.468997482913135,-1.,1.94794381136514));
#30223=CARTESIAN_POINT('Ctrl Pts',(0.468997482913135,1.,1.94794381136514));
#30224=CARTESIAN_POINT('Ctrl Pts',(0.472397672264072,-1.,1.95296148278133));
#30225=CARTESIAN_POINT('Ctrl Pts',(0.472397672264072,1.,1.95296148278133));
#30226=CARTESIAN_POINT('Ctrl Pts',(0.475848034683176,-1.,1.95796111148177));
#30227=CARTESIAN_POINT('Ctrl Pts',(0.475848034683176,1.,1.95796111148177));
#30228=CARTESIAN_POINT('Ctrl Pts',(0.479349583074855,-1.,1.96294933055943));
#30229=CARTESIAN_POINT('Ctrl Pts',(0.479349583074855,1.,1.96294933055943));
#30230=CARTESIAN_POINT('Ctrl Pts',(0.48290166212069,-1.,1.96792703422362));
#30231=CARTESIAN_POINT('Ctrl Pts',(0.48290166212069,1.,1.96792703422362));
#30232=CARTESIAN_POINT('Ctrl Pts',(0.486502692907658,-1.,1.97289186263272));
#30233=CARTESIAN_POINT('Ctrl Pts',(0.486502692907658,1.,1.97289186263272));
#30234=CARTESIAN_POINT('Ctrl Pts',(0.490150627860952,-1.,1.97783973019229));
#30235=CARTESIAN_POINT('Ctrl Pts',(0.490150627860952,1.,1.97783973019229));
#30236=CARTESIAN_POINT('Ctrl Pts',(0.493843476541494,-1.,1.98276658761821));
#30237=CARTESIAN_POINT('Ctrl Pts',(0.493843476541494,1.,1.98276658761821));
#30238=CARTESIAN_POINT('Ctrl Pts',(0.497579909545574,-1.,1.98767044752932));
#30239=CARTESIAN_POINT('Ctrl Pts',(0.497579909545574,1.,1.98767044752932));
#30240=CARTESIAN_POINT('Ctrl Pts',(0.501359287727146,-1.,1.99255149126155));
#30241=CARTESIAN_POINT('Ctrl Pts',(0.501359287727146,1.,1.99255149126155));
#30242=CARTESIAN_POINT('Ctrl Pts',(0.505181361323026,-1.,1.99741107463572));
#30243=CARTESIAN_POINT('Ctrl Pts',(0.505181361323026,1.,1.99741107463572));
#30244=CARTESIAN_POINT('Ctrl Pts',(0.509046069886157,-1.,2.00225107134734));
#30245=CARTESIAN_POINT('Ctrl Pts',(0.509046069886157,1.,2.00225107134734));
#30246=CARTESIAN_POINT('Ctrl Pts',(0.512953306961792,-1.,2.00707309946949));
#30247=CARTESIAN_POINT('Ctrl Pts',(0.512953306961792,1.,2.00707309946949));
#30248=CARTESIAN_POINT('Ctrl Pts',(0.516902681728687,-1.,2.01187773939242));
#30249=CARTESIAN_POINT('Ctrl Pts',(0.516902681728687,1.,2.01187773939242));
#30250=CARTESIAN_POINT('Ctrl Pts',(0.52089359039937,-1.,2.01666477917286));
#30251=CARTESIAN_POINT('Ctrl Pts',(0.52089359039937,1.,2.01666477917286));
#30252=CARTESIAN_POINT('Ctrl Pts',(0.524925318333476,-1.,2.02143356304698));
#30253=CARTESIAN_POINT('Ctrl Pts',(0.524925318333476,1.,2.02143356304698));
#30254=CARTESIAN_POINT('Ctrl Pts',(0.528997127241914,-1.,2.0261832908329));
#30255=CARTESIAN_POINT('Ctrl Pts',(0.528997127241914,1.,2.0261832908329));
#30256=CARTESIAN_POINT('Ctrl Pts',(0.533108355132976,-1.,2.03091336214426));
#30257=CARTESIAN_POINT('Ctrl Pts',(0.533108355132976,1.,2.03091336214426));
#30258=CARTESIAN_POINT('Ctrl Pts',(0.537258489833262,-1.,2.03562362954037));
#30259=CARTESIAN_POINT('Ctrl Pts',(0.537258489833262,1.,2.03562362954037));
#30260=CARTESIAN_POINT('Ctrl Pts',(0.541447120615659,-1.,2.04031422690527));
#30261=CARTESIAN_POINT('Ctrl Pts',(0.541447120615659,1.,2.04031422690527));
#30262=CARTESIAN_POINT('Ctrl Pts',(0.54567390381743,-1.,2.04498544714588));
#30263=CARTESIAN_POINT('Ctrl Pts',(0.54567390381743,1.,2.04498544714588));
#30264=CARTESIAN_POINT('Ctrl Pts',(0.549938525150295,-1.,2.04963761077958));
#30265=CARTESIAN_POINT('Ctrl Pts',(0.549938525150295,1.,2.04963761077958));
#30266=CARTESIAN_POINT('Ctrl Pts',(0.554240657463906,-1.,2.05427091604413));
#30267=CARTESIAN_POINT('Ctrl Pts',(0.554240657463906,1.,2.05427091604413));
#30268=CARTESIAN_POINT('Ctrl Pts',(0.558579940185151,-1.,2.05888537756462));
#30269=CARTESIAN_POINT('Ctrl Pts',(0.558579940185151,1.,2.05888537756462));
#30270=CARTESIAN_POINT('Ctrl Pts',(0.562955993082261,-1.,2.06348090160589));
#30271=CARTESIAN_POINT('Ctrl Pts',(0.562955993082261,1.,2.06348090160589));
#30272=CARTESIAN_POINT('Ctrl Pts',(0.567368421181087,-1.,2.06805732997334));
#30273=CARTESIAN_POINT('Ctrl Pts',(0.567368421181087,1.,2.06805732997334));
#30274=CARTESIAN_POINT('Ctrl Pts',(0.571816823242602,-1.,2.07261449292824));
#30275=CARTESIAN_POINT('Ctrl Pts',(0.571816823242602,1.,2.07261449292824));
#30276=CARTESIAN_POINT('Ctrl Pts',(0.576300797416844,-1.,2.07715226767559));
#30277=CARTESIAN_POINT('Ctrl Pts',(0.576300797416844,1.,2.07715226767559));
#30278=CARTESIAN_POINT('Ctrl Pts',(0.580819952108063,-1.,2.08167059018418));
#30279=CARTESIAN_POINT('Ctrl Pts',(0.580819952108063,1.,2.08167059018418));
#30280=CARTESIAN_POINT('Ctrl Pts',(0.585373918991617,-1.,2.08616943727951));
#30281=CARTESIAN_POINT('Ctrl Pts',(0.585373918991617,1.,2.08616943727951));
#30282=CARTESIAN_POINT('Ctrl Pts',(0.589962365403406,-1.,2.09064881812129));
#30283=CARTESIAN_POINT('Ctrl Pts',(0.589962365403406,1.,2.09064881812129));
#30284=CARTESIAN_POINT('Ctrl Pts',(0.594585006052162,-1.,2.0951087622027));
#30285=CARTESIAN_POINT('Ctrl Pts',(0.594585006052162,1.,2.0951087622027));
#30286=CARTESIAN_POINT('Ctrl Pts',(0.599241616420533,-1.,2.0995493086477));
#30287=CARTESIAN_POINT('Ctrl Pts',(0.599241616420533,1.,2.0995493086477));
#30288=CARTESIAN_POINT('Ctrl Pts',(0.60393203073603,-1.,2.10397049886949));
#30289=CARTESIAN_POINT('Ctrl Pts',(0.60393203073603,1.,2.10397049886949));
#30290=CARTESIAN_POINT('Ctrl Pts',(0.607711315454876,-1.,2.1074919961518));
#30291=CARTESIAN_POINT('Ctrl Pts',(0.607711315454876,1.,2.1074919961518));
#30292=CARTESIAN_POINT('Ctrl Pts',(0.610560911689898,-1.,2.11012443807238));
#30293=CARTESIAN_POINT('Ctrl Pts',(0.610560911689898,1.,2.11012443807238));
#30294=CARTESIAN_POINT('Ctrl Pts',(0.6124673655618,-1.,2.11187554259986));
#30295=CARTESIAN_POINT('Ctrl Pts',(0.6124673655618,1.,2.11187554259986));
#30296=CARTESIAN_POINT('Ctrl Pts',(0.61342227326009,-1.,2.11275013067528));
#30297=CARTESIAN_POINT('Ctrl Pts',(0.61342227326009,1.,2.11275013067528));
#30298=CARTESIAN_POINT('',(0.383122945602004,1.,1.7075470150345));
#30299=CARTESIAN_POINT('Ctrl Pts',(0.383122945602004,1.,1.7075470150345));
#30300=CARTESIAN_POINT('Ctrl Pts',(0.384119047315541,1.,1.71231062891958));
#30301=CARTESIAN_POINT('Ctrl Pts',(0.38607079032701,1.,1.72162022246158));
#30302=CARTESIAN_POINT('Ctrl Pts',(0.388877023509191,1.,1.7349317097561));
#30303=CARTESIAN_POINT('Ctrl Pts',(0.392375812294307,1.,1.75137405313962));
#30304=CARTESIAN_POINT('Ctrl Pts',(0.39634619612042,1.,1.7697556004756));
#30305=CARTESIAN_POINT('Ctrl Pts',(0.39991940378308,1.,1.78598826347533));
#30306=CARTESIAN_POINT('Ctrl Pts',(0.403107976170441,1.,1.80012077176221));
#30307=CARTESIAN_POINT('Ctrl Pts',(0.405933518411838,1.,1.81223801813988));
#30308=CARTESIAN_POINT('Ctrl Pts',(0.408428948108533,1.,1.8224702267854));
#30309=CARTESIAN_POINT('Ctrl Pts',(0.410641256301674,1.,1.83100408895216));
#30310=CARTESIAN_POINT('Ctrl Pts',(0.412633125322161,1.,1.83808953475839));
#30311=CARTESIAN_POINT('Ctrl Pts',(0.41448743825434,1.,1.8440575707371));
#30312=CARTESIAN_POINT('Ctrl Pts',(0.416300022038864,1.,1.84929312929882));
#30313=CARTESIAN_POINT('Ctrl Pts',(0.418164129143534,1.,1.85417632856234));
#30314=CARTESIAN_POINT('Ctrl Pts',(0.420157287975619,1.,1.85903281096686));
#30315=CARTESIAN_POINT('Ctrl Pts',(0.422327307418275,1.,1.86408083334028));
#30316=CARTESIAN_POINT('Ctrl Pts',(0.424678177291358,1.,1.86937803944323));
#30317=CARTESIAN_POINT('Ctrl Pts',(0.427183828519102,1.,1.87486989291484));
#30318=CARTESIAN_POINT('Ctrl Pts',(0.429803062482344,1.,1.88044229001832));
#30319=CARTESIAN_POINT('Ctrl Pts',(0.432493038548748,1.,1.88596913666793));
#30320=CARTESIAN_POINT('Ctrl Pts',(0.435225660963383,1.,1.89136993975504));
#30321=CARTESIAN_POINT('Ctrl Pts',(0.437995003948244,1.,1.89663648956466));
#30322=CARTESIAN_POINT('Ctrl Pts',(0.440807833704038,1.,1.90180124389086));
#30323=CARTESIAN_POINT('Ctrl Pts',(0.44367755684915,1.,1.90691756144898));
#30324=CARTESIAN_POINT('Ctrl Pts',(0.446617343485711,1.,1.9120369998112));
#30325=CARTESIAN_POINT('Ctrl Pts',(0.449632260106662,1.,1.91718342555755));
#30326=CARTESIAN_POINT('Ctrl Pts',(0.452719478359432,1.,1.92235380648502));
#30327=CARTESIAN_POINT('Ctrl Pts',(0.45587200517437,1.,1.92753067150476));
#30328=CARTESIAN_POINT('Ctrl Pts',(0.459081234547926,1.,1.93269066517934));
#30329=CARTESIAN_POINT('Ctrl Pts',(0.462340031009056,1.,1.93781486640821));
#30330=CARTESIAN_POINT('Ctrl Pts',(0.46564546202603,1.,1.9428979419619));
#30331=CARTESIAN_POINT('Ctrl Pts',(0.468997482913135,1.,1.94794381136514));
#30332=CARTESIAN_POINT('Ctrl Pts',(0.472397672264072,1.,1.95296148278133));
#30333=CARTESIAN_POINT('Ctrl Pts',(0.475848034683176,1.,1.95796111148177));
#30334=CARTESIAN_POINT('Ctrl Pts',(0.479349583074855,1.,1.96294933055943));
#30335=CARTESIAN_POINT('Ctrl Pts',(0.48290166212069,1.,1.96792703422362));
#30336=CARTESIAN_POINT('Ctrl Pts',(0.486502692907658,1.,1.97289186263272));
#30337=CARTESIAN_POINT('Ctrl Pts',(0.490150627860952,1.,1.97783973019229));
#30338=CARTESIAN_POINT('Ctrl Pts',(0.493843476541494,1.,1.98276658761821));
#30339=CARTESIAN_POINT('Ctrl Pts',(0.497579909545574,1.,1.98767044752932));
#30340=CARTESIAN_POINT('Ctrl Pts',(0.501359287727146,1.,1.99255149126155));
#30341=CARTESIAN_POINT('Ctrl Pts',(0.505181361323026,1.,1.99741107463572));
#30342=CARTESIAN_POINT('Ctrl Pts',(0.509046069886157,1.,2.00225107134734));
#30343=CARTESIAN_POINT('Ctrl Pts',(0.512953306961792,1.,2.00707309946949));
#30344=CARTESIAN_POINT('Ctrl Pts',(0.516902681728687,1.,2.01187773939242));
#30345=CARTESIAN_POINT('Ctrl Pts',(0.52089359039937,1.,2.01666477917286));
#30346=CARTESIAN_POINT('Ctrl Pts',(0.524925318333476,1.,2.02143356304698));
#30347=CARTESIAN_POINT('Ctrl Pts',(0.528997127241914,1.,2.0261832908329));
#30348=CARTESIAN_POINT('Ctrl Pts',(0.533108355132976,1.,2.03091336214426));
#30349=CARTESIAN_POINT('Ctrl Pts',(0.537258489833262,1.,2.03562362954037));
#30350=CARTESIAN_POINT('Ctrl Pts',(0.541447120615659,1.,2.04031422690527));
#30351=CARTESIAN_POINT('Ctrl Pts',(0.54567390381743,1.,2.04498544714588));
#30352=CARTESIAN_POINT('Ctrl Pts',(0.549938525150295,1.,2.04963761077958));
#30353=CARTESIAN_POINT('Ctrl Pts',(0.554240657463906,1.,2.05427091604413));
#30354=CARTESIAN_POINT('Ctrl Pts',(0.558579940185151,1.,2.05888537756462));
#30355=CARTESIAN_POINT('Ctrl Pts',(0.562955993082261,1.,2.06348090160589));
#30356=CARTESIAN_POINT('Ctrl Pts',(0.567368421181087,1.,2.06805732997334));
#30357=CARTESIAN_POINT('Ctrl Pts',(0.571816823242602,1.,2.07261449292824));
#30358=CARTESIAN_POINT('Ctrl Pts',(0.576300797416844,1.,2.07715226767559));
#30359=CARTESIAN_POINT('Ctrl Pts',(0.580819952108063,1.,2.08167059018418));
#30360=CARTESIAN_POINT('Ctrl Pts',(0.585373918991617,1.,2.08616943727951));
#30361=CARTESIAN_POINT('Ctrl Pts',(0.589962365403406,1.,2.09064881812129));
#30362=CARTESIAN_POINT('Ctrl Pts',(0.594585006052162,1.,2.0951087622027));
#30363=CARTESIAN_POINT('Ctrl Pts',(0.599241616420533,1.,2.0995493086477));
#30364=CARTESIAN_POINT('Ctrl Pts',(0.60393203073603,1.,2.10397049886949));
#30365=CARTESIAN_POINT('Ctrl Pts',(0.607711315454876,1.,2.1074919961518));
#30366=CARTESIAN_POINT('Ctrl Pts',(0.610560911689898,1.,2.11012443807238));
#30367=CARTESIAN_POINT('Ctrl Pts',(0.6124673655618,1.,2.11187554259986));
#30368=CARTESIAN_POINT('Ctrl Pts',(0.61342227326009,1.,2.11275013067528));
#30369=CARTESIAN_POINT('',(0.383122945602003,0.,1.7075470150345));
#30370=CARTESIAN_POINT('Origin',(0.,0.,0.));
#30371=CARTESIAN_POINT('',(0.163289472382896,1.,1.74236521665491));
#30372=CARTESIAN_POINT('Origin',(0.,1.,0.));
#30373=CARTESIAN_POINT('',(0.163289472382896,0.,1.74236521665491));
#30374=CARTESIAN_POINT('Ctrl Pts',(0.0694764450219578,-1.,2.19890268624765));
#30375=CARTESIAN_POINT('Ctrl Pts',(0.0694764450219578,1.,2.19890268624765));
#30376=CARTESIAN_POINT('Ctrl Pts',(0.0701143536325487,-1.,2.19777582085423));
#30377=CARTESIAN_POINT('Ctrl Pts',(0.0701143536325487,1.,2.19777582085423));
#30378=CARTESIAN_POINT('Ctrl Pts',(0.0713863779526151,-1.,2.19552129484002));
#30379=CARTESIAN_POINT('Ctrl Pts',(0.0713863779526151,1.,2.19552129484002));
#30380=CARTESIAN_POINT('Ctrl Pts',(0.0732830357306722,-1.,2.19213712013662));
#30381=CARTESIAN_POINT('Ctrl Pts',(0.0732830357306722,1.,2.19213712013662));
#30382=CARTESIAN_POINT('Ctrl Pts',(0.0757891465836145,-1.,2.1876201139953));
#30383=CARTESIAN_POINT('Ctrl Pts',(0.0757891465836145,1.,2.1876201139953));
#30384=CARTESIAN_POINT('Ctrl Pts',(0.078883772768524,-1.,2.18196589448887));
#30385=CARTESIAN_POINT('Ctrl Pts',(0.078883772768524,1.,2.18196589448887));
#30386=CARTESIAN_POINT('Ctrl Pts',(0.0819402680872763,-1.,2.176303712113));
#30387=CARTESIAN_POINT('Ctrl Pts',(0.0819402680872763,1.,2.176303712113));
#30388=CARTESIAN_POINT('Ctrl Pts',(0.084958462083537,-1.,2.17063357870952));
#30389=CARTESIAN_POINT('Ctrl Pts',(0.084958462083537,1.,2.17063357870952));
#30390=CARTESIAN_POINT('Ctrl Pts',(0.087938129138692,-1.,2.16495552645014));
#30391=CARTESIAN_POINT('Ctrl Pts',(0.087938129138692,1.,2.16495552645014));
#30392=CARTESIAN_POINT('Ctrl Pts',(0.0908789888107263,-1.,2.15926961544516));
#30393=CARTESIAN_POINT('Ctrl Pts',(0.0908789888107263,1.,2.15926961544516));
#30394=CARTESIAN_POINT('Ctrl Pts',(0.0937807218867641,-1.,2.1535759397817));
#30395=CARTESIAN_POINT('Ctrl Pts',(0.0937807218867641,1.,2.1535759397817));
#30396=CARTESIAN_POINT('Ctrl Pts',(0.0966429852305456,-1.,2.14787463531795));
#30397=CARTESIAN_POINT('Ctrl Pts',(0.0966429852305456,1.,2.14787463531795));
#30398=CARTESIAN_POINT('Ctrl Pts',(0.0994654261990913,-1.,2.14216588396025));
#30399=CARTESIAN_POINT('Ctrl Pts',(0.0994654261990913,1.,2.14216588396025));
#30400=CARTESIAN_POINT('Ctrl Pts',(0.1022477005561,-1.,2.13644992667165));
#30401=CARTESIAN_POINT('Ctrl Pts',(0.1022477005561,1.,2.13644992667165));
#30402=CARTESIAN_POINT('Ctrl Pts',(0.104989479152739,-1.,2.13072704887293));
#30403=CARTESIAN_POINT('Ctrl Pts',(0.104989479152739,1.,2.13072704887293));
#30404=CARTESIAN_POINT('Ctrl Pts',(0.10769043523109,-1.,2.12499752307));
#30405=CARTESIAN_POINT('Ctrl Pts',(0.10769043523109,1.,2.12499752307));
#30406=CARTESIAN_POINT('Ctrl Pts',(0.110350236135025,-1.,2.11926155590865));
#30407=CARTESIAN_POINT('Ctrl Pts',(0.110350236135025,1.,2.11926155590865));
#30408=CARTESIAN_POINT('Ctrl Pts',(0.112968534419737,-1.,2.11351924490306));
#30409=CARTESIAN_POINT('Ctrl Pts',(0.112968534419737,1.,2.11351924490306));
#30410=CARTESIAN_POINT('Ctrl Pts',(0.115544957687926,-1.,2.10777050261309));
#30411=CARTESIAN_POINT('Ctrl Pts',(0.115544957687926,1.,2.10777050261309));
#30412=CARTESIAN_POINT('Ctrl Pts',(0.118079107988355,-1.,2.102015121329));
#30413=CARTESIAN_POINT('Ctrl Pts',(0.118079107988355,1.,2.102015121329));
#30414=CARTESIAN_POINT('Ctrl Pts',(0.120570567965122,-1.,2.0962529286773));
#30415=CARTESIAN_POINT('Ctrl Pts',(0.120570567965122,1.,2.0962529286773));
#30416=CARTESIAN_POINT('Ctrl Pts',(0.123018905621083,-1.,2.09048392424825));
#30417=CARTESIAN_POINT('Ctrl Pts',(0.123018905621083,1.,2.09048392424825));
#30418=CARTESIAN_POINT('Ctrl Pts',(0.125423679412061,-1.,2.08470840653643));
#30419=CARTESIAN_POINT('Ctrl Pts',(0.125423679412061,1.,2.08470840653643));
#30420=CARTESIAN_POINT('Ctrl Pts',(0.12778444527612,-1.,2.07892715110987));
#30421=CARTESIAN_POINT('Ctrl Pts',(0.12778444527612,1.,2.07892715110987));
#30422=CARTESIAN_POINT('Ctrl Pts',(0.130100748328403,-1.,2.07314114713063));
#30423=CARTESIAN_POINT('Ctrl Pts',(0.130100748328403,1.,2.07314114713063));
#30424=CARTESIAN_POINT('Ctrl Pts',(0.13237211154771,-1.,2.06735123910326));
#30425=CARTESIAN_POINT('Ctrl Pts',(0.13237211154771,1.,2.06735123910326));
#30426=CARTESIAN_POINT('Ctrl Pts',(0.134598026192106,-1.,2.06155781517842));
#30427=CARTESIAN_POINT('Ctrl Pts',(0.134598026192106,1.,2.06155781517842));
#30428=CARTESIAN_POINT('Ctrl Pts',(0.136777941218043,-1.,2.05576044414264));
#30429=CARTESIAN_POINT('Ctrl Pts',(0.136777941218043,1.,2.05576044414264));
#30430=CARTESIAN_POINT('Ctrl Pts',(0.138911255368966,-1.,2.04995762001328));
#30431=CARTESIAN_POINT('Ctrl Pts',(0.138911255368966,1.,2.04995762001328));
#30432=CARTESIAN_POINT('Ctrl Pts',(0.140997332152546,-1.,2.04414757947916));
#30433=CARTESIAN_POINT('Ctrl Pts',(0.140997332152546,1.,2.04414757947916));
#30434=CARTESIAN_POINT('Ctrl Pts',(0.143035515058208,-1.,2.03832911025912));
#30435=CARTESIAN_POINT('Ctrl Pts',(0.143035515058208,1.,2.03832911025912));
#30436=CARTESIAN_POINT('Ctrl Pts',(0.145025140186057,-1.,2.03250223739942));
#30437=CARTESIAN_POINT('Ctrl Pts',(0.145025140186057,1.,2.03250223739942));
#30438=CARTESIAN_POINT('Ctrl Pts',(0.146965557332583,-1.,2.02666926182017));
#30439=CARTESIAN_POINT('Ctrl Pts',(0.146965557332583,1.,2.02666926182017));
#30440=CARTESIAN_POINT('Ctrl Pts',(0.148856124775337,-1.,2.02083464969894));
#30441=CARTESIAN_POINT('Ctrl Pts',(0.148856124775337,1.,2.02083464969894));
#30442=CARTESIAN_POINT('Ctrl Pts',(0.150696157673078,-1.,2.01500291940238));
#30443=CARTESIAN_POINT('Ctrl Pts',(0.150696157673078,1.,2.01500291940238));
#30444=CARTESIAN_POINT('Ctrl Pts',(0.152484883621449,-1.,2.00917680318424));
#30445=CARTESIAN_POINT('Ctrl Pts',(0.152484883621449,1.,2.00917680318424));
#30446=CARTESIAN_POINT('Ctrl Pts',(0.154221403049722,-1.,2.00335565310543));
#30447=CARTESIAN_POINT('Ctrl Pts',(0.154221403049722,1.,2.00335565310543));
#30448=CARTESIAN_POINT('Ctrl Pts',(0.155904629548783,-1.,1.99753284771497));
#30449=CARTESIAN_POINT('Ctrl Pts',(0.155904629548783,1.,1.99753284771497));
#30450=CARTESIAN_POINT('Ctrl Pts',(0.157533331459227,-1.,1.99169810931908));
#30451=CARTESIAN_POINT('Ctrl Pts',(0.157533331459227,1.,1.99169810931908));
#30452=CARTESIAN_POINT('Ctrl Pts',(0.159106226437299,-1.,1.98584238283292));
#30453=CARTESIAN_POINT('Ctrl Pts',(0.159106226437299,1.,1.98584238283292));
#30454=CARTESIAN_POINT('Ctrl Pts',(0.160622060784611,-1.,1.97996195437559));
#30455=CARTESIAN_POINT('Ctrl Pts',(0.160622060784611,1.,1.97996195437559));
#30456=CARTESIAN_POINT('Ctrl Pts',(0.162079693556288,-1.,1.97406280235188));
#30457=CARTESIAN_POINT('Ctrl Pts',(0.162079693556288,1.,1.97406280235188));
#30458=CARTESIAN_POINT('Ctrl Pts',(0.163478185457734,-1.,1.96816512677967));
#30459=CARTESIAN_POINT('Ctrl Pts',(0.163478185457734,1.,1.96816512677967));
#30460=CARTESIAN_POINT('Ctrl Pts',(0.164816568920269,-1.,1.96229379940136));
#30461=CARTESIAN_POINT('Ctrl Pts',(0.164816568920269,1.,1.96229379940136));
#30462=CARTESIAN_POINT('Ctrl Pts',(0.166093592002812,-1.,1.9564675971873));
#30463=CARTESIAN_POINT('Ctrl Pts',(0.166093592002812,1.,1.9564675971873));
#30464=CARTESIAN_POINT('Ctrl Pts',(0.167307501784475,-1.,1.95069027794294));
#30465=CARTESIAN_POINT('Ctrl Pts',(0.167307501784475,1.,1.95069027794294));
#30466=CARTESIAN_POINT('Ctrl Pts',(0.168455741607556,-1.,1.94493757756931));
#30467=CARTESIAN_POINT('Ctrl Pts',(0.168455741607556,1.,1.94493757756931));
#30468=CARTESIAN_POINT('Ctrl Pts',(0.16953490481749,-1.,1.93915639211581));
#30469=CARTESIAN_POINT('Ctrl Pts',(0.16953490481749,1.,1.93915639211581));
#30470=CARTESIAN_POINT('Ctrl Pts',(0.170541253116201,-1.,1.93329183155539));
#30471=CARTESIAN_POINT('Ctrl Pts',(0.170541253116201,1.,1.93329183155539));
#30472=CARTESIAN_POINT('Ctrl Pts',(0.171471191532988,-1.,1.92731093582036));
#30473=CARTESIAN_POINT('Ctrl Pts',(0.171471191532988,1.,1.92731093582036));
#30474=CARTESIAN_POINT('Ctrl Pts',(0.172321621259513,-1.,1.9212233439798));
#30475=CARTESIAN_POINT('Ctrl Pts',(0.172321621259513,1.,1.9212233439798));
#30476=CARTESIAN_POINT('Ctrl Pts',(0.173090695383496,-1.,1.91511429159527));
#30477=CARTESIAN_POINT('Ctrl Pts',(0.173090695383496,1.,1.91511429159527));
#30478=CARTESIAN_POINT('Ctrl Pts',(0.173776635257816,-1.,1.90911693975267));
#30479=CARTESIAN_POINT('Ctrl Pts',(0.173776635257816,1.,1.90911693975267));
#30480=CARTESIAN_POINT('Ctrl Pts',(0.174375518661085,-1.,1.90335253862834));
#30481=CARTESIAN_POINT('Ctrl Pts',(0.174375518661085,1.,1.90335253862834));
#30482=CARTESIAN_POINT('Ctrl Pts',(0.174879405091263,-1.,1.89788101117132));
#30483=CARTESIAN_POINT('Ctrl Pts',(0.174879405091263,1.,1.89788101117132));
#30484=CARTESIAN_POINT('Ctrl Pts',(0.175274276190844,-1.,1.892646301985));
#30485=CARTESIAN_POINT('Ctrl Pts',(0.175274276190844,1.,1.892646301985));
#30486=CARTESIAN_POINT('Ctrl Pts',(0.175538155840648,-1.,1.88742606273259));
#30487=CARTESIAN_POINT('Ctrl Pts',(0.175538155840648,1.,1.88742606273259));
#30488=CARTESIAN_POINT('Ctrl Pts',(0.175644148889698,-1.,1.88188663145367));
#30489=CARTESIAN_POINT('Ctrl Pts',(0.175644148889698,1.,1.88188663145367));
#30490=CARTESIAN_POINT('Ctrl Pts',(0.175563480746485,-1.,1.87563767773588));
#30491=CARTESIAN_POINT('Ctrl Pts',(0.175563480746485,1.,1.87563767773588));
#30492=CARTESIAN_POINT('Ctrl Pts',(0.175268337590757,-1.,1.86828349694799));
#30493=CARTESIAN_POINT('Ctrl Pts',(0.175268337590757,1.,1.86828349694799));
#30494=CARTESIAN_POINT('Ctrl Pts',(0.17473525927603,-1.,1.85948367088837));
#30495=CARTESIAN_POINT('Ctrl Pts',(0.17473525927603,1.,1.85948367088837));
#30496=CARTESIAN_POINT('Ctrl Pts',(0.173946627587731,-1.,1.8489811319852));
#30497=CARTESIAN_POINT('Ctrl Pts',(0.173946627587731,1.,1.8489811319852));
#30498=CARTESIAN_POINT('Ctrl Pts',(0.1728894428919,-1.,1.83658380527692));
#30499=CARTESIAN_POINT('Ctrl Pts',(0.1728894428919,1.,1.83658380527692));
#30500=CARTESIAN_POINT('Ctrl Pts',(0.171554770204119,-1.,1.82215766811545));
#30501=CARTESIAN_POINT('Ctrl Pts',(0.171554770204119,1.,1.82215766811545));
#30502=CARTESIAN_POINT('Ctrl Pts',(0.169936923904608,-1.,1.80561530629706));
#30503=CARTESIAN_POINT('Ctrl Pts',(0.169936923904608,1.,1.80561530629706));
#30504=CARTESIAN_POINT('Ctrl Pts',(0.168032772805197,-1.,1.7869064998507));
#30505=CARTESIAN_POINT('Ctrl Pts',(0.168032772805197,1.,1.7869064998507));
#30506=CARTESIAN_POINT('Ctrl Pts',(0.1662793551464,-1.,1.77018771684844));
#30507=CARTESIAN_POINT('Ctrl Pts',(0.1662793551464,1.,1.77018771684844));
#30508=CARTESIAN_POINT('Ctrl Pts',(0.164834765707158,-1.,1.75666056638427));
#30509=CARTESIAN_POINT('Ctrl Pts',(0.164834765707158,1.,1.75666056638427));
#30510=CARTESIAN_POINT('Ctrl Pts',(0.163814161002002,-1.,1.7472034950333));
#30511=CARTESIAN_POINT('Ctrl Pts',(0.163814161002002,1.,1.7472034950333));
#30512=CARTESIAN_POINT('Ctrl Pts',(0.163289472382896,-1.,1.74236521665491));
#30513=CARTESIAN_POINT('Ctrl Pts',(0.163289472382896,1.,1.74236521665491));
#30514=CARTESIAN_POINT('',(0.0694764450219578,1.,2.19890268624765));
#30515=CARTESIAN_POINT('Ctrl Pts',(0.0694764450219578,1.,2.19890268624765));
#30516=CARTESIAN_POINT('Ctrl Pts',(0.0701143536325487,1.,2.19777582085423));
#30517=CARTESIAN_POINT('Ctrl Pts',(0.0713863779526151,1.,2.19552129484002));
#30518=CARTESIAN_POINT('Ctrl Pts',(0.0732830357306722,1.,2.19213712013662));
#30519=CARTESIAN_POINT('Ctrl Pts',(0.0757891465836145,1.,2.1876201139953));
#30520=CARTESIAN_POINT('Ctrl Pts',(0.078883772768524,1.,2.18196589448887));
#30521=CARTESIAN_POINT('Ctrl Pts',(0.0819402680872763,1.,2.176303712113));
#30522=CARTESIAN_POINT('Ctrl Pts',(0.084958462083537,1.,2.17063357870952));
#30523=CARTESIAN_POINT('Ctrl Pts',(0.087938129138692,1.,2.16495552645014));
#30524=CARTESIAN_POINT('Ctrl Pts',(0.0908789888107263,1.,2.15926961544516));
#30525=CARTESIAN_POINT('Ctrl Pts',(0.0937807218867641,1.,2.1535759397817));
#30526=CARTESIAN_POINT('Ctrl Pts',(0.0966429852305456,1.,2.14787463531795));
#30527=CARTESIAN_POINT('Ctrl Pts',(0.0994654261990913,1.,2.14216588396025));
#30528=CARTESIAN_POINT('Ctrl Pts',(0.1022477005561,1.,2.13644992667165));
#30529=CARTESIAN_POINT('Ctrl Pts',(0.104989479152739,1.,2.13072704887293));
#30530=CARTESIAN_POINT('Ctrl Pts',(0.10769043523109,1.,2.12499752307));
#30531=CARTESIAN_POINT('Ctrl Pts',(0.110350236135025,1.,2.11926155590865));
#30532=CARTESIAN_POINT('Ctrl Pts',(0.112968534419737,1.,2.11351924490306));
#30533=CARTESIAN_POINT('Ctrl Pts',(0.115544957687926,1.,2.10777050261309));
#30534=CARTESIAN_POINT('Ctrl Pts',(0.118079107988355,1.,2.102015121329));
#30535=CARTESIAN_POINT('Ctrl Pts',(0.120570567965122,1.,2.0962529286773));
#30536=CARTESIAN_POINT('Ctrl Pts',(0.123018905621083,1.,2.09048392424825));
#30537=CARTESIAN_POINT('Ctrl Pts',(0.125423679412061,1.,2.08470840653643));
#30538=CARTESIAN_POINT('Ctrl Pts',(0.12778444527612,1.,2.07892715110987));
#30539=CARTESIAN_POINT('Ctrl Pts',(0.130100748328403,1.,2.07314114713063));
#30540=CARTESIAN_POINT('Ctrl Pts',(0.13237211154771,1.,2.06735123910326));
#30541=CARTESIAN_POINT('Ctrl Pts',(0.134598026192106,1.,2.06155781517842));
#30542=CARTESIAN_POINT('Ctrl Pts',(0.136777941218043,1.,2.05576044414264));
#30543=CARTESIAN_POINT('Ctrl Pts',(0.138911255368966,1.,2.04995762001328));
#30544=CARTESIAN_POINT('Ctrl Pts',(0.140997332152546,1.,2.04414757947916));
#30545=CARTESIAN_POINT('Ctrl Pts',(0.143035515058208,1.,2.03832911025912));
#30546=CARTESIAN_POINT('Ctrl Pts',(0.145025140186057,1.,2.03250223739942));
#30547=CARTESIAN_POINT('Ctrl Pts',(0.146965557332583,1.,2.02666926182017));
#30548=CARTESIAN_POINT('Ctrl Pts',(0.148856124775337,1.,2.02083464969894));
#30549=CARTESIAN_POINT('Ctrl Pts',(0.150696157673078,1.,2.01500291940238));
#30550=CARTESIAN_POINT('Ctrl Pts',(0.152484883621449,1.,2.00917680318424));
#30551=CARTESIAN_POINT('Ctrl Pts',(0.154221403049722,1.,2.00335565310543));
#30552=CARTESIAN_POINT('Ctrl Pts',(0.155904629548783,1.,1.99753284771497));
#30553=CARTESIAN_POINT('Ctrl Pts',(0.157533331459227,1.,1.99169810931908));
#30554=CARTESIAN_POINT('Ctrl Pts',(0.159106226437299,1.,1.98584238283292));
#30555=CARTESIAN_POINT('Ctrl Pts',(0.160622060784611,1.,1.97996195437559));
#30556=CARTESIAN_POINT('Ctrl Pts',(0.162079693556288,1.,1.97406280235188));
#30557=CARTESIAN_POINT('Ctrl Pts',(0.163478185457734,1.,1.96816512677967));
#30558=CARTESIAN_POINT('Ctrl Pts',(0.164816568920269,1.,1.96229379940136));
#30559=CARTESIAN_POINT('Ctrl Pts',(0.166093592002812,1.,1.9564675971873));
#30560=CARTESIAN_POINT('Ctrl Pts',(0.167307501784475,1.,1.95069027794294));
#30561=CARTESIAN_POINT('Ctrl Pts',(0.168455741607556,1.,1.94493757756931));
#30562=CARTESIAN_POINT('Ctrl Pts',(0.16953490481749,1.,1.93915639211581));
#30563=CARTESIAN_POINT('Ctrl Pts',(0.170541253116201,1.,1.93329183155539));
#30564=CARTESIAN_POINT('Ctrl Pts',(0.171471191532988,1.,1.92731093582036));
#30565=CARTESIAN_POINT('Ctrl Pts',(0.172321621259513,1.,1.9212233439798));
#30566=CARTESIAN_POINT('Ctrl Pts',(0.173090695383496,1.,1.91511429159527));
#30567=CARTESIAN_POINT('Ctrl Pts',(0.173776635257816,1.,1.90911693975267));
#30568=CARTESIAN_POINT('Ctrl Pts',(0.174375518661085,1.,1.90335253862834));
#30569=CARTESIAN_POINT('Ctrl Pts',(0.174879405091263,1.,1.89788101117132));
#30570=CARTESIAN_POINT('Ctrl Pts',(0.175274276190844,1.,1.892646301985));
#30571=CARTESIAN_POINT('Ctrl Pts',(0.175538155840648,1.,1.88742606273259));
#30572=CARTESIAN_POINT('Ctrl Pts',(0.175644148889698,1.,1.88188663145367));
#30573=CARTESIAN_POINT('Ctrl Pts',(0.175563480746485,1.,1.87563767773588));
#30574=CARTESIAN_POINT('Ctrl Pts',(0.175268337590757,1.,1.86828349694799));
#30575=CARTESIAN_POINT('Ctrl Pts',(0.17473525927603,1.,1.85948367088837));
#30576=CARTESIAN_POINT('Ctrl Pts',(0.173946627587731,1.,1.8489811319852));
#30577=CARTESIAN_POINT('Ctrl Pts',(0.1728894428919,1.,1.83658380527692));
#30578=CARTESIAN_POINT('Ctrl Pts',(0.171554770204119,1.,1.82215766811545));
#30579=CARTESIAN_POINT('Ctrl Pts',(0.169936923904608,1.,1.80561530629706));
#30580=CARTESIAN_POINT('Ctrl Pts',(0.168032772805197,1.,1.7869064998507));
#30581=CARTESIAN_POINT('Ctrl Pts',(0.1662793551464,1.,1.77018771684844));
#30582=CARTESIAN_POINT('Ctrl Pts',(0.164834765707158,1.,1.75666056638427));
#30583=CARTESIAN_POINT('Ctrl Pts',(0.163814161002002,1.,1.7472034950333));
#30584=CARTESIAN_POINT('Ctrl Pts',(0.163289472382896,1.,1.74236521665491));
#30585=CARTESIAN_POINT('',(0.0694764450219578,0.,2.19890268624765));
#30586=CARTESIAN_POINT('Origin',(-0.0694764450219586,0.,2.19890268624765));
#30587=CARTESIAN_POINT('',(-0.0694764450219586,1.,2.19890268624765));
#30588=CARTESIAN_POINT('',(0.0694764450219578,1.,2.19890268624765));
#30589=CARTESIAN_POINT('',(-0.0694764450219586,0.,2.19890268624765));
#30590=CARTESIAN_POINT('Ctrl Pts',(-0.163289472382896,-1.,1.74236521665491));
#30591=CARTESIAN_POINT('Ctrl Pts',(-0.163289472382896,1.,1.74236521665491));
#30592=CARTESIAN_POINT('Ctrl Pts',(-0.163814161002474,-1.,1.74720349503904));
#30593=CARTESIAN_POINT('Ctrl Pts',(-0.163814161002474,1.,1.74720349503904));
#30594=CARTESIAN_POINT('Ctrl Pts',(-0.164834765708484,-1.,1.75666056640041));
#30595=CARTESIAN_POINT('Ctrl Pts',(-0.164834765708484,1.,1.75666056640041));
#30596=CARTESIAN_POINT('Ctrl Pts',(-0.166279355148738,-1.,1.77018771687692));
#30597=CARTESIAN_POINT('Ctrl Pts',(-0.166279355148738,1.,1.77018771687692));
#30598=CARTESIAN_POINT('Ctrl Pts',(-0.16803277280837,-1.,1.78690649988931));
#30599=CARTESIAN_POINT('Ctrl Pts',(-0.16803277280837,1.,1.78690649988931));
#30600=CARTESIAN_POINT('Ctrl Pts',(-0.169936923908078,-1.,1.80561530633924));
#30601=CARTESIAN_POINT('Ctrl Pts',(-0.169936923908078,1.,1.80561530633924));
#30602=CARTESIAN_POINT('Ctrl Pts',(-0.171554770207306,-1.,1.82215766815414));
#30603=CARTESIAN_POINT('Ctrl Pts',(-0.171554770207306,1.,1.82215766815414));
#30604=CARTESIAN_POINT('Ctrl Pts',(-0.17288944289442,-1.,1.83658380530747));
#30605=CARTESIAN_POINT('Ctrl Pts',(-0.17288944289442,1.,1.83658380530747));
#30606=CARTESIAN_POINT('Ctrl Pts',(-0.173946627589401,-1.,1.84898113200543));
#30607=CARTESIAN_POINT('Ctrl Pts',(-0.173946627589401,1.,1.84898113200543));
#30608=CARTESIAN_POINT('Ctrl Pts',(-0.174735259276856,-1.,1.85948367089838));
#30609=CARTESIAN_POINT('Ctrl Pts',(-0.174735259276856,1.,1.85948367089838));
#30610=CARTESIAN_POINT('Ctrl Pts',(-0.175268337590901,-1.,1.86828349694972));
#30611=CARTESIAN_POINT('Ctrl Pts',(-0.175268337590901,1.,1.86828349694972));
#30612=CARTESIAN_POINT('Ctrl Pts',(-0.175563480746206,-1.,1.87563767773249));
#30613=CARTESIAN_POINT('Ctrl Pts',(-0.175563480746206,1.,1.87563767773249));
#30614=CARTESIAN_POINT('Ctrl Pts',(-0.175644148889271,-1.,1.88188663144846));
#30615=CARTESIAN_POINT('Ctrl Pts',(-0.175644148889271,1.,1.88188663144846));
#30616=CARTESIAN_POINT('Ctrl Pts',(-0.175538155840286,-1.,1.88742606272818));
#30617=CARTESIAN_POINT('Ctrl Pts',(-0.175538155840286,1.,1.88742606272818));
#30618=CARTESIAN_POINT('Ctrl Pts',(-0.175274276190664,-1.,1.89264630198279));
#30619=CARTESIAN_POINT('Ctrl Pts',(-0.175274276190664,1.,1.89264630198279));
#30620=CARTESIAN_POINT('Ctrl Pts',(-0.174879405091277,-1.,1.89788101117148));
#30621=CARTESIAN_POINT('Ctrl Pts',(-0.174879405091277,1.,1.89788101117148));
#30622=CARTESIAN_POINT('Ctrl Pts',(-0.174375518661222,-1.,1.90335253863003));
#30623=CARTESIAN_POINT('Ctrl Pts',(-0.174375518661222,1.,1.90335253863003));
#30624=CARTESIAN_POINT('Ctrl Pts',(-0.173776635257984,-1.,1.90911693975475));
#30625=CARTESIAN_POINT('Ctrl Pts',(-0.173776635257984,1.,1.90911693975475));
#30626=CARTESIAN_POINT('Ctrl Pts',(-0.173090695383619,-1.,1.91511429159681));
#30627=CARTESIAN_POINT('Ctrl Pts',(-0.173090695383619,1.,1.91511429159681));
#30628=CARTESIAN_POINT('Ctrl Pts',(-0.172321621259557,-1.,1.92122334398034));
#30629=CARTESIAN_POINT('Ctrl Pts',(-0.172321621259557,1.,1.92122334398034));
#30630=CARTESIAN_POINT('Ctrl Pts',(-0.17147119153296,-1.,1.92731093582));
#30631=CARTESIAN_POINT('Ctrl Pts',(-0.17147119153296,1.,1.92731093582));
#30632=CARTESIAN_POINT('Ctrl Pts',(-0.170541253116136,-1.,1.93329183155455));
#30633=CARTESIAN_POINT('Ctrl Pts',(-0.170541253116136,1.,1.93329183155455));
#30634=CARTESIAN_POINT('Ctrl Pts',(-0.169534904817425,-1.,1.93915639211497));
#30635=CARTESIAN_POINT('Ctrl Pts',(-0.169534904817425,1.,1.93915639211497));
#30636=CARTESIAN_POINT('Ctrl Pts',(-0.168455741607516,-1.,1.94493757756879));
#30637=CARTESIAN_POINT('Ctrl Pts',(-0.168455741607516,1.,1.94493757756879));
#30638=CARTESIAN_POINT('Ctrl Pts',(-0.167307501784469,-1.,1.95069027794286));
#30639=CARTESIAN_POINT('Ctrl Pts',(-0.167307501784469,1.,1.95069027794286));
#30640=CARTESIAN_POINT('Ctrl Pts',(-0.166093592002833,-1.,1.95646759718755));
#30641=CARTESIAN_POINT('Ctrl Pts',(-0.166093592002833,1.,1.95646759718755));
#30642=CARTESIAN_POINT('Ctrl Pts',(-0.1648165689203,-1.,1.96229379940174));
#30643=CARTESIAN_POINT('Ctrl Pts',(-0.1648165689203,1.,1.96229379940174));
#30644=CARTESIAN_POINT('Ctrl Pts',(-0.16347818545776,-1.,1.96816512678));
#30645=CARTESIAN_POINT('Ctrl Pts',(-0.16347818545776,1.,1.96816512678));
#30646=CARTESIAN_POINT('Ctrl Pts',(-0.162079693556302,-1.,1.97406280235204));
#30647=CARTESIAN_POINT('Ctrl Pts',(-0.162079693556302,1.,1.97406280235204));
#30648=CARTESIAN_POINT('Ctrl Pts',(-0.16062206078461,-1.,1.97996195437557));
#30649=CARTESIAN_POINT('Ctrl Pts',(-0.16062206078461,1.,1.97996195437557));
#30650=CARTESIAN_POINT('Ctrl Pts',(-0.159106226437289,-1.,1.98584238283279));
#30651=CARTESIAN_POINT('Ctrl Pts',(-0.159106226437289,1.,1.98584238283279));
#30652=CARTESIAN_POINT('Ctrl Pts',(-0.157533331459215,-1.,1.99169810931893));
#30653=CARTESIAN_POINT('Ctrl Pts',(-0.157533331459215,1.,1.99169810931893));
#30654=CARTESIAN_POINT('Ctrl Pts',(-0.155904629548775,-1.,1.99753284771487));
#30655=CARTESIAN_POINT('Ctrl Pts',(-0.155904629548775,1.,1.99753284771487));
#30656=CARTESIAN_POINT('Ctrl Pts',(-0.154221403049719,-1.,2.00335565310539));
#30657=CARTESIAN_POINT('Ctrl Pts',(-0.154221403049719,1.,2.00335565310539));
#30658=CARTESIAN_POINT('Ctrl Pts',(-0.152484883621452,-1.,2.00917680318426));
#30659=CARTESIAN_POINT('Ctrl Pts',(-0.152484883621452,1.,2.00917680318426));
#30660=CARTESIAN_POINT('Ctrl Pts',(-0.150696157673084,-1.,2.01500291940243));
#30661=CARTESIAN_POINT('Ctrl Pts',(-0.150696157673084,1.,2.01500291940243));
#30662=CARTESIAN_POINT('Ctrl Pts',(-0.148856124775343,-1.,2.02083464969897));
#30663=CARTESIAN_POINT('Ctrl Pts',(-0.148856124775343,1.,2.02083464969897));
#30664=CARTESIAN_POINT('Ctrl Pts',(-0.146965557332586,-1.,2.02666926182017));
#30665=CARTESIAN_POINT('Ctrl Pts',(-0.146965557332586,1.,2.02666926182017));
#30666=CARTESIAN_POINT('Ctrl Pts',(-0.145025140186058,-1.,2.03250223739941));
#30667=CARTESIAN_POINT('Ctrl Pts',(-0.145025140186058,1.,2.03250223739941));
#30668=CARTESIAN_POINT('Ctrl Pts',(-0.143035515058208,-1.,2.03832911025913));
#30669=CARTESIAN_POINT('Ctrl Pts',(-0.143035515058208,1.,2.03832911025913));
#30670=CARTESIAN_POINT('Ctrl Pts',(-0.140997332152546,-1.,2.04414757947919));
#30671=CARTESIAN_POINT('Ctrl Pts',(-0.140997332152546,1.,2.04414757947919));
#30672=CARTESIAN_POINT('Ctrl Pts',(-0.138911255368966,-1.,2.04995762001333));
#30673=CARTESIAN_POINT('Ctrl Pts',(-0.138911255368966,1.,2.04995762001333));
#30674=CARTESIAN_POINT('Ctrl Pts',(-0.136777941218044,-1.,2.0557604441427));
#30675=CARTESIAN_POINT('Ctrl Pts',(-0.136777941218044,1.,2.0557604441427));
#30676=CARTESIAN_POINT('Ctrl Pts',(-0.134598026192107,-1.,2.06155781517844));
#30677=CARTESIAN_POINT('Ctrl Pts',(-0.134598026192107,1.,2.06155781517844));
#30678=CARTESIAN_POINT('Ctrl Pts',(-0.13237211154771,-1.,2.06735123910319));
#30679=CARTESIAN_POINT('Ctrl Pts',(-0.13237211154771,1.,2.06735123910319));
#30680=CARTESIAN_POINT('Ctrl Pts',(-0.130100748328401,-1.,2.07314114713047));
#30681=CARTESIAN_POINT('Ctrl Pts',(-0.130100748328401,1.,2.07314114713047));
#30682=CARTESIAN_POINT('Ctrl Pts',(-0.127784445276116,-1.,2.07892715110967));
#30683=CARTESIAN_POINT('Ctrl Pts',(-0.127784445276116,1.,2.07892715110967));
#30684=CARTESIAN_POINT('Ctrl Pts',(-0.125423679412058,-1.,2.08470840653628));
#30685=CARTESIAN_POINT('Ctrl Pts',(-0.125423679412058,1.,2.08470840653628));
#30686=CARTESIAN_POINT('Ctrl Pts',(-0.123018905621083,-1.,2.09048392424826));
#30687=CARTESIAN_POINT('Ctrl Pts',(-0.123018905621083,1.,2.09048392424826));
#30688=CARTESIAN_POINT('Ctrl Pts',(-0.120570567965129,-1.,2.09625292867756));
#30689=CARTESIAN_POINT('Ctrl Pts',(-0.120570567965129,1.,2.09625292867756));
#30690=CARTESIAN_POINT('Ctrl Pts',(-0.118079107988368,-1.,2.10201512132945));
#30691=CARTESIAN_POINT('Ctrl Pts',(-0.118079107988368,1.,2.10201512132945));
#30692=CARTESIAN_POINT('Ctrl Pts',(-0.115544957687941,-1.,2.10777050261359));
#30693=CARTESIAN_POINT('Ctrl Pts',(-0.115544957687941,1.,2.10777050261359));
#30694=CARTESIAN_POINT('Ctrl Pts',(-0.112968534419746,-1.,2.11351924490335));
#30695=CARTESIAN_POINT('Ctrl Pts',(-0.112968534419746,1.,2.11351924490335));
#30696=CARTESIAN_POINT('Ctrl Pts',(-0.11035023613502,-1.,2.11926155590849));
#30697=CARTESIAN_POINT('Ctrl Pts',(-0.11035023613502,1.,2.11926155590849));
#30698=CARTESIAN_POINT('Ctrl Pts',(-0.107690435231068,-1.,2.12499752306927));
#30699=CARTESIAN_POINT('Ctrl Pts',(-0.107690435231068,1.,2.12499752306927));
#30700=CARTESIAN_POINT('Ctrl Pts',(-0.104989479152703,-1.,2.1307270488718));
#30701=CARTESIAN_POINT('Ctrl Pts',(-0.104989479152703,1.,2.1307270488718));
#30702=CARTESIAN_POINT('Ctrl Pts',(-0.102247700556064,-1.,2.13644992667052));
#30703=CARTESIAN_POINT('Ctrl Pts',(-0.102247700556064,1.,2.13644992667052));
#30704=CARTESIAN_POINT('Ctrl Pts',(-0.0994654261990745,-1.,2.14216588395974));
#30705=CARTESIAN_POINT('Ctrl Pts',(-0.0994654261990745,1.,2.14216588395974));
#30706=CARTESIAN_POINT('Ctrl Pts',(-0.0966429852305691,-1.,2.14787463531864));
#30707=CARTESIAN_POINT('Ctrl Pts',(-0.0966429852305691,1.,2.14787463531864));
#30708=CARTESIAN_POINT('Ctrl Pts',(-0.0937807218868348,-1.,2.15357593978377));
#30709=CARTESIAN_POINT('Ctrl Pts',(-0.0937807218868348,1.,2.15357593978377));
#30710=CARTESIAN_POINT('Ctrl Pts',(-0.0908789888108269,-1.,2.15926961544808));
#30711=CARTESIAN_POINT('Ctrl Pts',(-0.0908789888108269,1.,2.15926961544808));
#30712=CARTESIAN_POINT('Ctrl Pts',(-0.0879381291387825,-1.,2.16495552645275));
#30713=CARTESIAN_POINT('Ctrl Pts',(-0.0879381291387825,1.,2.16495552645275));
#30714=CARTESIAN_POINT('Ctrl Pts',(-0.0849584620835646,-1.,2.17063357871031));
#30715=CARTESIAN_POINT('Ctrl Pts',(-0.0849584620835646,1.,2.17063357871031));
#30716=CARTESIAN_POINT('Ctrl Pts',(-0.0819402680871942,-1.,2.1763037121106));
#30717=CARTESIAN_POINT('Ctrl Pts',(-0.0819402680871942,1.,2.1763037121106));
#30718=CARTESIAN_POINT('Ctrl Pts',(-0.078883772768323,-1.,2.18196589448304));
#30719=CARTESIAN_POINT('Ctrl Pts',(-0.078883772768323,1.,2.18196589448304));
#30720=CARTESIAN_POINT('Ctrl Pts',(-0.0757891465833414,-1.,2.1876201139874));
#30721=CARTESIAN_POINT('Ctrl Pts',(-0.0757891465833414,1.,2.1876201139874));
#30722=CARTESIAN_POINT('Ctrl Pts',(-0.0732830357304279,-1.,2.19213712012956));
#30723=CARTESIAN_POINT('Ctrl Pts',(-0.0732830357304279,1.,2.19213712012956));
#30724=CARTESIAN_POINT('Ctrl Pts',(-0.071386377952463,-1.,2.19552129483562));
#30725=CARTESIAN_POINT('Ctrl Pts',(-0.071386377952463,1.,2.19552129483562));
#30726=CARTESIAN_POINT('Ctrl Pts',(-0.0701143536324929,-1.,2.19777582085261));
#30727=CARTESIAN_POINT('Ctrl Pts',(-0.0701143536324929,1.,2.19777582085261));
#30728=CARTESIAN_POINT('Ctrl Pts',(-0.0694764450219586,-1.,2.19890268624765));
#30729=CARTESIAN_POINT('Ctrl Pts',(-0.0694764450219586,1.,2.19890268624765));
#30730=CARTESIAN_POINT('',(-0.163289472382896,1.,1.74236521665491));
#30731=CARTESIAN_POINT('Ctrl Pts',(-0.163289472382896,1.,1.74236521665491));
#30732=CARTESIAN_POINT('Ctrl Pts',(-0.163814161002474,1.,1.74720349503904));
#30733=CARTESIAN_POINT('Ctrl Pts',(-0.164834765708484,1.,1.75666056640041));
#30734=CARTESIAN_POINT('Ctrl Pts',(-0.166279355148738,1.,1.77018771687692));
#30735=CARTESIAN_POINT('Ctrl Pts',(-0.16803277280837,1.,1.78690649988931));
#30736=CARTESIAN_POINT('Ctrl Pts',(-0.169936923908078,1.,1.80561530633924));
#30737=CARTESIAN_POINT('Ctrl Pts',(-0.171554770207306,1.,1.82215766815414));
#30738=CARTESIAN_POINT('Ctrl Pts',(-0.17288944289442,1.,1.83658380530747));
#30739=CARTESIAN_POINT('Ctrl Pts',(-0.173946627589401,1.,1.84898113200543));
#30740=CARTESIAN_POINT('Ctrl Pts',(-0.174735259276856,1.,1.85948367089838));
#30741=CARTESIAN_POINT('Ctrl Pts',(-0.175268337590901,1.,1.86828349694972));
#30742=CARTESIAN_POINT('Ctrl Pts',(-0.175563480746206,1.,1.87563767773249));
#30743=CARTESIAN_POINT('Ctrl Pts',(-0.175644148889271,1.,1.88188663144846));
#30744=CARTESIAN_POINT('Ctrl Pts',(-0.175538155840286,1.,1.88742606272818));
#30745=CARTESIAN_POINT('Ctrl Pts',(-0.175274276190664,1.,1.89264630198279));
#30746=CARTESIAN_POINT('Ctrl Pts',(-0.174879405091277,1.,1.89788101117148));
#30747=CARTESIAN_POINT('Ctrl Pts',(-0.174375518661222,1.,1.90335253863003));
#30748=CARTESIAN_POINT('Ctrl Pts',(-0.173776635257984,1.,1.90911693975475));
#30749=CARTESIAN_POINT('Ctrl Pts',(-0.173090695383619,1.,1.91511429159681));
#30750=CARTESIAN_POINT('Ctrl Pts',(-0.172321621259557,1.,1.92122334398034));
#30751=CARTESIAN_POINT('Ctrl Pts',(-0.17147119153296,1.,1.92731093582));
#30752=CARTESIAN_POINT('Ctrl Pts',(-0.170541253116136,1.,1.93329183155455));
#30753=CARTESIAN_POINT('Ctrl Pts',(-0.169534904817425,1.,1.93915639211497));
#30754=CARTESIAN_POINT('Ctrl Pts',(-0.168455741607516,1.,1.94493757756879));
#30755=CARTESIAN_POINT('Ctrl Pts',(-0.167307501784469,1.,1.95069027794286));
#30756=CARTESIAN_POINT('Ctrl Pts',(-0.166093592002833,1.,1.95646759718755));
#30757=CARTESIAN_POINT('Ctrl Pts',(-0.1648165689203,1.,1.96229379940174));
#30758=CARTESIAN_POINT('Ctrl Pts',(-0.16347818545776,1.,1.96816512678));
#30759=CARTESIAN_POINT('Ctrl Pts',(-0.162079693556302,1.,1.97406280235204));
#30760=CARTESIAN_POINT('Ctrl Pts',(-0.16062206078461,1.,1.97996195437557));
#30761=CARTESIAN_POINT('Ctrl Pts',(-0.159106226437289,1.,1.98584238283279));
#30762=CARTESIAN_POINT('Ctrl Pts',(-0.157533331459215,1.,1.99169810931893));
#30763=CARTESIAN_POINT('Ctrl Pts',(-0.155904629548775,1.,1.99753284771487));
#30764=CARTESIAN_POINT('Ctrl Pts',(-0.154221403049719,1.,2.00335565310539));
#30765=CARTESIAN_POINT('Ctrl Pts',(-0.152484883621452,1.,2.00917680318426));
#30766=CARTESIAN_POINT('Ctrl Pts',(-0.150696157673084,1.,2.01500291940243));
#30767=CARTESIAN_POINT('Ctrl Pts',(-0.148856124775343,1.,2.02083464969897));
#30768=CARTESIAN_POINT('Ctrl Pts',(-0.146965557332586,1.,2.02666926182017));
#30769=CARTESIAN_POINT('Ctrl Pts',(-0.145025140186058,1.,2.03250223739941));
#30770=CARTESIAN_POINT('Ctrl Pts',(-0.143035515058208,1.,2.03832911025913));
#30771=CARTESIAN_POINT('Ctrl Pts',(-0.140997332152546,1.,2.04414757947919));
#30772=CARTESIAN_POINT('Ctrl Pts',(-0.138911255368966,1.,2.04995762001333));
#30773=CARTESIAN_POINT('Ctrl Pts',(-0.136777941218044,1.,2.0557604441427));
#30774=CARTESIAN_POINT('Ctrl Pts',(-0.134598026192107,1.,2.06155781517844));
#30775=CARTESIAN_POINT('Ctrl Pts',(-0.13237211154771,1.,2.06735123910319));
#30776=CARTESIAN_POINT('Ctrl Pts',(-0.130100748328401,1.,2.07314114713047));
#30777=CARTESIAN_POINT('Ctrl Pts',(-0.127784445276116,1.,2.07892715110967));
#30778=CARTESIAN_POINT('Ctrl Pts',(-0.125423679412058,1.,2.08470840653628));
#30779=CARTESIAN_POINT('Ctrl Pts',(-0.123018905621083,1.,2.09048392424826));
#30780=CARTESIAN_POINT('Ctrl Pts',(-0.120570567965129,1.,2.09625292867756));
#30781=CARTESIAN_POINT('Ctrl Pts',(-0.118079107988368,1.,2.10201512132945));
#30782=CARTESIAN_POINT('Ctrl Pts',(-0.115544957687941,1.,2.10777050261359));
#30783=CARTESIAN_POINT('Ctrl Pts',(-0.112968534419746,1.,2.11351924490335));
#30784=CARTESIAN_POINT('Ctrl Pts',(-0.11035023613502,1.,2.11926155590849));
#30785=CARTESIAN_POINT('Ctrl Pts',(-0.107690435231068,1.,2.12499752306927));
#30786=CARTESIAN_POINT('Ctrl Pts',(-0.104989479152703,1.,2.1307270488718));
#30787=CARTESIAN_POINT('Ctrl Pts',(-0.102247700556064,1.,2.13644992667052));
#30788=CARTESIAN_POINT('Ctrl Pts',(-0.0994654261990745,1.,2.14216588395974));
#30789=CARTESIAN_POINT('Ctrl Pts',(-0.0966429852305691,1.,2.14787463531864));
#30790=CARTESIAN_POINT('Ctrl Pts',(-0.0937807218868348,1.,2.15357593978377));
#30791=CARTESIAN_POINT('Ctrl Pts',(-0.0908789888108269,1.,2.15926961544808));
#30792=CARTESIAN_POINT('Ctrl Pts',(-0.0879381291387825,1.,2.16495552645275));
#30793=CARTESIAN_POINT('Ctrl Pts',(-0.0849584620835646,1.,2.17063357871031));
#30794=CARTESIAN_POINT('Ctrl Pts',(-0.0819402680871942,1.,2.1763037121106));
#30795=CARTESIAN_POINT('Ctrl Pts',(-0.078883772768323,1.,2.18196589448304));
#30796=CARTESIAN_POINT('Ctrl Pts',(-0.0757891465833414,1.,2.1876201139874));
#30797=CARTESIAN_POINT('Ctrl Pts',(-0.0732830357304279,1.,2.19213712012956));
#30798=CARTESIAN_POINT('Ctrl Pts',(-0.071386377952463,1.,2.19552129483562));
#30799=CARTESIAN_POINT('Ctrl Pts',(-0.0701143536324929,1.,2.19777582085261));
#30800=CARTESIAN_POINT('Ctrl Pts',(-0.0694764450219586,1.,2.19890268624765));
#30801=CARTESIAN_POINT('',(-0.163289472382897,0.,1.74236521665491));
#30802=CARTESIAN_POINT('Origin',(0.,0.,0.));
#30803=CARTESIAN_POINT('',(-0.383122945602004,1.,1.7075470150345));
#30804=CARTESIAN_POINT('Origin',(0.,1.,0.));
#30805=CARTESIAN_POINT('',(-0.383122945602004,0.,1.7075470150345));
#30806=CARTESIAN_POINT('Ctrl Pts',(-0.61342227326009,-1.,2.11275013067528));
#30807=CARTESIAN_POINT('Ctrl Pts',(-0.61342227326009,1.,2.11275013067528));
#30808=CARTESIAN_POINT('Ctrl Pts',(-0.61246736556225,-1.,2.11187554260142));
#30809=CARTESIAN_POINT('Ctrl Pts',(-0.61246736556225,1.,2.11187554260142));
#30810=CARTESIAN_POINT('Ctrl Pts',(-0.610560911691113,-1.,2.11012443807661));
#30811=CARTESIAN_POINT('Ctrl Pts',(-0.610560911691113,1.,2.11012443807661));
#30812=CARTESIAN_POINT('Ctrl Pts',(-0.607711315456826,-1.,2.10749199615859));
#30813=CARTESIAN_POINT('Ctrl Pts',(-0.607711315456826,1.,2.10749199615859));
#30814=CARTESIAN_POINT('Ctrl Pts',(-0.603932030738212,-1.,2.10397049887709));
#30815=CARTESIAN_POINT('Ctrl Pts',(-0.603932030738212,1.,2.10397049887709));
#30816=CARTESIAN_POINT('Ctrl Pts',(-0.599241616422144,-1.,2.09954930865331));
#30817=CARTESIAN_POINT('Ctrl Pts',(-0.599241616422144,1.,2.09954930865331));
#30818=CARTESIAN_POINT('Ctrl Pts',(-0.594585006052824,-1.,2.09510876220501));
#30819=CARTESIAN_POINT('Ctrl Pts',(-0.594585006052824,1.,2.09510876220501));
#30820=CARTESIAN_POINT('Ctrl Pts',(-0.589962365403189,-1.,2.09064881812053));
#30821=CARTESIAN_POINT('Ctrl Pts',(-0.589962365403189,1.,2.09064881812053));
#30822=CARTESIAN_POINT('Ctrl Pts',(-0.585373918990895,-1.,2.086169437277));
#30823=CARTESIAN_POINT('Ctrl Pts',(-0.585373918990895,1.,2.086169437277));
#30824=CARTESIAN_POINT('Ctrl Pts',(-0.580819952107257,-1.,2.08167059018138));
#30825=CARTESIAN_POINT('Ctrl Pts',(-0.580819952107257,1.,2.08167059018138));
#30826=CARTESIAN_POINT('Ctrl Pts',(-0.576300797416275,-1.,2.07715226767361));
#30827=CARTESIAN_POINT('Ctrl Pts',(-0.576300797416275,1.,2.07715226767361));
#30828=CARTESIAN_POINT('Ctrl Pts',(-0.571816823242411,-1.,2.07261449292757));
#30829=CARTESIAN_POINT('Ctrl Pts',(-0.571816823242411,1.,2.07261449292757));
#30830=CARTESIAN_POINT('Ctrl Pts',(-0.567368421181229,-1.,2.06805732997383));
#30831=CARTESIAN_POINT('Ctrl Pts',(-0.567368421181229,1.,2.06805732997383));
#30832=CARTESIAN_POINT('Ctrl Pts',(-0.562955993082574,-1.,2.06348090160697));
#30833=CARTESIAN_POINT('Ctrl Pts',(-0.562955993082574,1.,2.06348090160697));
#30834=CARTESIAN_POINT('Ctrl Pts',(-0.558579940185467,-1.,2.05888537756571));
#30835=CARTESIAN_POINT('Ctrl Pts',(-0.558579940185467,1.,2.05888537756571));
#30836=CARTESIAN_POINT('Ctrl Pts',(-0.55424065746411,-1.,2.05427091604482));
#30837=CARTESIAN_POINT('Ctrl Pts',(-0.55424065746411,1.,2.05427091604482));
#30838=CARTESIAN_POINT('Ctrl Pts',(-0.549938525150342,-1.,2.04963761077974));
#30839=CARTESIAN_POINT('Ctrl Pts',(-0.549938525150342,1.,2.04963761077974));
#30840=CARTESIAN_POINT('Ctrl Pts',(-0.545673903817348,-1.,2.0449854471456));
#30841=CARTESIAN_POINT('Ctrl Pts',(-0.545673903817348,1.,2.0449854471456));
#30842=CARTESIAN_POINT('Ctrl Pts',(-0.54144712061552,-1.,2.0403142269048));
#30843=CARTESIAN_POINT('Ctrl Pts',(-0.54144712061552,1.,2.0403142269048));
#30844=CARTESIAN_POINT('Ctrl Pts',(-0.537258489833134,-1.,2.03562362953993));
#30845=CARTESIAN_POINT('Ctrl Pts',(-0.537258489833134,1.,2.03562362953993));
#30846=CARTESIAN_POINT('Ctrl Pts',(-0.533108355132905,-1.,2.03091336214401));
#30847=CARTESIAN_POINT('Ctrl Pts',(-0.533108355132905,1.,2.03091336214401));
#30848=CARTESIAN_POINT('Ctrl Pts',(-0.528997127241911,-1.,2.02618329083289));
#30849=CARTESIAN_POINT('Ctrl Pts',(-0.528997127241911,1.,2.02618329083289));
#30850=CARTESIAN_POINT('Ctrl Pts',(-0.524925318333518,-1.,2.02143356304712));
#30851=CARTESIAN_POINT('Ctrl Pts',(-0.524925318333518,1.,2.02143356304712));
#30852=CARTESIAN_POINT('Ctrl Pts',(-0.520893590399428,-1.,2.01666477917305));
#30853=CARTESIAN_POINT('Ctrl Pts',(-0.520893590399428,1.,2.01666477917305));
#30854=CARTESIAN_POINT('Ctrl Pts',(-0.516902681728733,-1.,2.01187773939257));
#30855=CARTESIAN_POINT('Ctrl Pts',(-0.516902681728733,1.,2.01187773939257));
#30856=CARTESIAN_POINT('Ctrl Pts',(-0.512953306961814,-1.,2.00707309946955));
#30857=CARTESIAN_POINT('Ctrl Pts',(-0.512953306961814,1.,2.00707309946955));
#30858=CARTESIAN_POINT('Ctrl Pts',(-0.509046069886152,-1.,2.00225107134733));
#30859=CARTESIAN_POINT('Ctrl Pts',(-0.509046069886152,1.,2.00225107134733));
#30860=CARTESIAN_POINT('Ctrl Pts',(-0.505181361323011,-1.,1.99741107463567));
#30861=CARTESIAN_POINT('Ctrl Pts',(-0.505181361323011,1.,1.99741107463567));
#30862=CARTESIAN_POINT('Ctrl Pts',(-0.501359287727129,-1.,1.9925514912615));
#30863=CARTESIAN_POINT('Ctrl Pts',(-0.501359287727129,1.,1.9925514912615));
#30864=CARTESIAN_POINT('Ctrl Pts',(-0.497579909545564,-1.,1.98767044752929));
#30865=CARTESIAN_POINT('Ctrl Pts',(-0.497579909545564,1.,1.98767044752929));
#30866=CARTESIAN_POINT('Ctrl Pts',(-0.493843476541492,-1.,1.9827665876182));
#30867=CARTESIAN_POINT('Ctrl Pts',(-0.493843476541492,1.,1.9827665876182));
#30868=CARTESIAN_POINT('Ctrl Pts',(-0.490150627860955,-1.,1.97783973019229));
#30869=CARTESIAN_POINT('Ctrl Pts',(-0.490150627860955,1.,1.97783973019229));
#30870=CARTESIAN_POINT('Ctrl Pts',(-0.486502692907661,-1.,1.97289186263272));
#30871=CARTESIAN_POINT('Ctrl Pts',(-0.486502692907661,1.,1.97289186263272));
#30872=CARTESIAN_POINT('Ctrl Pts',(-0.482901662120687,-1.,1.96792703422358));
#30873=CARTESIAN_POINT('Ctrl Pts',(-0.482901662120687,1.,1.96792703422358));
#30874=CARTESIAN_POINT('Ctrl Pts',(-0.479349583074846,-1.,1.96294933055938));
#30875=CARTESIAN_POINT('Ctrl Pts',(-0.479349583074846,1.,1.96294933055938));
#30876=CARTESIAN_POINT('Ctrl Pts',(-0.475848034683172,-1.,1.95796111148175));
#30877=CARTESIAN_POINT('Ctrl Pts',(-0.475848034683172,1.,1.95796111148175));
#30878=CARTESIAN_POINT('Ctrl Pts',(-0.47239767226408,-1.,1.95296148278136));
#30879=CARTESIAN_POINT('Ctrl Pts',(-0.47239767226408,1.,1.95296148278136));
#30880=CARTESIAN_POINT('Ctrl Pts',(-0.468997482913158,-1.,1.94794381136524));
#30881=CARTESIAN_POINT('Ctrl Pts',(-0.468997482913158,1.,1.94794381136524));
#30882=CARTESIAN_POINT('Ctrl Pts',(-0.465645462026065,-1.,1.94289794196205));
#30883=CARTESIAN_POINT('Ctrl Pts',(-0.465645462026065,1.,1.94289794196205));
#30884=CARTESIAN_POINT('Ctrl Pts',(-0.462340031009087,-1.,1.93781486640834));
#30885=CARTESIAN_POINT('Ctrl Pts',(-0.462340031009087,1.,1.93781486640834));
#30886=CARTESIAN_POINT('Ctrl Pts',(-0.459081234547931,-1.,1.93269066517936));
#30887=CARTESIAN_POINT('Ctrl Pts',(-0.459081234547931,1.,1.93269066517936));
#30888=CARTESIAN_POINT('Ctrl Pts',(-0.455872005174335,-1.,1.92753067150461));
#30889=CARTESIAN_POINT('Ctrl Pts',(-0.455872005174335,1.,1.92753067150461));
#30890=CARTESIAN_POINT('Ctrl Pts',(-0.452719478359356,-1.,1.9223538064847));
#30891=CARTESIAN_POINT('Ctrl Pts',(-0.452719478359356,1.,1.9223538064847));
#30892=CARTESIAN_POINT('Ctrl Pts',(-0.449632260106572,-1.,1.91718342555717));
#30893=CARTESIAN_POINT('Ctrl Pts',(-0.449632260106572,1.,1.91718342555717));
#30894=CARTESIAN_POINT('Ctrl Pts',(-0.446617343485651,-1.,1.91203699981095));
#30895=CARTESIAN_POINT('Ctrl Pts',(-0.446617343485651,1.,1.91203699981095));
#30896=CARTESIAN_POINT('Ctrl Pts',(-0.44367755684917,-1.,1.90691756144906));
#30897=CARTESIAN_POINT('Ctrl Pts',(-0.44367755684917,1.,1.90691756144906));
#30898=CARTESIAN_POINT('Ctrl Pts',(-0.440807833704161,-1.,1.90180124389137));
#30899=CARTESIAN_POINT('Ctrl Pts',(-0.440807833704161,1.,1.90180124389137));
#30900=CARTESIAN_POINT('Ctrl Pts',(-0.437995003948443,-1.,1.89663648956549));
#30901=CARTESIAN_POINT('Ctrl Pts',(-0.437995003948443,1.,1.89663648956549));
#30902=CARTESIAN_POINT('Ctrl Pts',(-0.43522566096358,-1.,1.89136993975585));
#30903=CARTESIAN_POINT('Ctrl Pts',(-0.43522566096358,1.,1.89136993975585));
#30904=CARTESIAN_POINT('Ctrl Pts',(-0.432493038548833,-1.,1.88596913666828));
#30905=CARTESIAN_POINT('Ctrl Pts',(-0.432493038548833,1.,1.88596913666828));
#30906=CARTESIAN_POINT('Ctrl Pts',(-0.429803062482217,-1.,1.88044229001778));
#30907=CARTESIAN_POINT('Ctrl Pts',(-0.429803062482217,1.,1.88044229001778));
#30908=CARTESIAN_POINT('Ctrl Pts',(-0.427183828518743,-1.,1.87486989291333));
#30909=CARTESIAN_POINT('Ctrl Pts',(-0.427183828518743,1.,1.87486989291333));
#30910=CARTESIAN_POINT('Ctrl Pts',(-0.424678177290876,-1.,1.8693780394412));
#30911=CARTESIAN_POINT('Ctrl Pts',(-0.424678177290876,1.,1.8693780394412));
#30912=CARTESIAN_POINT('Ctrl Pts',(-0.422327307417885,-1.,1.86408083333863));
#30913=CARTESIAN_POINT('Ctrl Pts',(-0.422327307417885,1.,1.86408083333863));
#30914=CARTESIAN_POINT('Ctrl Pts',(-0.420157287975583,-1.,1.8590328109667));
#30915=CARTESIAN_POINT('Ctrl Pts',(-0.420157287975583,1.,1.8590328109667));
#30916=CARTESIAN_POINT('Ctrl Pts',(-0.418164129144045,-1.,1.8541763285645));
#30917=CARTESIAN_POINT('Ctrl Pts',(-0.418164129144045,1.,1.8541763285645));
#30918=CARTESIAN_POINT('Ctrl Pts',(-0.416300022039885,-1.,1.84929312930314));
#30919=CARTESIAN_POINT('Ctrl Pts',(-0.416300022039885,1.,1.84929312930314));
#30920=CARTESIAN_POINT('Ctrl Pts',(-0.414487438255542,-1.,1.84405757074218));
#30921=CARTESIAN_POINT('Ctrl Pts',(-0.414487438255542,1.,1.84405757074218));
#30922=CARTESIAN_POINT('Ctrl Pts',(-0.412633125322945,-1.,1.8380895347617));
#30923=CARTESIAN_POINT('Ctrl Pts',(-0.412633125322945,1.,1.8380895347617));
#30924=CARTESIAN_POINT('Ctrl Pts',(-0.410641256301276,-1.,1.83100408895047));
#30925=CARTESIAN_POINT('Ctrl Pts',(-0.410641256301276,1.,1.83100408895047));
#30926=CARTESIAN_POINT('Ctrl Pts',(-0.408428948106227,-1.,1.82247022677562));
#30927=CARTESIAN_POINT('Ctrl Pts',(-0.408428948106227,1.,1.82247022677562));
#30928=CARTESIAN_POINT('Ctrl Pts',(-0.405933518407175,-1.,1.81223801812013));
#30929=CARTESIAN_POINT('Ctrl Pts',(-0.405933518407175,1.,1.81223801812013));
#30930=CARTESIAN_POINT('Ctrl Pts',(-0.403107976163396,-1.,1.80012077173238));
#30931=CARTESIAN_POINT('Ctrl Pts',(-0.403107976163396,1.,1.80012077173238));
#30932=CARTESIAN_POINT('Ctrl Pts',(-0.399919403774155,-1.,1.78598826343754));
#30933=CARTESIAN_POINT('Ctrl Pts',(-0.399919403774155,1.,1.78598826343754));
#30934=CARTESIAN_POINT('Ctrl Pts',(-0.396346196110688,-1.,1.76975560043442));
#30935=CARTESIAN_POINT('Ctrl Pts',(-0.396346196110688,1.,1.76975560043442));
#30936=CARTESIAN_POINT('Ctrl Pts',(-0.392375812285395,-1.,1.75137405310193));
#30937=CARTESIAN_POINT('Ctrl Pts',(-0.392375812285395,1.,1.75137405310193));
#30938=CARTESIAN_POINT('Ctrl Pts',(-0.388877023502615,-1.,1.73493170972829));
#30939=CARTESIAN_POINT('Ctrl Pts',(-0.388877023502615,1.,1.73493170972829));
#30940=CARTESIAN_POINT('Ctrl Pts',(-0.386070790323281,-1.,1.72162022244582));
#30941=CARTESIAN_POINT('Ctrl Pts',(-0.386070790323281,1.,1.72162022244582));
#30942=CARTESIAN_POINT('Ctrl Pts',(-0.384119047314215,-1.,1.71231062891398));
#30943=CARTESIAN_POINT('Ctrl Pts',(-0.384119047314215,1.,1.71231062891398));
#30944=CARTESIAN_POINT('Ctrl Pts',(-0.383122945602004,-1.,1.7075470150345));
#30945=CARTESIAN_POINT('Ctrl Pts',(-0.383122945602004,1.,1.7075470150345));
#30946=CARTESIAN_POINT('',(-0.61342227326009,1.,2.11275013067528));
#30947=CARTESIAN_POINT('Ctrl Pts',(-0.61342227326009,1.,2.11275013067528));
#30948=CARTESIAN_POINT('Ctrl Pts',(-0.61246736556225,1.,2.11187554260142));
#30949=CARTESIAN_POINT('Ctrl Pts',(-0.610560911691113,1.,2.11012443807661));
#30950=CARTESIAN_POINT('Ctrl Pts',(-0.607711315456826,1.,2.10749199615859));
#30951=CARTESIAN_POINT('Ctrl Pts',(-0.603932030738212,1.,2.10397049887709));
#30952=CARTESIAN_POINT('Ctrl Pts',(-0.599241616422144,1.,2.09954930865331));
#30953=CARTESIAN_POINT('Ctrl Pts',(-0.594585006052824,1.,2.09510876220501));
#30954=CARTESIAN_POINT('Ctrl Pts',(-0.589962365403189,1.,2.09064881812053));
#30955=CARTESIAN_POINT('Ctrl Pts',(-0.585373918990895,1.,2.086169437277));
#30956=CARTESIAN_POINT('Ctrl Pts',(-0.580819952107257,1.,2.08167059018138));
#30957=CARTESIAN_POINT('Ctrl Pts',(-0.576300797416275,1.,2.07715226767361));
#30958=CARTESIAN_POINT('Ctrl Pts',(-0.571816823242411,1.,2.07261449292757));
#30959=CARTESIAN_POINT('Ctrl Pts',(-0.567368421181229,1.,2.06805732997383));
#30960=CARTESIAN_POINT('Ctrl Pts',(-0.562955993082574,1.,2.06348090160697));
#30961=CARTESIAN_POINT('Ctrl Pts',(-0.558579940185467,1.,2.05888537756571));
#30962=CARTESIAN_POINT('Ctrl Pts',(-0.55424065746411,1.,2.05427091604482));
#30963=CARTESIAN_POINT('Ctrl Pts',(-0.549938525150342,1.,2.04963761077974));
#30964=CARTESIAN_POINT('Ctrl Pts',(-0.545673903817348,1.,2.0449854471456));
#30965=CARTESIAN_POINT('Ctrl Pts',(-0.54144712061552,1.,2.0403142269048));
#30966=CARTESIAN_POINT('Ctrl Pts',(-0.537258489833134,1.,2.03562362953993));
#30967=CARTESIAN_POINT('Ctrl Pts',(-0.533108355132905,1.,2.03091336214401));
#30968=CARTESIAN_POINT('Ctrl Pts',(-0.528997127241911,1.,2.02618329083289));
#30969=CARTESIAN_POINT('Ctrl Pts',(-0.524925318333518,1.,2.02143356304712));
#30970=CARTESIAN_POINT('Ctrl Pts',(-0.520893590399428,1.,2.01666477917305));
#30971=CARTESIAN_POINT('Ctrl Pts',(-0.516902681728733,1.,2.01187773939257));
#30972=CARTESIAN_POINT('Ctrl Pts',(-0.512953306961814,1.,2.00707309946955));
#30973=CARTESIAN_POINT('Ctrl Pts',(-0.509046069886152,1.,2.00225107134733));
#30974=CARTESIAN_POINT('Ctrl Pts',(-0.505181361323011,1.,1.99741107463567));
#30975=CARTESIAN_POINT('Ctrl Pts',(-0.501359287727129,1.,1.9925514912615));
#30976=CARTESIAN_POINT('Ctrl Pts',(-0.497579909545564,1.,1.98767044752929));
#30977=CARTESIAN_POINT('Ctrl Pts',(-0.493843476541492,1.,1.9827665876182));
#30978=CARTESIAN_POINT('Ctrl Pts',(-0.490150627860955,1.,1.97783973019229));
#30979=CARTESIAN_POINT('Ctrl Pts',(-0.486502692907661,1.,1.97289186263272));
#30980=CARTESIAN_POINT('Ctrl Pts',(-0.482901662120687,1.,1.96792703422358));
#30981=CARTESIAN_POINT('Ctrl Pts',(-0.479349583074846,1.,1.96294933055938));
#30982=CARTESIAN_POINT('Ctrl Pts',(-0.475848034683172,1.,1.95796111148175));
#30983=CARTESIAN_POINT('Ctrl Pts',(-0.47239767226408,1.,1.95296148278136));
#30984=CARTESIAN_POINT('Ctrl Pts',(-0.468997482913158,1.,1.94794381136524));
#30985=CARTESIAN_POINT('Ctrl Pts',(-0.465645462026065,1.,1.94289794196205));
#30986=CARTESIAN_POINT('Ctrl Pts',(-0.462340031009087,1.,1.93781486640834));
#30987=CARTESIAN_POINT('Ctrl Pts',(-0.459081234547931,1.,1.93269066517936));
#30988=CARTESIAN_POINT('Ctrl Pts',(-0.455872005174335,1.,1.92753067150461));
#30989=CARTESIAN_POINT('Ctrl Pts',(-0.452719478359356,1.,1.9223538064847));
#30990=CARTESIAN_POINT('Ctrl Pts',(-0.449632260106572,1.,1.91718342555717));
#30991=CARTESIAN_POINT('Ctrl Pts',(-0.446617343485651,1.,1.91203699981095));
#30992=CARTESIAN_POINT('Ctrl Pts',(-0.44367755684917,1.,1.90691756144906));
#30993=CARTESIAN_POINT('Ctrl Pts',(-0.440807833704161,1.,1.90180124389137));
#30994=CARTESIAN_POINT('Ctrl Pts',(-0.437995003948443,1.,1.89663648956549));
#30995=CARTESIAN_POINT('Ctrl Pts',(-0.43522566096358,1.,1.89136993975585));
#30996=CARTESIAN_POINT('Ctrl Pts',(-0.432493038548833,1.,1.88596913666828));
#30997=CARTESIAN_POINT('Ctrl Pts',(-0.429803062482217,1.,1.88044229001778));
#30998=CARTESIAN_POINT('Ctrl Pts',(-0.427183828518743,1.,1.87486989291333));
#30999=CARTESIAN_POINT('Ctrl Pts',(-0.424678177290876,1.,1.8693780394412));
#31000=CARTESIAN_POINT('Ctrl Pts',(-0.422327307417885,1.,1.86408083333863));
#31001=CARTESIAN_POINT('Ctrl Pts',(-0.420157287975583,1.,1.8590328109667));
#31002=CARTESIAN_POINT('Ctrl Pts',(-0.418164129144045,1.,1.8541763285645));
#31003=CARTESIAN_POINT('Ctrl Pts',(-0.416300022039885,1.,1.84929312930314));
#31004=CARTESIAN_POINT('Ctrl Pts',(-0.414487438255542,1.,1.84405757074218));
#31005=CARTESIAN_POINT('Ctrl Pts',(-0.412633125322945,1.,1.8380895347617));
#31006=CARTESIAN_POINT('Ctrl Pts',(-0.410641256301276,1.,1.83100408895047));
#31007=CARTESIAN_POINT('Ctrl Pts',(-0.408428948106227,1.,1.82247022677562));
#31008=CARTESIAN_POINT('Ctrl Pts',(-0.405933518407175,1.,1.81223801812013));
#31009=CARTESIAN_POINT('Ctrl Pts',(-0.403107976163396,1.,1.80012077173238));
#31010=CARTESIAN_POINT('Ctrl Pts',(-0.399919403774155,1.,1.78598826343754));
#31011=CARTESIAN_POINT('Ctrl Pts',(-0.396346196110688,1.,1.76975560043442));
#31012=CARTESIAN_POINT('Ctrl Pts',(-0.392375812285395,1.,1.75137405310193));
#31013=CARTESIAN_POINT('Ctrl Pts',(-0.388877023502615,1.,1.73493170972829));
#31014=CARTESIAN_POINT('Ctrl Pts',(-0.386070790323281,1.,1.72162022244582));
#31015=CARTESIAN_POINT('Ctrl Pts',(-0.384119047314215,1.,1.71231062891398));
#31016=CARTESIAN_POINT('Ctrl Pts',(-0.383122945602004,1.,1.7075470150345));
#31017=CARTESIAN_POINT('',(-0.61342227326009,0.,2.11275013067528));
#31018=CARTESIAN_POINT('Origin',(-0.745574324794401,0.,2.0698113262342));
#31019=CARTESIAN_POINT('',(-0.745574324794401,1.,2.0698113262342));
#31020=CARTESIAN_POINT('',(-0.61342227326009,1.,2.11275013067528));
#31021=CARTESIAN_POINT('',(-0.745574324794401,0.,2.0698113262342));
#31022=CARTESIAN_POINT('Ctrl Pts',(-0.693717979106306,-1.,1.60662857109684));
#31023=CARTESIAN_POINT('Ctrl Pts',(-0.693717979106306,1.,1.60662857109684));
#31024=CARTESIAN_POINT('Ctrl Pts',(-0.695712097881194,-1.,1.61106790958151));
#31025=CARTESIAN_POINT('Ctrl Pts',(-0.695712097881194,1.,1.61106790958151));
#31026=CARTESIAN_POINT('Ctrl Pts',(-0.699605146405088,-1.,1.61974673472612));
#31027=CARTESIAN_POINT('Ctrl Pts',(-0.699605146405088,1.,1.61974673472612));
#31028=CARTESIAN_POINT('Ctrl Pts',(-0.705159151988319,-1.,1.63216541664676));
#31029=CARTESIAN_POINT('Ctrl Pts',(-0.705159151988319,1.,1.63216541664676));
#31030=CARTESIAN_POINT('Ctrl Pts',(-0.711993139355394,-1.,1.64752408832016));
#31031=CARTESIAN_POINT('Ctrl Pts',(-0.711993139355394,1.,1.64752408832016));
#31032=CARTESIAN_POINT('Ctrl Pts',(-0.719585433804282,-1.,1.6647288055568));
#31033=CARTESIAN_POINT('Ctrl Pts',(-0.719585433804282,1.,1.6647288055568));
#31034=CARTESIAN_POINT('Ctrl Pts',(-0.726235967997433,-1.,1.67996158455503));
#31035=CARTESIAN_POINT('Ctrl Pts',(-0.726235967997433,1.,1.67996158455503));
#31036=CARTESIAN_POINT('Ctrl Pts',(-0.731963238697195,-1.,1.69326921975743));
#31037=CARTESIAN_POINT('Ctrl Pts',(-0.731963238697195,1.,1.69326921975743));
#31038=CARTESIAN_POINT('Ctrl Pts',(-0.736799665724771,-1.,1.70473309006121));
#31039=CARTESIAN_POINT('Ctrl Pts',(-0.736799665724771,1.,1.70473309006121));
#31040=CARTESIAN_POINT('Ctrl Pts',(-0.740795162032088,-1.,1.71447789751927));
#31041=CARTESIAN_POINT('Ctrl Pts',(-0.740795162032088,1.,1.71447789751927));
#31042=CARTESIAN_POINT('Ctrl Pts',(-0.744021445433764,-1.,1.7226822991693));
#31043=CARTESIAN_POINT('Ctrl Pts',(-0.744021445433764,1.,1.7226822991693));
#31044=CARTESIAN_POINT('Ctrl Pts',(-0.746574710096436,-1.,1.72958533647399));
#31045=CARTESIAN_POINT('Ctrl Pts',(-0.746574710096436,1.,1.72958533647399));
#31046=CARTESIAN_POINT('Ctrl Pts',(-0.748582462954855,-1.,1.73550351679848));
#31047=CARTESIAN_POINT('Ctrl Pts',(-0.748582462954855,1.,1.73550351679848));
#31048=CARTESIAN_POINT('Ctrl Pts',(-0.75019343597954,-1.,1.74080458266705));
#31049=CARTESIAN_POINT('Ctrl Pts',(-0.75019343597954,1.,1.74080458266705));
#31050=CARTESIAN_POINT('Ctrl Pts',(-0.751555614163629,-1.,1.74585086852298));
#31051=CARTESIAN_POINT('Ctrl Pts',(-0.751555614163629,1.,1.74585086852298));
#31052=CARTESIAN_POINT('Ctrl Pts',(-0.752797683531377,-1.,1.75095139468809));
#31053=CARTESIAN_POINT('Ctrl Pts',(-0.752797683531377,1.,1.75095139468809));
#31054=CARTESIAN_POINT('Ctrl Pts',(-0.75400925402848,-1.,1.75631083600175));
#31055=CARTESIAN_POINT('Ctrl Pts',(-0.75400925402848,1.,1.75631083600175));
#31056=CARTESIAN_POINT('Ctrl Pts',(-0.755220979975262,-1.,1.7619781724032));
#31057=CARTESIAN_POINT('Ctrl Pts',(-0.755220979975262,1.,1.7619781724032));
#31058=CARTESIAN_POINT('Ctrl Pts',(-0.756421896028403,-1.,1.76789396003141));
#31059=CARTESIAN_POINT('Ctrl Pts',(-0.756421896028403,1.,1.76789396003141));
#31060=CARTESIAN_POINT('Ctrl Pts',(-0.757578264077238,-1.,1.77394167108342));
#31061=CARTESIAN_POINT('Ctrl Pts',(-0.757578264077238,1.,1.77394167108342));
#31062=CARTESIAN_POINT('Ctrl Pts',(-0.75865062667738,-1.,1.77999411220912));
#31063=CARTESIAN_POINT('Ctrl Pts',(-0.75865062667738,1.,1.77999411220912));
#31064=CARTESIAN_POINT('Ctrl Pts',(-0.759614401109868,-1.,1.78596964884526));
#31065=CARTESIAN_POINT('Ctrl Pts',(-0.759614401109868,1.,1.78596964884526));
#31066=CARTESIAN_POINT('Ctrl Pts',(-0.760469555880425,-1.,1.79185815610802));
#31067=CARTESIAN_POINT('Ctrl Pts',(-0.760469555880425,1.,1.79185815610802));
#31068=CARTESIAN_POINT('Ctrl Pts',(-0.761229695230359,-1.,1.79768986997735));
#31069=CARTESIAN_POINT('Ctrl Pts',(-0.761229695230359,1.,1.79768986997735));
#31070=CARTESIAN_POINT('Ctrl Pts',(-0.761915336443516,-1.,1.80351583877334));
#31071=CARTESIAN_POINT('Ctrl Pts',(-0.761915336443516,1.,1.80351583877334));
#31072=CARTESIAN_POINT('Ctrl Pts',(-0.762546129464036,-1.,1.80938551463989));
#31073=CARTESIAN_POINT('Ctrl Pts',(-0.762546129464036,1.,1.80938551463989));
#31074=CARTESIAN_POINT('Ctrl Pts',(-0.763132003836783,-1.,1.81532118405566));
#31075=CARTESIAN_POINT('Ctrl Pts',(-0.763132003836783,1.,1.81532118405566));
#31076=CARTESIAN_POINT('Ctrl Pts',(-0.763673465462854,-1.,1.82131873145297));
#31077=CARTESIAN_POINT('Ctrl Pts',(-0.763673465462854,1.,1.82131873145297));
#31078=CARTESIAN_POINT('Ctrl Pts',(-0.764165902606055,-1.,1.8273599120008));
#31079=CARTESIAN_POINT('Ctrl Pts',(-0.764165902606055,1.,1.8273599120008));
#31080=CARTESIAN_POINT('Ctrl Pts',(-0.764602549687845,-1.,1.8334207722714));
#31081=CARTESIAN_POINT('Ctrl Pts',(-0.764602549687845,1.,1.8334207722714));
#31082=CARTESIAN_POINT('Ctrl Pts',(-0.764978057881687,-1.,1.83948181064823));
#31083=CARTESIAN_POINT('Ctrl Pts',(-0.764978057881687,1.,1.83948181064823));
#31084=CARTESIAN_POINT('Ctrl Pts',(-0.765291664861971,-1.,1.8455369887591));
#31085=CARTESIAN_POINT('Ctrl Pts',(-0.765291664861971,1.,1.8455369887591));
#31086=CARTESIAN_POINT('Ctrl Pts',(-0.765545710619023,-1.,1.85158945130054));
#31087=CARTESIAN_POINT('Ctrl Pts',(-0.765545710619023,1.,1.85158945130054));
#31088=CARTESIAN_POINT('Ctrl Pts',(-0.765744212909305,-1.,1.85764741390391));
#31089=CARTESIAN_POINT('Ctrl Pts',(-0.765744212909305,1.,1.85764741390391));
#31090=CARTESIAN_POINT('Ctrl Pts',(-0.765891519092557,-1.,1.86372027063314));
#31091=CARTESIAN_POINT('Ctrl Pts',(-0.765891519092557,1.,1.86372027063314));
#31092=CARTESIAN_POINT('Ctrl Pts',(-0.765990708546111,-1.,1.86981398314345));
#31093=CARTESIAN_POINT('Ctrl Pts',(-0.765990708546111,1.,1.86981398314345));
#31094=CARTESIAN_POINT('Ctrl Pts',(-0.766042837036759,-1.,1.87592888967886));
#31095=CARTESIAN_POINT('Ctrl Pts',(-0.766042837036759,1.,1.87592888967886));
#31096=CARTESIAN_POINT('Ctrl Pts',(-0.766047794851869,-1.,1.88206215302561));
#31097=CARTESIAN_POINT('Ctrl Pts',(-0.766047794851869,1.,1.88206215302561));
#31098=CARTESIAN_POINT('Ctrl Pts',(-0.76600483706209,-1.,1.88820926433409));
#31099=CARTESIAN_POINT('Ctrl Pts',(-0.76600483706209,1.,1.88820926433409));
#31100=CARTESIAN_POINT('Ctrl Pts',(-0.765913193856979,-1.,1.89436577771389));
#31101=CARTESIAN_POINT('Ctrl Pts',(-0.765913193856979,1.,1.89436577771389));
#31102=CARTESIAN_POINT('Ctrl Pts',(-0.765772772593395,-1.,1.90052930393599));
#31103=CARTESIAN_POINT('Ctrl Pts',(-0.765772772593395,1.,1.90052930393599));
#31104=CARTESIAN_POINT('Ctrl Pts',(-0.765584196937936,-1.,1.90669961402362));
#31105=CARTESIAN_POINT('Ctrl Pts',(-0.765584196937936,1.,1.90669961402362));
#31106=CARTESIAN_POINT('Ctrl Pts',(-0.765348465884739,-1.,1.91287765805174));
#31107=CARTESIAN_POINT('Ctrl Pts',(-0.765348465884739,1.,1.91287765805174));
#31108=CARTESIAN_POINT('Ctrl Pts',(-0.765066729667095,-1.,1.91906491634197));
#31109=CARTESIAN_POINT('Ctrl Pts',(-0.765066729667095,1.,1.91906491634197));
#31110=CARTESIAN_POINT('Ctrl Pts',(-0.764740025488189,-1.,1.92526263537041));
#31111=CARTESIAN_POINT('Ctrl Pts',(-0.764740025488189,1.,1.92526263537041));
#31112=CARTESIAN_POINT('Ctrl Pts',(-0.764369010673889,-1.,1.93147105496367));
#31113=CARTESIAN_POINT('Ctrl Pts',(-0.764369010673889,1.,1.93147105496367));
#31114=CARTESIAN_POINT('Ctrl Pts',(-0.763954049121393,-1.,1.93768964875867));
#31115=CARTESIAN_POINT('Ctrl Pts',(-0.763954049121393,1.,1.93768964875867));
#31116=CARTESIAN_POINT('Ctrl Pts',(-0.76349533353858,-1.,1.94391746617626));
#31117=CARTESIAN_POINT('Ctrl Pts',(-0.76349533353858,1.,1.94391746617626));
#31118=CARTESIAN_POINT('Ctrl Pts',(-0.762992990878774,-1.,1.95015342590025));
#31119=CARTESIAN_POINT('Ctrl Pts',(-0.762992990878774,1.,1.95015342590025));
#31120=CARTESIAN_POINT('Ctrl Pts',(-0.762447203806263,-1.,1.95639665309893));
#31121=CARTESIAN_POINT('Ctrl Pts',(-0.762447203806263,1.,1.95639665309893));
#31122=CARTESIAN_POINT('Ctrl Pts',(-0.761858300014575,-1.,1.96264672744229));
#31123=CARTESIAN_POINT('Ctrl Pts',(-0.761858300014575,1.,1.96264672744229));
#31124=CARTESIAN_POINT('Ctrl Pts',(-0.761226690483986,-1.,1.96890351582545));
#31125=CARTESIAN_POINT('Ctrl Pts',(-0.761226690483986,1.,1.96890351582545));
#31126=CARTESIAN_POINT('Ctrl Pts',(-0.760552825409855,-1.,1.97516705321521));
#31127=CARTESIAN_POINT('Ctrl Pts',(-0.760552825409855,1.,1.97516705321521));
#31128=CARTESIAN_POINT('Ctrl Pts',(-0.759837147452135,-1.,1.98143741418156));
#31129=CARTESIAN_POINT('Ctrl Pts',(-0.759837147452135,1.,1.98143741418156));
#31130=CARTESIAN_POINT('Ctrl Pts',(-0.759080037802243,-1.,1.98771456680806));
#31131=CARTESIAN_POINT('Ctrl Pts',(-0.759080037802243,1.,1.98771456680806));
#31132=CARTESIAN_POINT('Ctrl Pts',(-0.758281796766377,-1.,1.9939983109871));
#31133=CARTESIAN_POINT('Ctrl Pts',(-0.758281796766377,1.,1.9939983109871));
#31134=CARTESIAN_POINT('Ctrl Pts',(-0.757442676862341,-1.,2.00028834739072));
#31135=CARTESIAN_POINT('Ctrl Pts',(-0.757442676862341,1.,2.00028834739072));
#31136=CARTESIAN_POINT('Ctrl Pts',(-0.756562904646496,-1.,2.00658431587682));
#31137=CARTESIAN_POINT('Ctrl Pts',(-0.756562904646496,1.,2.00658431587682));
#31138=CARTESIAN_POINT('Ctrl Pts',(-0.7556427049581,-1.,2.01288584328149));
#31139=CARTESIAN_POINT('Ctrl Pts',(-0.7556427049581,1.,2.01288584328149));
#31140=CARTESIAN_POINT('Ctrl Pts',(-0.75468233072352,-1.,2.01919259406003));
#31141=CARTESIAN_POINT('Ctrl Pts',(-0.75468233072352,1.,2.01919259406003));
#31142=CARTESIAN_POINT('Ctrl Pts',(-0.753682061113766,-1.,2.02550428623587));
#31143=CARTESIAN_POINT('Ctrl Pts',(-0.753682061113766,1.,2.02550428623587));
#31144=CARTESIAN_POINT('Ctrl Pts',(-0.752642180488104,-1.,2.03182068456467));
#31145=CARTESIAN_POINT('Ctrl Pts',(-0.752642180488104,1.,2.03182068456467));
#31146=CARTESIAN_POINT('Ctrl Pts',(-0.751562963361384,-1.,2.03814160092173));
#31147=CARTESIAN_POINT('Ctrl Pts',(-0.751562963361384,1.,2.03814160092173));
#31148=CARTESIAN_POINT('Ctrl Pts',(-0.750444657874758,-1.,2.04446689147754));
#31149=CARTESIAN_POINT('Ctrl Pts',(-0.750444657874758,1.,2.04446689147754));
#31150=CARTESIAN_POINT('Ctrl Pts',(-0.749287468663053,-1.,2.05079645591606));
#31151=CARTESIAN_POINT('Ctrl Pts',(-0.749287468663053,1.,2.05079645591606));
#31152=CARTESIAN_POINT('Ctrl Pts',(-0.748091554181101,-1.,2.05713023030263));
#31153=CARTESIAN_POINT('Ctrl Pts',(-0.748091554181101,1.,2.05713023030263));
#31154=CARTESIAN_POINT('Ctrl Pts',(-0.747103932785504,-1.,2.06220058927162));
#31155=CARTESIAN_POINT('Ctrl Pts',(-0.747103932785504,1.,2.06220058927162));
#31156=CARTESIAN_POINT('Ctrl Pts',(-0.746345871542696,-1.,2.06600523016401));
#31157=CARTESIAN_POINT('Ctrl Pts',(-0.746345871542696,1.,2.06600523016401));
#31158=CARTESIAN_POINT('Ctrl Pts',(-0.74583279137781,-1.,2.06854248895575));
#31159=CARTESIAN_POINT('Ctrl Pts',(-0.74583279137781,1.,2.06854248895575));
#31160=CARTESIAN_POINT('Ctrl Pts',(-0.745574324794401,-1.,2.0698113262342));
#31161=CARTESIAN_POINT('Ctrl Pts',(-0.745574324794401,1.,2.0698113262342));
#31162=CARTESIAN_POINT('',(-0.693717979106306,1.,1.60662857109684));
#31163=CARTESIAN_POINT('Ctrl Pts',(-0.693717979106306,1.,1.60662857109684));
#31164=CARTESIAN_POINT('Ctrl Pts',(-0.695712097881194,1.,1.61106790958151));
#31165=CARTESIAN_POINT('Ctrl Pts',(-0.699605146405088,1.,1.61974673472612));
#31166=CARTESIAN_POINT('Ctrl Pts',(-0.705159151988319,1.,1.63216541664676));
#31167=CARTESIAN_POINT('Ctrl Pts',(-0.711993139355394,1.,1.64752408832016));
#31168=CARTESIAN_POINT('Ctrl Pts',(-0.719585433804282,1.,1.6647288055568));
#31169=CARTESIAN_POINT('Ctrl Pts',(-0.726235967997433,1.,1.67996158455503));
#31170=CARTESIAN_POINT('Ctrl Pts',(-0.731963238697195,1.,1.69326921975743));
#31171=CARTESIAN_POINT('Ctrl Pts',(-0.736799665724771,1.,1.70473309006121));
#31172=CARTESIAN_POINT('Ctrl Pts',(-0.740795162032088,1.,1.71447789751927));
#31173=CARTESIAN_POINT('Ctrl Pts',(-0.744021445433764,1.,1.7226822991693));
#31174=CARTESIAN_POINT('Ctrl Pts',(-0.746574710096436,1.,1.72958533647399));
#31175=CARTESIAN_POINT('Ctrl Pts',(-0.748582462954855,1.,1.73550351679848));
#31176=CARTESIAN_POINT('Ctrl Pts',(-0.75019343597954,1.,1.74080458266705));
#31177=CARTESIAN_POINT('Ctrl Pts',(-0.751555614163629,1.,1.74585086852298));
#31178=CARTESIAN_POINT('Ctrl Pts',(-0.752797683531377,1.,1.75095139468809));
#31179=CARTESIAN_POINT('Ctrl Pts',(-0.75400925402848,1.,1.75631083600175));
#31180=CARTESIAN_POINT('Ctrl Pts',(-0.755220979975262,1.,1.7619781724032));
#31181=CARTESIAN_POINT('Ctrl Pts',(-0.756421896028403,1.,1.76789396003141));
#31182=CARTESIAN_POINT('Ctrl Pts',(-0.757578264077238,1.,1.77394167108342));
#31183=CARTESIAN_POINT('Ctrl Pts',(-0.75865062667738,1.,1.77999411220912));
#31184=CARTESIAN_POINT('Ctrl Pts',(-0.759614401109868,1.,1.78596964884526));
#31185=CARTESIAN_POINT('Ctrl Pts',(-0.760469555880425,1.,1.79185815610802));
#31186=CARTESIAN_POINT('Ctrl Pts',(-0.761229695230359,1.,1.79768986997735));
#31187=CARTESIAN_POINT('Ctrl Pts',(-0.761915336443516,1.,1.80351583877334));
#31188=CARTESIAN_POINT('Ctrl Pts',(-0.762546129464036,1.,1.80938551463989));
#31189=CARTESIAN_POINT('Ctrl Pts',(-0.763132003836783,1.,1.81532118405566));
#31190=CARTESIAN_POINT('Ctrl Pts',(-0.763673465462854,1.,1.82131873145297));
#31191=CARTESIAN_POINT('Ctrl Pts',(-0.764165902606055,1.,1.8273599120008));
#31192=CARTESIAN_POINT('Ctrl Pts',(-0.764602549687845,1.,1.8334207722714));
#31193=CARTESIAN_POINT('Ctrl Pts',(-0.764978057881687,1.,1.83948181064823));
#31194=CARTESIAN_POINT('Ctrl Pts',(-0.765291664861971,1.,1.8455369887591));
#31195=CARTESIAN_POINT('Ctrl Pts',(-0.765545710619023,1.,1.85158945130054));
#31196=CARTESIAN_POINT('Ctrl Pts',(-0.765744212909305,1.,1.85764741390391));
#31197=CARTESIAN_POINT('Ctrl Pts',(-0.765891519092557,1.,1.86372027063314));
#31198=CARTESIAN_POINT('Ctrl Pts',(-0.765990708546111,1.,1.86981398314345));
#31199=CARTESIAN_POINT('Ctrl Pts',(-0.766042837036759,1.,1.87592888967886));
#31200=CARTESIAN_POINT('Ctrl Pts',(-0.766047794851869,1.,1.88206215302561));
#31201=CARTESIAN_POINT('Ctrl Pts',(-0.76600483706209,1.,1.88820926433409));
#31202=CARTESIAN_POINT('Ctrl Pts',(-0.765913193856979,1.,1.89436577771389));
#31203=CARTESIAN_POINT('Ctrl Pts',(-0.765772772593395,1.,1.90052930393599));
#31204=CARTESIAN_POINT('Ctrl Pts',(-0.765584196937936,1.,1.90669961402362));
#31205=CARTESIAN_POINT('Ctrl Pts',(-0.765348465884739,1.,1.91287765805174));
#31206=CARTESIAN_POINT('Ctrl Pts',(-0.765066729667095,1.,1.91906491634197));
#31207=CARTESIAN_POINT('Ctrl Pts',(-0.764740025488189,1.,1.92526263537041));
#31208=CARTESIAN_POINT('Ctrl Pts',(-0.764369010673889,1.,1.93147105496367));
#31209=CARTESIAN_POINT('Ctrl Pts',(-0.763954049121393,1.,1.93768964875867));
#31210=CARTESIAN_POINT('Ctrl Pts',(-0.76349533353858,1.,1.94391746617626));
#31211=CARTESIAN_POINT('Ctrl Pts',(-0.762992990878774,1.,1.95015342590025));
#31212=CARTESIAN_POINT('Ctrl Pts',(-0.762447203806263,1.,1.95639665309893));
#31213=CARTESIAN_POINT('Ctrl Pts',(-0.761858300014575,1.,1.96264672744229));
#31214=CARTESIAN_POINT('Ctrl Pts',(-0.761226690483986,1.,1.96890351582545));
#31215=CARTESIAN_POINT('Ctrl Pts',(-0.760552825409855,1.,1.97516705321521));
#31216=CARTESIAN_POINT('Ctrl Pts',(-0.759837147452135,1.,1.98143741418156));
#31217=CARTESIAN_POINT('Ctrl Pts',(-0.759080037802243,1.,1.98771456680806));
#31218=CARTESIAN_POINT('Ctrl Pts',(-0.758281796766377,1.,1.9939983109871));
#31219=CARTESIAN_POINT('Ctrl Pts',(-0.757442676862341,1.,2.00028834739072));
#31220=CARTESIAN_POINT('Ctrl Pts',(-0.756562904646496,1.,2.00658431587682));
#31221=CARTESIAN_POINT('Ctrl Pts',(-0.7556427049581,1.,2.01288584328149));
#31222=CARTESIAN_POINT('Ctrl Pts',(-0.75468233072352,1.,2.01919259406003));
#31223=CARTESIAN_POINT('Ctrl Pts',(-0.753682061113766,1.,2.02550428623587));
#31224=CARTESIAN_POINT('Ctrl Pts',(-0.752642180488104,1.,2.03182068456467));
#31225=CARTESIAN_POINT('Ctrl Pts',(-0.751562963361384,1.,2.03814160092173));
#31226=CARTESIAN_POINT('Ctrl Pts',(-0.750444657874758,1.,2.04446689147754));
#31227=CARTESIAN_POINT('Ctrl Pts',(-0.749287468663053,1.,2.05079645591606));
#31228=CARTESIAN_POINT('Ctrl Pts',(-0.748091554181101,1.,2.05713023030263));
#31229=CARTESIAN_POINT('Ctrl Pts',(-0.747103932785504,1.,2.06220058927162));
#31230=CARTESIAN_POINT('Ctrl Pts',(-0.746345871542696,1.,2.06600523016401));
#31231=CARTESIAN_POINT('Ctrl Pts',(-0.74583279137781,1.,2.06854248895575));
#31232=CARTESIAN_POINT('Ctrl Pts',(-0.745574324794401,1.,2.0698113262342));
#31233=CARTESIAN_POINT('',(-0.693717979106306,0.,1.60662857109684));
#31234=CARTESIAN_POINT('Origin',(0.,0.,0.));
#31235=CARTESIAN_POINT('',(-0.892032620296855,1.,1.5055822144029));
#31236=CARTESIAN_POINT('Origin',(0.,1.,0.));
#31237=CARTESIAN_POINT('',(-0.892032620296855,0.,1.5055822144029));
#31238=CARTESIAN_POINT('Ctrl Pts',(-1.23627494547115,-1.,1.81978687191668));
#31239=CARTESIAN_POINT('Ctrl Pts',(-1.23627494547115,1.,1.81978687191668));
#31240=CARTESIAN_POINT('Ctrl Pts',(-1.23509651170476,-1.,1.81925017193666));
#31241=CARTESIAN_POINT('Ctrl Pts',(-1.23509651170476,1.,1.81925017193666));
#31242=CARTESIAN_POINT('Ctrl Pts',(-1.2327422452705,-1.,1.81817389921279));
#31243=CARTESIAN_POINT('Ctrl Pts',(-1.2327422452705,1.,1.81817389921279));
#31244=CARTESIAN_POINT('Ctrl Pts',(-1.2292186489137,-1.,1.8165508718364));
#31245=CARTESIAN_POINT('Ctrl Pts',(-1.2292186489137,1.,1.8165508718364));
#31246=CARTESIAN_POINT('Ctrl Pts',(-1.2245361330495,-1.,1.81436959210434));
#31247=CARTESIAN_POINT('Ctrl Pts',(-1.2245361330495,1.,1.81436959210434));
#31248=CARTESIAN_POINT('Ctrl Pts',(-1.21870906103557,-1.,1.81161420806656));
#31249=CARTESIAN_POINT('Ctrl Pts',(-1.21870906103557,1.,1.81161420806656));
#31250=CARTESIAN_POINT('Ctrl Pts',(-1.21290815708314,-1.,1.80882996917129));
#31251=CARTESIAN_POINT('Ctrl Pts',(-1.21290815708314,1.,1.80882996917129));
#31252=CARTESIAN_POINT('Ctrl Pts',(-1.20713356605475,-1.,1.80601678480707));
#31253=CARTESIAN_POINT('Ctrl Pts',(-1.20713356605475,1.,1.80601678480707));
#31254=CARTESIAN_POINT('Ctrl Pts',(-1.20138548938974,-1.,1.80317454838603));
#31255=CARTESIAN_POINT('Ctrl Pts',(-1.20138548938974,1.,1.80317454838603));
#31256=CARTESIAN_POINT('Ctrl Pts',(-1.19566418930242,-1.,1.80030314369879));
#31257=CARTESIAN_POINT('Ctrl Pts',(-1.19566418930242,1.,1.80030314369879));
#31258=CARTESIAN_POINT('Ctrl Pts',(-1.18996997934445,-1.,1.79740245923478));
#31259=CARTESIAN_POINT('Ctrl Pts',(-1.18996997934445,1.,1.79740245923478));
#31260=CARTESIAN_POINT('Ctrl Pts',(-1.18430321697432,-1.,1.79447240321515));
#31261=CARTESIAN_POINT('Ctrl Pts',(-1.18430321697432,1.,1.79447240321515));
#31262=CARTESIAN_POINT('Ctrl Pts',(-1.17866429440809,-1.,1.79151291552689));
#31263=CARTESIAN_POINT('Ctrl Pts',(-1.17866429440809,1.,1.79151291552689));
#31264=CARTESIAN_POINT('Ctrl Pts',(-1.17305363177328,-1.,1.78852398877616));
#31265=CARTESIAN_POINT('Ctrl Pts',(-1.17305363177328,1.,1.78852398877616));
#31266=CARTESIAN_POINT('Ctrl Pts',(-1.16747166312303,-1.,1.78550566040443));
#31267=CARTESIAN_POINT('Ctrl Pts',(-1.16747166312303,1.,1.78550566040443));
#31268=CARTESIAN_POINT('Ctrl Pts',(-1.16191881298499,-1.,1.78245795881009));
#31269=CARTESIAN_POINT('Ctrl Pts',(-1.16191881298499,1.,1.78245795881009));
#31270=CARTESIAN_POINT('Ctrl Pts',(-1.15639547194698,-1.,1.77938085564275));
#31271=CARTESIAN_POINT('Ctrl Pts',(-1.15639547194698,1.,1.77938085564275));
#31272=CARTESIAN_POINT('Ctrl Pts',(-1.15090197841515,-1.,1.7762742255701));
#31273=CARTESIAN_POINT('Ctrl Pts',(-1.15090197841515,1.,1.7762742255701));
#31274=CARTESIAN_POINT('Ctrl Pts',(-1.1454385822692,-1.,1.77313777896194));
#31275=CARTESIAN_POINT('Ctrl Pts',(-1.1454385822692,1.,1.77313777896194));
#31276=CARTESIAN_POINT('Ctrl Pts',(-1.14000548336975,-1.,1.76997111386769));
#31277=CARTESIAN_POINT('Ctrl Pts',(-1.14000548336975,1.,1.76997111386769));
#31278=CARTESIAN_POINT('Ctrl Pts',(-1.1346029180462,-1.,1.76677384551862));
#31279=CARTESIAN_POINT('Ctrl Pts',(-1.1346029180462,1.,1.76677384551862));
#31280=CARTESIAN_POINT('Ctrl Pts',(-1.12923123555075,-1.,1.7635457196617));
#31281=CARTESIAN_POINT('Ctrl Pts',(-1.12923123555075,1.,1.7635457196617));
#31282=CARTESIAN_POINT('Ctrl Pts',(-1.12389096855086,-1.,1.76028671825096));
#31283=CARTESIAN_POINT('Ctrl Pts',(-1.12389096855086,1.,1.76028671825096));
#31284=CARTESIAN_POINT('Ctrl Pts',(-1.11858293216763,-1.,1.75699720772105));
#31285=CARTESIAN_POINT('Ctrl Pts',(-1.11858293216763,1.,1.75699720772105));
#31286=CARTESIAN_POINT('Ctrl Pts',(-1.11330807582551,-1.,1.7536777209463));
#31287=CARTESIAN_POINT('Ctrl Pts',(-1.11330807582551,1.,1.7536777209463));
#31288=CARTESIAN_POINT('Ctrl Pts',(-1.10806728183007,-1.,1.7503286607592));
#31289=CARTESIAN_POINT('Ctrl Pts',(-1.10806728183007,1.,1.7503286607592));
#31290=CARTESIAN_POINT('Ctrl Pts',(-1.10286118991143,-1.,1.74695004214923));
#31291=CARTESIAN_POINT('Ctrl Pts',(-1.10286118991143,1.,1.74695004214923));
#31292=CARTESIAN_POINT('Ctrl Pts',(-1.09768999241225,-1.,1.74354119236208));
#31293=CARTESIAN_POINT('Ctrl Pts',(-1.09768999241225,1.,1.74354119236208));
#31294=CARTESIAN_POINT('Ctrl Pts',(-1.09255329056493,-1.,1.74010053962247));
#31295=CARTESIAN_POINT('Ctrl Pts',(-1.09255329056493,1.,1.74010053962247));
#31296=CARTESIAN_POINT('Ctrl Pts',(-1.08745056285427,-1.,1.73662628326091));
#31297=CARTESIAN_POINT('Ctrl Pts',(-1.08745056285427,1.,1.73662628326091));
#31298=CARTESIAN_POINT('Ctrl Pts',(-1.08238162784749,-1.,1.73311705663407));
#31299=CARTESIAN_POINT('Ctrl Pts',(-1.08238162784749,1.,1.73311705663407));
#31300=CARTESIAN_POINT('Ctrl Pts',(-1.0773470373727,-1.,1.72957248977424));
#31301=CARTESIAN_POINT('Ctrl Pts',(-1.0773470373727,1.,1.72957248977424));
#31302=CARTESIAN_POINT('Ctrl Pts',(-1.07234866990252,-1.,1.72599406198488));
#31303=CARTESIAN_POINT('Ctrl Pts',(-1.07234866990252,1.,1.72599406198488));
#31304=CARTESIAN_POINT('Ctrl Pts',(-1.06738966975462,-1.,1.72238500928453));
#31305=CARTESIAN_POINT('Ctrl Pts',(-1.06738966975462,1.,1.72238500928453));
#31306=CARTESIAN_POINT('Ctrl Pts',(-1.06247324680647,-1.,1.71874858456904));
#31307=CARTESIAN_POINT('Ctrl Pts',(-1.06247324680647,1.,1.71874858456904));
#31308=CARTESIAN_POINT('Ctrl Pts',(-1.05760163192479,-1.,1.7150865442702));
#31309=CARTESIAN_POINT('Ctrl Pts',(-1.05760163192479,1.,1.7150865442702));
#31310=CARTESIAN_POINT('Ctrl Pts',(-1.05277517202855,-1.,1.71139783543989));
#31311=CARTESIAN_POINT('Ctrl Pts',(-1.05277517202855,1.,1.71139783543989));
#31312=CARTESIAN_POINT('Ctrl Pts',(-1.04799085404995,-1.,1.70767646263649));
#31313=CARTESIAN_POINT('Ctrl Pts',(-1.04799085404995,1.,1.70767646263649));
#31314=CARTESIAN_POINT('Ctrl Pts',(-1.04324363334554,-1.,1.70391338707982));
#31315=CARTESIAN_POINT('Ctrl Pts',(-1.04324363334554,1.,1.70391338707982));
#31316=CARTESIAN_POINT('Ctrl Pts',(-1.03852922490789,-1.,1.70010052930962));
#31317=CARTESIAN_POINT('Ctrl Pts',(-1.03852922490789,1.,1.70010052930962));
#31318=CARTESIAN_POINT('Ctrl Pts',(-1.03384646003588,-1.,1.69623414782771));
#31319=CARTESIAN_POINT('Ctrl Pts',(-1.03384646003588,1.,1.69623414782771));
#31320=CARTESIAN_POINT('Ctrl Pts',(-1.02919977579147,-1.,1.69231840863458));
#31321=CARTESIAN_POINT('Ctrl Pts',(-1.02919977579147,1.,1.69231840863458));
#31322=CARTESIAN_POINT('Ctrl Pts',(-1.02460180535255,-1.,1.68836910178447));
#31323=CARTESIAN_POINT('Ctrl Pts',(-1.02460180535255,1.,1.68836910178447));
#31324=CARTESIAN_POINT('Ctrl Pts',(-1.02006795074201,-1.,1.68440578021706));
#31325=CARTESIAN_POINT('Ctrl Pts',(-1.02006795074201,1.,1.68440578021706));
#31326=CARTESIAN_POINT('Ctrl Pts',(-1.01561026162773,-1.,1.68044289894798));
#31327=CARTESIAN_POINT('Ctrl Pts',(-1.01561026162773,1.,1.68044289894798));
#31328=CARTESIAN_POINT('Ctrl Pts',(-1.01123236493511,-1.,1.67648246776464));
#31329=CARTESIAN_POINT('Ctrl Pts',(-1.01123236493511,1.,1.67648246776464));
#31330=CARTESIAN_POINT('Ctrl Pts',(-1.00692206696414,-1.,1.67250335383293));
#31331=CARTESIAN_POINT('Ctrl Pts',(-1.00692206696414,1.,1.67250335383293));
#31332=CARTESIAN_POINT('Ctrl Pts',(-1.00265091003727,-1.,1.66846059277303));
#31333=CARTESIAN_POINT('Ctrl Pts',(-1.00265091003727,1.,1.66846059277303));
#31334=CARTESIAN_POINT('Ctrl Pts',(-0.998389654952758,-1.,1.66430758030376));
#31335=CARTESIAN_POINT('Ctrl Pts',(-0.998389654952758,1.,1.66430758030376));
#31336=CARTESIAN_POINT('Ctrl Pts',(-0.994121836661306,-1.,1.66001553809947));
#31337=CARTESIAN_POINT('Ctrl Pts',(-0.994121836661306,1.,1.66001553809947));
#31338=CARTESIAN_POINT('Ctrl Pts',(-0.989855627854165,-1.,1.65559044289699));
#31339=CARTESIAN_POINT('Ctrl Pts',(-0.989855627854165,1.,1.65559044289699));
#31340=CARTESIAN_POINT('Ctrl Pts',(-0.985642622920821,-1.,1.65110016612638));
#31341=CARTESIAN_POINT('Ctrl Pts',(-0.985642622920821,1.,1.65110016612638));
#31342=CARTESIAN_POINT('Ctrl Pts',(-0.981562530939489,-1.,1.64665139190656));
#31343=CARTESIAN_POINT('Ctrl Pts',(-0.981562530939489,1.,1.64665139190656));
#31344=CARTESIAN_POINT('Ctrl Pts',(-0.977689794119416,-1.,1.64233990826687));
#31345=CARTESIAN_POINT('Ctrl Pts',(-0.977689794119416,1.,1.64233990826687));
#31346=CARTESIAN_POINT('Ctrl Pts',(-0.974066058287418,-1.,1.63820952658144));
#31347=CARTESIAN_POINT('Ctrl Pts',(-0.974066058287418,1.,1.63820952658144));
#31348=CARTESIAN_POINT('Ctrl Pts',(-0.970669715997509,-1.,1.63420665729798));
#31349=CARTESIAN_POINT('Ctrl Pts',(-0.970669715997509,1.,1.63420665729798));
#31350=CARTESIAN_POINT('Ctrl Pts',(-0.967387853230345,-1.,1.63013849959461));
#31351=CARTESIAN_POINT('Ctrl Pts',(-0.967387853230345,1.,1.63013849959461));
#31352=CARTESIAN_POINT('Ctrl Pts',(-0.964046107040536,-1.,1.62571930670187));
#31353=CARTESIAN_POINT('Ctrl Pts',(-0.964046107040536,1.,1.62571930670187));
#31354=CARTESIAN_POINT('Ctrl Pts',(-0.960438326101729,-1.,1.62061638140221));
#31355=CARTESIAN_POINT('Ctrl Pts',(-0.960438326101729,1.,1.62061638140221));
#31356=CARTESIAN_POINT('Ctrl Pts',(-0.956354422920671,-1.,1.61449324337085));
#31357=CARTESIAN_POINT('Ctrl Pts',(-0.956354422920671,1.,1.61449324337085));
#31358=CARTESIAN_POINT('Ctrl Pts',(-0.951613284356035,-1.,1.60706069896936));
#31359=CARTESIAN_POINT('Ctrl Pts',(-0.951613284356035,1.,1.60706069896936));
#31360=CARTESIAN_POINT('Ctrl Pts',(-0.946078063315257,-1.,1.59810042043673));
#31361=CARTESIAN_POINT('Ctrl Pts',(-0.946078063315257,1.,1.59810042043673));
#31362=CARTESIAN_POINT('Ctrl Pts',(-0.939646377893399,-1.,1.58744937487176));
#31363=CARTESIAN_POINT('Ctrl Pts',(-0.939646377893399,1.,1.58744937487176));
#31364=CARTESIAN_POINT('Ctrl Pts',(-0.932246680108685,-1.,1.57499388382243));
#31365=CARTESIAN_POINT('Ctrl Pts',(-0.932246680108685,1.,1.57499388382243));
#31366=CARTESIAN_POINT('Ctrl Pts',(-0.923832188944341,-1.,1.56065988578893));
#31367=CARTESIAN_POINT('Ctrl Pts',(-0.923832188944341,1.,1.56065988578893));
#31368=CARTESIAN_POINT('Ctrl Pts',(-0.914375919026456,-1.,1.54440491149498));
#31369=CARTESIAN_POINT('Ctrl Pts',(-0.914375919026456,1.,1.54440491149498));
#31370=CARTESIAN_POINT('Ctrl Pts',(-0.905967409625651,-1.,1.52984849887993));
#31371=CARTESIAN_POINT('Ctrl Pts',(-0.905967409625651,1.,1.52984849887993));
#31372=CARTESIAN_POINT('Ctrl Pts',(-0.899185047483511,-1.,1.51805569590094));
#31373=CARTESIAN_POINT('Ctrl Pts',(-0.899185047483511,1.,1.51805569590094));
#31374=CARTESIAN_POINT('Ctrl Pts',(-0.894452006964543,-1.,1.50980486806688));
#31375=CARTESIAN_POINT('Ctrl Pts',(-0.894452006964543,1.,1.50980486806688));
#31376=CARTESIAN_POINT('Ctrl Pts',(-0.892032620296855,-1.,1.5055822144029));
#31377=CARTESIAN_POINT('Ctrl Pts',(-0.892032620296855,1.,1.5055822144029));
#31378=CARTESIAN_POINT('',(-1.23627494547115,1.,1.81978687191668));
#31379=CARTESIAN_POINT('Ctrl Pts',(-1.23627494547115,1.,1.81978687191668));
#31380=CARTESIAN_POINT('Ctrl Pts',(-1.23509651170476,1.,1.81925017193666));
#31381=CARTESIAN_POINT('Ctrl Pts',(-1.2327422452705,1.,1.81817389921279));
#31382=CARTESIAN_POINT('Ctrl Pts',(-1.2292186489137,1.,1.8165508718364));
#31383=CARTESIAN_POINT('Ctrl Pts',(-1.2245361330495,1.,1.81436959210434));
#31384=CARTESIAN_POINT('Ctrl Pts',(-1.21870906103557,1.,1.81161420806656));
#31385=CARTESIAN_POINT('Ctrl Pts',(-1.21290815708314,1.,1.80882996917129));
#31386=CARTESIAN_POINT('Ctrl Pts',(-1.20713356605475,1.,1.80601678480707));
#31387=CARTESIAN_POINT('Ctrl Pts',(-1.20138548938974,1.,1.80317454838603));
#31388=CARTESIAN_POINT('Ctrl Pts',(-1.19566418930242,1.,1.80030314369879));
#31389=CARTESIAN_POINT('Ctrl Pts',(-1.18996997934445,1.,1.79740245923478));
#31390=CARTESIAN_POINT('Ctrl Pts',(-1.18430321697432,1.,1.79447240321515));
#31391=CARTESIAN_POINT('Ctrl Pts',(-1.17866429440809,1.,1.79151291552689));
#31392=CARTESIAN_POINT('Ctrl Pts',(-1.17305363177328,1.,1.78852398877616));
#31393=CARTESIAN_POINT('Ctrl Pts',(-1.16747166312303,1.,1.78550566040443));
#31394=CARTESIAN_POINT('Ctrl Pts',(-1.16191881298499,1.,1.78245795881009));
#31395=CARTESIAN_POINT('Ctrl Pts',(-1.15639547194698,1.,1.77938085564275));
#31396=CARTESIAN_POINT('Ctrl Pts',(-1.15090197841515,1.,1.7762742255701));
#31397=CARTESIAN_POINT('Ctrl Pts',(-1.1454385822692,1.,1.77313777896194));
#31398=CARTESIAN_POINT('Ctrl Pts',(-1.14000548336975,1.,1.76997111386769));
#31399=CARTESIAN_POINT('Ctrl Pts',(-1.1346029180462,1.,1.76677384551862));
#31400=CARTESIAN_POINT('Ctrl Pts',(-1.12923123555075,1.,1.7635457196617));
#31401=CARTESIAN_POINT('Ctrl Pts',(-1.12389096855086,1.,1.76028671825096));
#31402=CARTESIAN_POINT('Ctrl Pts',(-1.11858293216763,1.,1.75699720772105));
#31403=CARTESIAN_POINT('Ctrl Pts',(-1.11330807582551,1.,1.7536777209463));
#31404=CARTESIAN_POINT('Ctrl Pts',(-1.10806728183007,1.,1.7503286607592));
#31405=CARTESIAN_POINT('Ctrl Pts',(-1.10286118991143,1.,1.74695004214923));
#31406=CARTESIAN_POINT('Ctrl Pts',(-1.09768999241225,1.,1.74354119236208));
#31407=CARTESIAN_POINT('Ctrl Pts',(-1.09255329056493,1.,1.74010053962247));
#31408=CARTESIAN_POINT('Ctrl Pts',(-1.08745056285427,1.,1.73662628326091));
#31409=CARTESIAN_POINT('Ctrl Pts',(-1.08238162784749,1.,1.73311705663407));
#31410=CARTESIAN_POINT('Ctrl Pts',(-1.0773470373727,1.,1.72957248977424));
#31411=CARTESIAN_POINT('Ctrl Pts',(-1.07234866990252,1.,1.72599406198488));
#31412=CARTESIAN_POINT('Ctrl Pts',(-1.06738966975462,1.,1.72238500928453));
#31413=CARTESIAN_POINT('Ctrl Pts',(-1.06247324680647,1.,1.71874858456904));
#31414=CARTESIAN_POINT('Ctrl Pts',(-1.05760163192479,1.,1.7150865442702));
#31415=CARTESIAN_POINT('Ctrl Pts',(-1.05277517202855,1.,1.71139783543989));
#31416=CARTESIAN_POINT('Ctrl Pts',(-1.04799085404995,1.,1.70767646263649));
#31417=CARTESIAN_POINT('Ctrl Pts',(-1.04324363334554,1.,1.70391338707982));
#31418=CARTESIAN_POINT('Ctrl Pts',(-1.03852922490789,1.,1.70010052930962));
#31419=CARTESIAN_POINT('Ctrl Pts',(-1.03384646003588,1.,1.69623414782771));
#31420=CARTESIAN_POINT('Ctrl Pts',(-1.02919977579147,1.,1.69231840863458));
#31421=CARTESIAN_POINT('Ctrl Pts',(-1.02460180535255,1.,1.68836910178447));
#31422=CARTESIAN_POINT('Ctrl Pts',(-1.02006795074201,1.,1.68440578021706));
#31423=CARTESIAN_POINT('Ctrl Pts',(-1.01561026162773,1.,1.68044289894798));
#31424=CARTESIAN_POINT('Ctrl Pts',(-1.01123236493511,1.,1.67648246776464));
#31425=CARTESIAN_POINT('Ctrl Pts',(-1.00692206696414,1.,1.67250335383293));
#31426=CARTESIAN_POINT('Ctrl Pts',(-1.00265091003727,1.,1.66846059277303));
#31427=CARTESIAN_POINT('Ctrl Pts',(-0.998389654952758,1.,1.66430758030376));
#31428=CARTESIAN_POINT('Ctrl Pts',(-0.994121836661306,1.,1.66001553809947));
#31429=CARTESIAN_POINT('Ctrl Pts',(-0.989855627854165,1.,1.65559044289699));
#31430=CARTESIAN_POINT('Ctrl Pts',(-0.985642622920821,1.,1.65110016612638));
#31431=CARTESIAN_POINT('Ctrl Pts',(-0.981562530939489,1.,1.64665139190656));
#31432=CARTESIAN_POINT('Ctrl Pts',(-0.977689794119416,1.,1.64233990826687));
#31433=CARTESIAN_POINT('Ctrl Pts',(-0.974066058287418,1.,1.63820952658144));
#31434=CARTESIAN_POINT('Ctrl Pts',(-0.970669715997509,1.,1.63420665729798));
#31435=CARTESIAN_POINT('Ctrl Pts',(-0.967387853230345,1.,1.63013849959461));
#31436=CARTESIAN_POINT('Ctrl Pts',(-0.964046107040536,1.,1.62571930670187));
#31437=CARTESIAN_POINT('Ctrl Pts',(-0.960438326101729,1.,1.62061638140221));
#31438=CARTESIAN_POINT('Ctrl Pts',(-0.956354422920671,1.,1.61449324337085));
#31439=CARTESIAN_POINT('Ctrl Pts',(-0.951613284356035,1.,1.60706069896936));
#31440=CARTESIAN_POINT('Ctrl Pts',(-0.946078063315257,1.,1.59810042043673));
#31441=CARTESIAN_POINT('Ctrl Pts',(-0.939646377893399,1.,1.58744937487176));
#31442=CARTESIAN_POINT('Ctrl Pts',(-0.932246680108685,1.,1.57499388382243));
#31443=CARTESIAN_POINT('Ctrl Pts',(-0.923832188944341,1.,1.56065988578893));
#31444=CARTESIAN_POINT('Ctrl Pts',(-0.914375919026456,1.,1.54440491149498));
#31445=CARTESIAN_POINT('Ctrl Pts',(-0.905967409625651,1.,1.52984849887993));
#31446=CARTESIAN_POINT('Ctrl Pts',(-0.899185047483511,1.,1.51805569590094));
#31447=CARTESIAN_POINT('Ctrl Pts',(-0.894452006964543,1.,1.50980486806688));
#31448=CARTESIAN_POINT('Ctrl Pts',(-0.892032620296855,1.,1.5055822144029));
#31449=CARTESIAN_POINT('',(-1.23627494547115,0.,1.81978687191668));
#31450=CARTESIAN_POINT('Origin',(-1.34869019493419,0.,1.73811241238545));
#31451=CARTESIAN_POINT('',(-1.34869019493419,1.,1.73811241238545));
#31452=CARTESIAN_POINT('',(-1.23627494547115,1.,1.81978687191668));
#31453=CARTESIAN_POINT('',(-1.34869019493419,0.,1.73811241238545));
#31454=CARTESIAN_POINT('Ctrl Pts',(-1.15624053661742,-1.,1.31362392696032));
#31455=CARTESIAN_POINT('Ctrl Pts',(-1.15624053661742,1.,1.31362392696032));
#31456=CARTESIAN_POINT('Ctrl Pts',(-1.15950888730809,-1.,1.31722977216397));
#31457=CARTESIAN_POINT('Ctrl Pts',(-1.15950888730809,1.,1.31722977216397));
#31458=CARTESIAN_POINT('Ctrl Pts',(-1.16589330093588,-1.,1.32428080721772));
#31459=CARTESIAN_POINT('Ctrl Pts',(-1.16589330093588,1.,1.32428080721772));
#31460=CARTESIAN_POINT('Ctrl Pts',(-1.17501305789857,-1.,1.33437539347008));
#31461=CARTESIAN_POINT('Ctrl Pts',(-1.17501305789857,1.,1.33437539347008));
#31462=CARTESIAN_POINT('Ctrl Pts',(-1.18625865667441,-1.,1.34687054001093));
#31463=CARTESIAN_POINT('Ctrl Pts',(-1.18625865667441,1.,1.34687054001093));
#31464=CARTESIAN_POINT('Ctrl Pts',(-1.1987959077932,-1.,1.36088705043885));
#31465=CARTESIAN_POINT('Ctrl Pts',(-1.1987959077932,1.,1.36088705043885));
#31466=CARTESIAN_POINT('Ctrl Pts',(-1.20982812925645,-1.,1.37331915607905));
#31467=CARTESIAN_POINT('Ctrl Pts',(-1.20982812925645,1.,1.37331915607905));
#31468=CARTESIAN_POINT('Ctrl Pts',(-1.21938737280852,-1.,1.38420564527715));
#31469=CARTESIAN_POINT('Ctrl Pts',(-1.21938737280852,1.,1.38420564527715));
#31470=CARTESIAN_POINT('Ctrl Pts',(-1.22752961899387,-1.,1.39361389568796));
#31471=CARTESIAN_POINT('Ctrl Pts',(-1.22752961899387,1.,1.39361389568796));
#31472=CARTESIAN_POINT('Ctrl Pts',(-1.23434087290423,-1.,1.40164708206106));
#31473=CARTESIAN_POINT('Ctrl Pts',(-1.23434087290423,1.,1.40164708206106));
#31474=CARTESIAN_POINT('Ctrl Pts',(-1.23994455029534,-1.,1.40845295531283));
#31475=CARTESIAN_POINT('Ctrl Pts',(-1.23994455029534,1.,1.40845295531283));
#31476=CARTESIAN_POINT('Ctrl Pts',(-1.24450600513056,-1.,1.41422913175179));
#31477=CARTESIAN_POINT('Ctrl Pts',(-1.24450600513056,1.,1.41422913175179));
#31478=CARTESIAN_POINT('Ctrl Pts',(-1.24824430986571,-1.,1.41923722596025));
#31479=CARTESIAN_POINT('Ctrl Pts',(-1.24824430986571,1.,1.41923722596025));
#31480=CARTESIAN_POINT('Ctrl Pts',(-1.2514145557001,-1.,1.42378102115575));
#31481=CARTESIAN_POINT('Ctrl Pts',(-1.2514145557001,1.,1.42378102115575));
#31482=CARTESIAN_POINT('Ctrl Pts',(-1.25426945222639,-1.,1.42815938799387));
#31483=CARTESIAN_POINT('Ctrl Pts',(-1.25426945222639,1.,1.42815938799387));
#31484=CARTESIAN_POINT('Ctrl Pts',(-1.25702687965755,-1.,1.43262645609691));
#31485=CARTESIAN_POINT('Ctrl Pts',(-1.25702687965755,1.,1.43262645609691));
#31486=CARTESIAN_POINT('Ctrl Pts',(-1.25983531012005,-1.,1.43734919180848));
#31487=CARTESIAN_POINT('Ctrl Pts',(-1.25983531012005,1.,1.43734919180848));
#31488=CARTESIAN_POINT('Ctrl Pts',(-1.26273903323859,-1.,1.44236470511303));
#31489=CARTESIAN_POINT('Ctrl Pts',(-1.26273903323859,1.,1.44236470511303));
#31490=CARTESIAN_POINT('Ctrl Pts',(-1.26570925118868,-1.,1.44761985001662));
#31491=CARTESIAN_POINT('Ctrl Pts',(-1.26570925118868,1.,1.44761985001662));
#31492=CARTESIAN_POINT('Ctrl Pts',(-1.2686778680489,-1.,1.45301422764247));
#31493=CARTESIAN_POINT('Ctrl Pts',(-1.2686778680489,1.,1.45301422764247));
#31494=CARTESIAN_POINT('Ctrl Pts',(-1.27156805265289,-1.,1.45843906294697));
#31495=CARTESIAN_POINT('Ctrl Pts',(-1.27156805265289,1.,1.45843906294697));
#31496=CARTESIAN_POINT('Ctrl Pts',(-1.27433119897822,-1.,1.46382431332476));
#31497=CARTESIAN_POINT('Ctrl Pts',(-1.27433119897822,1.,1.46382431332476));
#31498=CARTESIAN_POINT('Ctrl Pts',(-1.27696414831089,-1.,1.46916035917133));
#31499=CARTESIAN_POINT('Ctrl Pts',(-1.27696414831089,1.,1.46916035917133));
#31500=CARTESIAN_POINT('Ctrl Pts',(-1.2794891824849,-1.,1.4744717526707));
#31501=CARTESIAN_POINT('Ctrl Pts',(-1.2794891824849,1.,1.4744717526707));
#31502=CARTESIAN_POINT('Ctrl Pts',(-1.28194158939517,-1.,1.47980070347095));
#31503=CARTESIAN_POINT('Ctrl Pts',(-1.28194158939517,1.,1.47980070347095));
#31504=CARTESIAN_POINT('Ctrl Pts',(-1.28435533880201,-1.,1.4851881711891));
#31505=CARTESIAN_POINT('Ctrl Pts',(-1.28435533880201,1.,1.4851881711891));
#31506=CARTESIAN_POINT('Ctrl Pts',(-1.2867467611644,-1.,1.4906522831278));
#31507=CARTESIAN_POINT('Ctrl Pts',(-1.2867467611644,1.,1.4906522831278));
#31508=CARTESIAN_POINT('Ctrl Pts',(-1.28911506584254,-1.,1.49618896881754));
#31509=CARTESIAN_POINT('Ctrl Pts',(-1.28911506584254,1.,1.49618896881754));
#31510=CARTESIAN_POINT('Ctrl Pts',(-1.29145022885181,-1.,1.50178230149776));
#31511=CARTESIAN_POINT('Ctrl Pts',(-1.29145022885181,1.,1.50178230149776));
#31512=CARTESIAN_POINT('Ctrl Pts',(-1.29373841372842,-1.,1.50741159078365));
#31513=CARTESIAN_POINT('Ctrl Pts',(-1.29373841372842,1.,1.50741159078365));
#31514=CARTESIAN_POINT('Ctrl Pts',(-1.29596850710509,-1.,1.51305994241402));
#31515=CARTESIAN_POINT('Ctrl Pts',(-1.29596850710509,1.,1.51305994241402));
#31516=CARTESIAN_POINT('Ctrl Pts',(-1.29813791800747,-1.,1.51872184912724));
#31517=CARTESIAN_POINT('Ctrl Pts',(-1.29813791800747,1.,1.51872184912724));
#31518=CARTESIAN_POINT('Ctrl Pts',(-1.30024984366328,-1.,1.52439957861062));
#31519=CARTESIAN_POINT('Ctrl Pts',(-1.30024984366328,1.,1.52439957861062));
#31520=CARTESIAN_POINT('Ctrl Pts',(-1.30231064395568,-1.,1.53009970283891));
#31521=CARTESIAN_POINT('Ctrl Pts',(-1.30231064395568,1.,1.53009970283891));
#31522=CARTESIAN_POINT('Ctrl Pts',(-1.30432735639489,-1.,1.53582981268977));
#31523=CARTESIAN_POINT('Ctrl Pts',(-1.30432735639489,1.,1.53582981268977));
#31524=CARTESIAN_POINT('Ctrl Pts',(-1.30630475189556,-1.,1.54159462645432));
#31525=CARTESIAN_POINT('Ctrl Pts',(-1.30630475189556,1.,1.54159462645432));
#31526=CARTESIAN_POINT('Ctrl Pts',(-1.30824393907473,-1.,1.54739413957185));
#31527=CARTESIAN_POINT('Ctrl Pts',(-1.30824393907473,1.,1.54739413957185));
#31528=CARTESIAN_POINT('Ctrl Pts',(-1.31014393684222,-1.,1.55322568759481));
#31529=CARTESIAN_POINT('Ctrl Pts',(-1.31014393684222,1.,1.55322568759481));
#31530=CARTESIAN_POINT('Ctrl Pts',(-1.31200264341696,-1.,1.55908521254821));
#31531=CARTESIAN_POINT('Ctrl Pts',(-1.31200264341696,1.,1.55908521254821));
#31532=CARTESIAN_POINT('Ctrl Pts',(-1.31381795281002,-1.,1.56496872402353));
#31533=CARTESIAN_POINT('Ctrl Pts',(-1.31381795281002,1.,1.56496872402353));
#31534=CARTESIAN_POINT('Ctrl Pts',(-1.31558903860016,-1.,1.57087397835723));
#31535=CARTESIAN_POINT('Ctrl Pts',(-1.31558903860016,1.,1.57087397835723));
#31536=CARTESIAN_POINT('Ctrl Pts',(-1.31731642317187,-1.,1.5768005650559));
#31537=CARTESIAN_POINT('Ctrl Pts',(-1.31731642317187,1.,1.5768005650559));
#31538=CARTESIAN_POINT('Ctrl Pts',(-1.31900135021432,-1.,1.58274907898834));
#31539=CARTESIAN_POINT('Ctrl Pts',(-1.31900135021432,1.,1.58274907898834));
#31540=CARTESIAN_POINT('Ctrl Pts',(-1.32064537110892,-1.,1.58872057258245));
#31541=CARTESIAN_POINT('Ctrl Pts',(-1.32064537110892,1.,1.58872057258245));
#31542=CARTESIAN_POINT('Ctrl Pts',(-1.32224985747682,-1.,1.59471591079403));
#31543=CARTESIAN_POINT('Ctrl Pts',(-1.32224985747682,1.,1.59471591079403));
#31544=CARTESIAN_POINT('Ctrl Pts',(-1.32381550858256,-1.,1.60073511858687));
#31545=CARTESIAN_POINT('Ctrl Pts',(-1.32381550858256,1.,1.60073511858687));
#31546=CARTESIAN_POINT('Ctrl Pts',(-1.32534250785782,-1.,1.60677758290954));
#31547=CARTESIAN_POINT('Ctrl Pts',(-1.32534250785782,1.,1.60677758290954));
#31548=CARTESIAN_POINT('Ctrl Pts',(-1.32683074483356,-1.,1.6128423401575));
#31549=CARTESIAN_POINT('Ctrl Pts',(-1.32683074483356,1.,1.6128423401575));
#31550=CARTESIAN_POINT('Ctrl Pts',(-1.32828000610449,-1.,1.61892832270724));
#31551=CARTESIAN_POINT('Ctrl Pts',(-1.32828000610449,1.,1.61892832270724));
#31552=CARTESIAN_POINT('Ctrl Pts',(-1.3296901950568,-1.,1.62503464209797));
#31553=CARTESIAN_POINT('Ctrl Pts',(-1.3296901950568,1.,1.62503464209797));
#31554=CARTESIAN_POINT('Ctrl Pts',(-1.33106149345645,-1.,1.63116079730923));
#31555=CARTESIAN_POINT('Ctrl Pts',(-1.33106149345645,1.,1.63116079730923));
#31556=CARTESIAN_POINT('Ctrl Pts',(-1.33239425103724,-1.,1.63730653475089));
#31557=CARTESIAN_POINT('Ctrl Pts',(-1.33239425103724,1.,1.63730653475089));
#31558=CARTESIAN_POINT('Ctrl Pts',(-1.33368890676572,-1.,1.6434717485603));
#31559=CARTESIAN_POINT('Ctrl Pts',(-1.33368890676572,1.,1.6434717485603));
#31560=CARTESIAN_POINT('Ctrl Pts',(-1.33494590467993,-1.,1.6496563728683));
#31561=CARTESIAN_POINT('Ctrl Pts',(-1.33494590467993,1.,1.6496563728683));
#31562=CARTESIAN_POINT('Ctrl Pts',(-1.33616559745172,-1.,1.65586025952593));
#31563=CARTESIAN_POINT('Ctrl Pts',(-1.33616559745172,1.,1.65586025952593));
#31564=CARTESIAN_POINT('Ctrl Pts',(-1.33734820885262,-1.,1.66208312541983));
#31565=CARTESIAN_POINT('Ctrl Pts',(-1.33734820885262,1.,1.66208312541983));
#31566=CARTESIAN_POINT('Ctrl Pts',(-1.33849388654388,-1.,1.66832460783989));
#31567=CARTESIAN_POINT('Ctrl Pts',(-1.33849388654388,1.,1.66832460783989));
#31568=CARTESIAN_POINT('Ctrl Pts',(-1.3396027347034,-1.,1.67458429426086));
#31569=CARTESIAN_POINT('Ctrl Pts',(-1.3396027347034,1.,1.67458429426086));
#31570=CARTESIAN_POINT('Ctrl Pts',(-1.34067485185203,-1.,1.68086176030362));
#31571=CARTESIAN_POINT('Ctrl Pts',(-1.34067485185203,1.,1.68086176030362));
#31572=CARTESIAN_POINT('Ctrl Pts',(-1.341710374848,-1.,1.68715660868764));
#31573=CARTESIAN_POINT('Ctrl Pts',(-1.341710374848,1.,1.68715660868764));
#31574=CARTESIAN_POINT('Ctrl Pts',(-1.34270948206319,-1.,1.6934684849687));
#31575=CARTESIAN_POINT('Ctrl Pts',(-1.34270948206319,1.,1.6934684849687));
#31576=CARTESIAN_POINT('Ctrl Pts',(-1.34367237124483,-1.,1.69979707754427));
#31577=CARTESIAN_POINT('Ctrl Pts',(-1.34367237124483,1.,1.69979707754427));
#31578=CARTESIAN_POINT('Ctrl Pts',(-1.34459924533831,-1.,1.70614212266738));
#31579=CARTESIAN_POINT('Ctrl Pts',(-1.34459924533831,1.,1.70614212266738));
#31580=CARTESIAN_POINT('Ctrl Pts',(-1.34549029589416,-1.,1.71250340686822));
#31581=CARTESIAN_POINT('Ctrl Pts',(-1.34549029589416,1.,1.71250340686822));
#31582=CARTESIAN_POINT('Ctrl Pts',(-1.34634568653227,-1.,1.7188807715049));
#31583=CARTESIAN_POINT('Ctrl Pts',(-1.34634568653227,1.,1.7188807715049));
#31584=CARTESIAN_POINT('Ctrl Pts',(-1.34716554819527,-1.,1.72527410680674));
#31585=CARTESIAN_POINT('Ctrl Pts',(-1.34716554819527,1.,1.72527410680674));
#31586=CARTESIAN_POINT('Ctrl Pts',(-1.34779309152035,-1.,1.7304014965394));
#31587=CARTESIAN_POINT('Ctrl Pts',(-1.34779309152035,1.,1.7304014965394));
#31588=CARTESIAN_POINT('Ctrl Pts',(-1.34824783112887,-1.,1.73425417885907));
#31589=CARTESIAN_POINT('Ctrl Pts',(-1.34824783112887,1.,1.73425417885907));
#31590=CARTESIAN_POINT('Ctrl Pts',(-1.34854391898045,-1.,1.73682580585691));
#31591=CARTESIAN_POINT('Ctrl Pts',(-1.34854391898045,1.,1.73682580585691));
#31592=CARTESIAN_POINT('Ctrl Pts',(-1.34869019493419,-1.,1.73811241238545));
#31593=CARTESIAN_POINT('Ctrl Pts',(-1.34869019493419,1.,1.73811241238545));
#31594=CARTESIAN_POINT('',(-1.15624053661742,1.,1.31362392696032));
#31595=CARTESIAN_POINT('Ctrl Pts',(-1.15624053661742,1.,1.31362392696032));
#31596=CARTESIAN_POINT('Ctrl Pts',(-1.15950888730809,1.,1.31722977216397));
#31597=CARTESIAN_POINT('Ctrl Pts',(-1.16589330093588,1.,1.32428080721772));
#31598=CARTESIAN_POINT('Ctrl Pts',(-1.17501305789857,1.,1.33437539347008));
#31599=CARTESIAN_POINT('Ctrl Pts',(-1.18625865667441,1.,1.34687054001093));
#31600=CARTESIAN_POINT('Ctrl Pts',(-1.1987959077932,1.,1.36088705043885));
#31601=CARTESIAN_POINT('Ctrl Pts',(-1.20982812925645,1.,1.37331915607905));
#31602=CARTESIAN_POINT('Ctrl Pts',(-1.21938737280852,1.,1.38420564527715));
#31603=CARTESIAN_POINT('Ctrl Pts',(-1.22752961899387,1.,1.39361389568796));
#31604=CARTESIAN_POINT('Ctrl Pts',(-1.23434087290423,1.,1.40164708206106));
#31605=CARTESIAN_POINT('Ctrl Pts',(-1.23994455029534,1.,1.40845295531283));
#31606=CARTESIAN_POINT('Ctrl Pts',(-1.24450600513056,1.,1.41422913175179));
#31607=CARTESIAN_POINT('Ctrl Pts',(-1.24824430986571,1.,1.41923722596025));
#31608=CARTESIAN_POINT('Ctrl Pts',(-1.2514145557001,1.,1.42378102115575));
#31609=CARTESIAN_POINT('Ctrl Pts',(-1.25426945222639,1.,1.42815938799387));
#31610=CARTESIAN_POINT('Ctrl Pts',(-1.25702687965755,1.,1.43262645609691));
#31611=CARTESIAN_POINT('Ctrl Pts',(-1.25983531012005,1.,1.43734919180848));
#31612=CARTESIAN_POINT('Ctrl Pts',(-1.26273903323859,1.,1.44236470511303));
#31613=CARTESIAN_POINT('Ctrl Pts',(-1.26570925118868,1.,1.44761985001662));
#31614=CARTESIAN_POINT('Ctrl Pts',(-1.2686778680489,1.,1.45301422764247));
#31615=CARTESIAN_POINT('Ctrl Pts',(-1.27156805265289,1.,1.45843906294697));
#31616=CARTESIAN_POINT('Ctrl Pts',(-1.27433119897822,1.,1.46382431332476));
#31617=CARTESIAN_POINT('Ctrl Pts',(-1.27696414831089,1.,1.46916035917133));
#31618=CARTESIAN_POINT('Ctrl Pts',(-1.2794891824849,1.,1.4744717526707));
#31619=CARTESIAN_POINT('Ctrl Pts',(-1.28194158939517,1.,1.47980070347095));
#31620=CARTESIAN_POINT('Ctrl Pts',(-1.28435533880201,1.,1.4851881711891));
#31621=CARTESIAN_POINT('Ctrl Pts',(-1.2867467611644,1.,1.4906522831278));
#31622=CARTESIAN_POINT('Ctrl Pts',(-1.28911506584254,1.,1.49618896881754));
#31623=CARTESIAN_POINT('Ctrl Pts',(-1.29145022885181,1.,1.50178230149776));
#31624=CARTESIAN_POINT('Ctrl Pts',(-1.29373841372842,1.,1.50741159078365));
#31625=CARTESIAN_POINT('Ctrl Pts',(-1.29596850710509,1.,1.51305994241402));
#31626=CARTESIAN_POINT('Ctrl Pts',(-1.29813791800747,1.,1.51872184912724));
#31627=CARTESIAN_POINT('Ctrl Pts',(-1.30024984366328,1.,1.52439957861062));
#31628=CARTESIAN_POINT('Ctrl Pts',(-1.30231064395568,1.,1.53009970283891));
#31629=CARTESIAN_POINT('Ctrl Pts',(-1.30432735639489,1.,1.53582981268977));
#31630=CARTESIAN_POINT('Ctrl Pts',(-1.30630475189556,1.,1.54159462645432));
#31631=CARTESIAN_POINT('Ctrl Pts',(-1.30824393907473,1.,1.54739413957185));
#31632=CARTESIAN_POINT('Ctrl Pts',(-1.31014393684222,1.,1.55322568759481));
#31633=CARTESIAN_POINT('Ctrl Pts',(-1.31200264341696,1.,1.55908521254821));
#31634=CARTESIAN_POINT('Ctrl Pts',(-1.31381795281002,1.,1.56496872402353));
#31635=CARTESIAN_POINT('Ctrl Pts',(-1.31558903860016,1.,1.57087397835723));
#31636=CARTESIAN_POINT('Ctrl Pts',(-1.31731642317187,1.,1.5768005650559));
#31637=CARTESIAN_POINT('Ctrl Pts',(-1.31900135021432,1.,1.58274907898834));
#31638=CARTESIAN_POINT('Ctrl Pts',(-1.32064537110892,1.,1.58872057258245));
#31639=CARTESIAN_POINT('Ctrl Pts',(-1.32224985747682,1.,1.59471591079403));
#31640=CARTESIAN_POINT('Ctrl Pts',(-1.32381550858256,1.,1.60073511858687));
#31641=CARTESIAN_POINT('Ctrl Pts',(-1.32534250785782,1.,1.60677758290954));
#31642=CARTESIAN_POINT('Ctrl Pts',(-1.32683074483356,1.,1.6128423401575));
#31643=CARTESIAN_POINT('Ctrl Pts',(-1.32828000610449,1.,1.61892832270724));
#31644=CARTESIAN_POINT('Ctrl Pts',(-1.3296901950568,1.,1.62503464209797));
#31645=CARTESIAN_POINT('Ctrl Pts',(-1.33106149345645,1.,1.63116079730923));
#31646=CARTESIAN_POINT('Ctrl Pts',(-1.33239425103724,1.,1.63730653475089));
#31647=CARTESIAN_POINT('Ctrl Pts',(-1.33368890676572,1.,1.6434717485603));
#31648=CARTESIAN_POINT('Ctrl Pts',(-1.33494590467993,1.,1.6496563728683));
#31649=CARTESIAN_POINT('Ctrl Pts',(-1.33616559745172,1.,1.65586025952593));
#31650=CARTESIAN_POINT('Ctrl Pts',(-1.33734820885262,1.,1.66208312541983));
#31651=CARTESIAN_POINT('Ctrl Pts',(-1.33849388654388,1.,1.66832460783989));
#31652=CARTESIAN_POINT('Ctrl Pts',(-1.3396027347034,1.,1.67458429426086));
#31653=CARTESIAN_POINT('Ctrl Pts',(-1.34067485185203,1.,1.68086176030362));
#31654=CARTESIAN_POINT('Ctrl Pts',(-1.341710374848,1.,1.68715660868764));
#31655=CARTESIAN_POINT('Ctrl Pts',(-1.34270948206319,1.,1.6934684849687));
#31656=CARTESIAN_POINT('Ctrl Pts',(-1.34367237124483,1.,1.69979707754427));
#31657=CARTESIAN_POINT('Ctrl Pts',(-1.34459924533831,1.,1.70614212266738));
#31658=CARTESIAN_POINT('Ctrl Pts',(-1.34549029589416,1.,1.71250340686822));
#31659=CARTESIAN_POINT('Ctrl Pts',(-1.34634568653227,1.,1.7188807715049));
#31660=CARTESIAN_POINT('Ctrl Pts',(-1.34716554819527,1.,1.72527410680674));
#31661=CARTESIAN_POINT('Ctrl Pts',(-1.34779309152035,1.,1.7304014965394));
#31662=CARTESIAN_POINT('Ctrl Pts',(-1.34824783112887,1.,1.73425417885907));
#31663=CARTESIAN_POINT('Ctrl Pts',(-1.34854391898045,1.,1.73682580585691));
#31664=CARTESIAN_POINT('Ctrl Pts',(-1.34869019493419,1.,1.73811241238545));
#31665=CARTESIAN_POINT('',(-1.15624053661742,0.,1.31362392696032));
#31666=CARTESIAN_POINT('Origin',(0.,0.,0.));
#31667=CARTESIAN_POINT('',(-1.31362392696033,1.,1.15624053661742));
#31668=CARTESIAN_POINT('Origin',(0.,1.,0.));
#31669=CARTESIAN_POINT('',(-1.31362392696033,0.,1.15624053661742));
#31670=CARTESIAN_POINT('Ctrl Pts',(-1.73811241238545,-1.,1.34869019493419));
#31671=CARTESIAN_POINT('Ctrl Pts',(-1.73811241238545,1.,1.34869019493419));
#31672=CARTESIAN_POINT('Ctrl Pts',(-1.73682580585819,-1.,1.34854391898145));
#31673=CARTESIAN_POINT('Ctrl Pts',(-1.73682580585819,1.,1.34854391898145));
#31674=CARTESIAN_POINT('Ctrl Pts',(-1.73425417886255,-1.,1.34824783113158));
#31675=CARTESIAN_POINT('Ctrl Pts',(-1.73425417886255,1.,1.34824783113158));
#31676=CARTESIAN_POINT('Ctrl Pts',(-1.73040149654497,-1.,1.3477930915247));
#31677=CARTESIAN_POINT('Ctrl Pts',(-1.73040149654497,1.,1.3477930915247));
#31678=CARTESIAN_POINT('Ctrl Pts',(-1.72527410681298,-1.,1.34716554820013));
#31679=CARTESIAN_POINT('Ctrl Pts',(-1.72527410681298,1.,1.34716554820013));
#31680=CARTESIAN_POINT('Ctrl Pts',(-1.7188807715095,-1.,1.34634568653586));
#31681=CARTESIAN_POINT('Ctrl Pts',(-1.7188807715095,1.,1.34634568653586));
#31682=CARTESIAN_POINT('Ctrl Pts',(-1.71250340687011,-1.,1.34549029589563));
#31683=CARTESIAN_POINT('Ctrl Pts',(-1.71250340687011,1.,1.34549029589563));
#31684=CARTESIAN_POINT('Ctrl Pts',(-1.70614212266676,-1.,1.34459924533783));
#31685=CARTESIAN_POINT('Ctrl Pts',(-1.70614212266676,1.,1.34459924533783));
#31686=CARTESIAN_POINT('Ctrl Pts',(-1.69979707754221,-1.,1.34367237124322));
#31687=CARTESIAN_POINT('Ctrl Pts',(-1.69979707754221,1.,1.34367237124322));
#31688=CARTESIAN_POINT('Ctrl Pts',(-1.6934684849664,-1.,1.34270948206139));
#31689=CARTESIAN_POINT('Ctrl Pts',(-1.6934684849664,1.,1.34270948206139));
#31690=CARTESIAN_POINT('Ctrl Pts',(-1.68715660868602,-1.,1.34171037484673));
#31691=CARTESIAN_POINT('Ctrl Pts',(-1.68715660868602,1.,1.34171037484673));
#31692=CARTESIAN_POINT('Ctrl Pts',(-1.68086176030308,-1.,1.3406748518516));
#31693=CARTESIAN_POINT('Ctrl Pts',(-1.68086176030308,1.,1.3406748518516));
#31694=CARTESIAN_POINT('Ctrl Pts',(-1.67458429426126,-1.,1.33960273470372));
#31695=CARTESIAN_POINT('Ctrl Pts',(-1.67458429426126,1.,1.33960273470372));
#31696=CARTESIAN_POINT('Ctrl Pts',(-1.66832460784078,-1.,1.33849388654458));
#31697=CARTESIAN_POINT('Ctrl Pts',(-1.66832460784078,1.,1.33849388654458));
#31698=CARTESIAN_POINT('Ctrl Pts',(-1.66208312542073,-1.,1.33734820885331));
#31699=CARTESIAN_POINT('Ctrl Pts',(-1.66208312542073,1.,1.33734820885331));
#31700=CARTESIAN_POINT('Ctrl Pts',(-1.65586025952651,-1.,1.33616559745217));
#31701=CARTESIAN_POINT('Ctrl Pts',(-1.65586025952651,1.,1.33616559745217));
#31702=CARTESIAN_POINT('Ctrl Pts',(-1.64965637286843,-1.,1.33494590468003));
#31703=CARTESIAN_POINT('Ctrl Pts',(-1.64965637286843,1.,1.33494590468003));
#31704=CARTESIAN_POINT('Ctrl Pts',(-1.64347174856007,-1.,1.33368890676554));
#31705=CARTESIAN_POINT('Ctrl Pts',(-1.64347174856007,1.,1.33368890676554));
#31706=CARTESIAN_POINT('Ctrl Pts',(-1.6373065347505,-1.,1.33239425103694));
#31707=CARTESIAN_POINT('Ctrl Pts',(-1.6373065347505,1.,1.33239425103694));
#31708=CARTESIAN_POINT('Ctrl Pts',(-1.63116079730887,-1.,1.33106149345618));
#31709=CARTESIAN_POINT('Ctrl Pts',(-1.63116079730887,1.,1.33106149345618));
#31710=CARTESIAN_POINT('Ctrl Pts',(-1.62503464209777,-1.,1.32969019505665));
#31711=CARTESIAN_POINT('Ctrl Pts',(-1.62503464209777,1.,1.32969019505665));
#31712=CARTESIAN_POINT('Ctrl Pts',(-1.61892832270723,-1.,1.32828000610448));
#31713=CARTESIAN_POINT('Ctrl Pts',(-1.61892832270723,1.,1.32828000610448));
#31714=CARTESIAN_POINT('Ctrl Pts',(-1.61284234015762,-1.,1.32683074483365));
#31715=CARTESIAN_POINT('Ctrl Pts',(-1.61284234015762,1.,1.32683074483365));
#31716=CARTESIAN_POINT('Ctrl Pts',(-1.6067775829097,-1.,1.32534250785794));
#31717=CARTESIAN_POINT('Ctrl Pts',(-1.6067775829097,1.,1.32534250785794));
#31718=CARTESIAN_POINT('Ctrl Pts',(-1.600735118587,-1.,1.32381550858266));
#31719=CARTESIAN_POINT('Ctrl Pts',(-1.600735118587,1.,1.32381550858266));
#31720=CARTESIAN_POINT('Ctrl Pts',(-1.59471591079408,-1.,1.32224985747686));
#31721=CARTESIAN_POINT('Ctrl Pts',(-1.59471591079408,1.,1.32224985747686));
#31722=CARTESIAN_POINT('Ctrl Pts',(-1.58872057258244,-1.,1.32064537110891));
#31723=CARTESIAN_POINT('Ctrl Pts',(-1.58872057258244,1.,1.32064537110891));
#31724=CARTESIAN_POINT('Ctrl Pts',(-1.58274907898829,-1.,1.31900135021428));
#31725=CARTESIAN_POINT('Ctrl Pts',(-1.58274907898829,1.,1.31900135021428));
#31726=CARTESIAN_POINT('Ctrl Pts',(-1.57680056505585,-1.,1.31731642317183));
#31727=CARTESIAN_POINT('Ctrl Pts',(-1.57680056505585,1.,1.31731642317183));
#31728=CARTESIAN_POINT('Ctrl Pts',(-1.57087397835721,-1.,1.31558903860015));
#31729=CARTESIAN_POINT('Ctrl Pts',(-1.57087397835721,1.,1.31558903860015));
#31730=CARTESIAN_POINT('Ctrl Pts',(-1.56496872402352,-1.,1.31381795281002));
#31731=CARTESIAN_POINT('Ctrl Pts',(-1.56496872402352,1.,1.31381795281002));
#31732=CARTESIAN_POINT('Ctrl Pts',(-1.55908521254822,-1.,1.31200264341696));
#31733=CARTESIAN_POINT('Ctrl Pts',(-1.55908521254822,1.,1.31200264341696));
#31734=CARTESIAN_POINT('Ctrl Pts',(-1.55322568759481,-1.,1.31014393684221));
#31735=CARTESIAN_POINT('Ctrl Pts',(-1.55322568759481,1.,1.31014393684221));
#31736=CARTESIAN_POINT('Ctrl Pts',(-1.54739413957183,-1.,1.30824393907471));
#31737=CARTESIAN_POINT('Ctrl Pts',(-1.54739413957183,1.,1.30824393907471));
#31738=CARTESIAN_POINT('Ctrl Pts',(-1.54159462645428,-1.,1.30630475189553));
#31739=CARTESIAN_POINT('Ctrl Pts',(-1.54159462645428,1.,1.30630475189553));
#31740=CARTESIAN_POINT('Ctrl Pts',(-1.53582981268976,-1.,1.30432735639487));
#31741=CARTESIAN_POINT('Ctrl Pts',(-1.53582981268976,1.,1.30432735639487));
#31742=CARTESIAN_POINT('Ctrl Pts',(-1.53009970283893,-1.,1.3023106439557));
#31743=CARTESIAN_POINT('Ctrl Pts',(-1.53009970283893,1.,1.3023106439557));
#31744=CARTESIAN_POINT('Ctrl Pts',(-1.5243995786107,-1.,1.30024984366334));
#31745=CARTESIAN_POINT('Ctrl Pts',(-1.5243995786107,1.,1.30024984366334));
#31746=CARTESIAN_POINT('Ctrl Pts',(-1.51872184912735,-1.,1.29813791800757));
#31747=CARTESIAN_POINT('Ctrl Pts',(-1.51872184912735,1.,1.29813791800757));
#31748=CARTESIAN_POINT('Ctrl Pts',(-1.51305994241412,-1.,1.29596850710518));
#31749=CARTESIAN_POINT('Ctrl Pts',(-1.51305994241412,1.,1.29596850710518));
#31750=CARTESIAN_POINT('Ctrl Pts',(-1.50741159078367,-1.,1.29373841372843));
#31751=CARTESIAN_POINT('Ctrl Pts',(-1.50741159078367,1.,1.29373841372843));
#31752=CARTESIAN_POINT('Ctrl Pts',(-1.50178230149764,-1.,1.29145022885171));
#31753=CARTESIAN_POINT('Ctrl Pts',(-1.50178230149764,1.,1.29145022885171));
#31754=CARTESIAN_POINT('Ctrl Pts',(-1.49618896881729,-1.,1.28911506584232));
#31755=CARTESIAN_POINT('Ctrl Pts',(-1.49618896881729,1.,1.28911506584232));
#31756=CARTESIAN_POINT('Ctrl Pts',(-1.4906522831275,-1.,1.28674676116415));
#31757=CARTESIAN_POINT('Ctrl Pts',(-1.4906522831275,1.,1.28674676116415));
#31758=CARTESIAN_POINT('Ctrl Pts',(-1.48518817118891,-1.,1.28435533880184));
#31759=CARTESIAN_POINT('Ctrl Pts',(-1.48518817118891,1.,1.28435533880184));
#31760=CARTESIAN_POINT('Ctrl Pts',(-1.47980070347102,-1.,1.28194158939522));
#31761=CARTESIAN_POINT('Ctrl Pts',(-1.47980070347102,1.,1.28194158939522));
#31762=CARTESIAN_POINT('Ctrl Pts',(-1.4744717526711,-1.,1.27948918248524));
#31763=CARTESIAN_POINT('Ctrl Pts',(-1.4744717526711,1.,1.27948918248524));
#31764=CARTESIAN_POINT('Ctrl Pts',(-1.46916035917197,-1.,1.27696414831144));
#31765=CARTESIAN_POINT('Ctrl Pts',(-1.46916035917197,1.,1.27696414831144));
#31766=CARTESIAN_POINT('Ctrl Pts',(-1.4638243133254,-1.,1.27433119897877));
#31767=CARTESIAN_POINT('Ctrl Pts',(-1.4638243133254,1.,1.27433119897877));
#31768=CARTESIAN_POINT('Ctrl Pts',(-1.45843906294725,-1.,1.27156805265312));
#31769=CARTESIAN_POINT('Ctrl Pts',(-1.45843906294725,1.,1.27156805265312));
#31770=CARTESIAN_POINT('Ctrl Pts',(-1.45301422764205,-1.,1.26867786804854));
#31771=CARTESIAN_POINT('Ctrl Pts',(-1.45301422764205,1.,1.26867786804854));
#31772=CARTESIAN_POINT('Ctrl Pts',(-1.44761985001544,-1.,1.26570925118767));
#31773=CARTESIAN_POINT('Ctrl Pts',(-1.44761985001544,1.,1.26570925118767));
#31774=CARTESIAN_POINT('Ctrl Pts',(-1.44236470511145,-1.,1.26273903323723));
#31775=CARTESIAN_POINT('Ctrl Pts',(-1.44236470511145,1.,1.26273903323723));
#31776=CARTESIAN_POINT('Ctrl Pts',(-1.43734919180719,-1.,1.25983531011894));
#31777=CARTESIAN_POINT('Ctrl Pts',(-1.43734919180719,1.,1.25983531011894));
#31778=CARTESIAN_POINT('Ctrl Pts',(-1.43262645609679,-1.,1.25702687965744));
#31779=CARTESIAN_POINT('Ctrl Pts',(-1.43262645609679,1.,1.25702687965744));
#31780=CARTESIAN_POINT('Ctrl Pts',(-1.42815938799555,-1.,1.25426945222783));
#31781=CARTESIAN_POINT('Ctrl Pts',(-1.42815938799555,1.,1.25426945222783));
#31782=CARTESIAN_POINT('Ctrl Pts',(-1.42378102115911,-1.,1.25141455570299));
#31783=CARTESIAN_POINT('Ctrl Pts',(-1.42378102115911,1.,1.25141455570299));
#31784=CARTESIAN_POINT('Ctrl Pts',(-1.41923722596421,-1.,1.24824430986911));
#31785=CARTESIAN_POINT('Ctrl Pts',(-1.41923722596421,1.,1.24824430986911));
#31786=CARTESIAN_POINT('Ctrl Pts',(-1.41422913175437,-1.,1.24450600513278));
#31787=CARTESIAN_POINT('Ctrl Pts',(-1.41422913175437,1.,1.24450600513278));
#31788=CARTESIAN_POINT('Ctrl Pts',(-1.40845295531151,-1.,1.23994455029421));
#31789=CARTESIAN_POINT('Ctrl Pts',(-1.40845295531151,1.,1.23994455029421));
#31790=CARTESIAN_POINT('Ctrl Pts',(-1.40164708205345,-1.,1.23434087289768));
#31791=CARTESIAN_POINT('Ctrl Pts',(-1.40164708205345,1.,1.23434087289768));
#31792=CARTESIAN_POINT('Ctrl Pts',(-1.39361389567257,-1.,1.22752961898063));
#31793=CARTESIAN_POINT('Ctrl Pts',(-1.39361389567257,1.,1.22752961898063));
#31794=CARTESIAN_POINT('Ctrl Pts',(-1.38420564525391,-1.,1.21938737278853));
#31795=CARTESIAN_POINT('Ctrl Pts',(-1.38420564525391,1.,1.21938737278853));
#31796=CARTESIAN_POINT('Ctrl Pts',(-1.37331915604962,-1.,1.20982812923113));
#31797=CARTESIAN_POINT('Ctrl Pts',(-1.37331915604962,1.,1.20982812923113));
#31798=CARTESIAN_POINT('Ctrl Pts',(-1.36088705040677,-1.,1.1987959077656));
#31799=CARTESIAN_POINT('Ctrl Pts',(-1.36088705040677,1.,1.1987959077656));
#31800=CARTESIAN_POINT('Ctrl Pts',(-1.34687053998157,-1.,1.18625865664915));
#31801=CARTESIAN_POINT('Ctrl Pts',(-1.34687053998157,1.,1.18625865664915));
#31802=CARTESIAN_POINT('Ctrl Pts',(-1.33437539344842,-1.,1.17501305787994));
#31803=CARTESIAN_POINT('Ctrl Pts',(-1.33437539344842,1.,1.17501305787994));
#31804=CARTESIAN_POINT('Ctrl Pts',(-1.32428080720544,-1.,1.16589330092532));
#31805=CARTESIAN_POINT('Ctrl Pts',(-1.32428080720544,1.,1.16589330092532));
#31806=CARTESIAN_POINT('Ctrl Pts',(-1.3172297721596,-1.,1.15950888730433));
#31807=CARTESIAN_POINT('Ctrl Pts',(-1.3172297721596,1.,1.15950888730433));
#31808=CARTESIAN_POINT('Ctrl Pts',(-1.31362392696033,-1.,1.15624053661742));
#31809=CARTESIAN_POINT('Ctrl Pts',(-1.31362392696033,1.,1.15624053661742));
#31810=CARTESIAN_POINT('',(-1.73811241238545,1.,1.34869019493419));
#31811=CARTESIAN_POINT('Ctrl Pts',(-1.73811241238545,1.,1.34869019493419));
#31812=CARTESIAN_POINT('Ctrl Pts',(-1.73682580585819,1.,1.34854391898145));
#31813=CARTESIAN_POINT('Ctrl Pts',(-1.73425417886255,1.,1.34824783113158));
#31814=CARTESIAN_POINT('Ctrl Pts',(-1.73040149654497,1.,1.3477930915247));
#31815=CARTESIAN_POINT('Ctrl Pts',(-1.72527410681298,1.,1.34716554820013));
#31816=CARTESIAN_POINT('Ctrl Pts',(-1.7188807715095,1.,1.34634568653586));
#31817=CARTESIAN_POINT('Ctrl Pts',(-1.71250340687011,1.,1.34549029589563));
#31818=CARTESIAN_POINT('Ctrl Pts',(-1.70614212266676,1.,1.34459924533783));
#31819=CARTESIAN_POINT('Ctrl Pts',(-1.69979707754221,1.,1.34367237124322));
#31820=CARTESIAN_POINT('Ctrl Pts',(-1.6934684849664,1.,1.34270948206139));
#31821=CARTESIAN_POINT('Ctrl Pts',(-1.68715660868602,1.,1.34171037484673));
#31822=CARTESIAN_POINT('Ctrl Pts',(-1.68086176030308,1.,1.3406748518516));
#31823=CARTESIAN_POINT('Ctrl Pts',(-1.67458429426126,1.,1.33960273470372));
#31824=CARTESIAN_POINT('Ctrl Pts',(-1.66832460784078,1.,1.33849388654458));
#31825=CARTESIAN_POINT('Ctrl Pts',(-1.66208312542073,1.,1.33734820885331));
#31826=CARTESIAN_POINT('Ctrl Pts',(-1.65586025952651,1.,1.33616559745217));
#31827=CARTESIAN_POINT('Ctrl Pts',(-1.64965637286843,1.,1.33494590468003));
#31828=CARTESIAN_POINT('Ctrl Pts',(-1.64347174856007,1.,1.33368890676554));
#31829=CARTESIAN_POINT('Ctrl Pts',(-1.6373065347505,1.,1.33239425103694));
#31830=CARTESIAN_POINT('Ctrl Pts',(-1.63116079730887,1.,1.33106149345618));
#31831=CARTESIAN_POINT('Ctrl Pts',(-1.62503464209777,1.,1.32969019505665));
#31832=CARTESIAN_POINT('Ctrl Pts',(-1.61892832270723,1.,1.32828000610448));
#31833=CARTESIAN_POINT('Ctrl Pts',(-1.61284234015762,1.,1.32683074483365));
#31834=CARTESIAN_POINT('Ctrl Pts',(-1.6067775829097,1.,1.32534250785794));
#31835=CARTESIAN_POINT('Ctrl Pts',(-1.600735118587,1.,1.32381550858266));
#31836=CARTESIAN_POINT('Ctrl Pts',(-1.59471591079408,1.,1.32224985747686));
#31837=CARTESIAN_POINT('Ctrl Pts',(-1.58872057258244,1.,1.32064537110891));
#31838=CARTESIAN_POINT('Ctrl Pts',(-1.58274907898829,1.,1.31900135021428));
#31839=CARTESIAN_POINT('Ctrl Pts',(-1.57680056505585,1.,1.31731642317183));
#31840=CARTESIAN_POINT('Ctrl Pts',(-1.57087397835721,1.,1.31558903860015));
#31841=CARTESIAN_POINT('Ctrl Pts',(-1.56496872402352,1.,1.31381795281002));
#31842=CARTESIAN_POINT('Ctrl Pts',(-1.55908521254822,1.,1.31200264341696));
#31843=CARTESIAN_POINT('Ctrl Pts',(-1.55322568759481,1.,1.31014393684221));
#31844=CARTESIAN_POINT('Ctrl Pts',(-1.54739413957183,1.,1.30824393907471));
#31845=CARTESIAN_POINT('Ctrl Pts',(-1.54159462645428,1.,1.30630475189553));
#31846=CARTESIAN_POINT('Ctrl Pts',(-1.53582981268976,1.,1.30432735639487));
#31847=CARTESIAN_POINT('Ctrl Pts',(-1.53009970283893,1.,1.3023106439557));
#31848=CARTESIAN_POINT('Ctrl Pts',(-1.5243995786107,1.,1.30024984366334));
#31849=CARTESIAN_POINT('Ctrl Pts',(-1.51872184912735,1.,1.29813791800757));
#31850=CARTESIAN_POINT('Ctrl Pts',(-1.51305994241412,1.,1.29596850710518));
#31851=CARTESIAN_POINT('Ctrl Pts',(-1.50741159078367,1.,1.29373841372843));
#31852=CARTESIAN_POINT('Ctrl Pts',(-1.50178230149764,1.,1.29145022885171));
#31853=CARTESIAN_POINT('Ctrl Pts',(-1.49618896881729,1.,1.28911506584232));
#31854=CARTESIAN_POINT('Ctrl Pts',(-1.4906522831275,1.,1.28674676116415));
#31855=CARTESIAN_POINT('Ctrl Pts',(-1.48518817118891,1.,1.28435533880184));
#31856=CARTESIAN_POINT('Ctrl Pts',(-1.47980070347102,1.,1.28194158939522));
#31857=CARTESIAN_POINT('Ctrl Pts',(-1.4744717526711,1.,1.27948918248524));
#31858=CARTESIAN_POINT('Ctrl Pts',(-1.46916035917197,1.,1.27696414831144));
#31859=CARTESIAN_POINT('Ctrl Pts',(-1.4638243133254,1.,1.27433119897877));
#31860=CARTESIAN_POINT('Ctrl Pts',(-1.45843906294725,1.,1.27156805265312));
#31861=CARTESIAN_POINT('Ctrl Pts',(-1.45301422764205,1.,1.26867786804854));
#31862=CARTESIAN_POINT('Ctrl Pts',(-1.44761985001544,1.,1.26570925118767));
#31863=CARTESIAN_POINT('Ctrl Pts',(-1.44236470511145,1.,1.26273903323723));
#31864=CARTESIAN_POINT('Ctrl Pts',(-1.43734919180719,1.,1.25983531011894));
#31865=CARTESIAN_POINT('Ctrl Pts',(-1.43262645609679,1.,1.25702687965744));
#31866=CARTESIAN_POINT('Ctrl Pts',(-1.42815938799555,1.,1.25426945222783));
#31867=CARTESIAN_POINT('Ctrl Pts',(-1.42378102115911,1.,1.25141455570299));
#31868=CARTESIAN_POINT('Ctrl Pts',(-1.41923722596421,1.,1.24824430986911));
#31869=CARTESIAN_POINT('Ctrl Pts',(-1.41422913175437,1.,1.24450600513278));
#31870=CARTESIAN_POINT('Ctrl Pts',(-1.40845295531151,1.,1.23994455029421));
#31871=CARTESIAN_POINT('Ctrl Pts',(-1.40164708205345,1.,1.23434087289768));
#31872=CARTESIAN_POINT('Ctrl Pts',(-1.39361389567257,1.,1.22752961898063));
#31873=CARTESIAN_POINT('Ctrl Pts',(-1.38420564525391,1.,1.21938737278853));
#31874=CARTESIAN_POINT('Ctrl Pts',(-1.37331915604962,1.,1.20982812923113));
#31875=CARTESIAN_POINT('Ctrl Pts',(-1.36088705040677,1.,1.1987959077656));
#31876=CARTESIAN_POINT('Ctrl Pts',(-1.34687053998157,1.,1.18625865664915));
#31877=CARTESIAN_POINT('Ctrl Pts',(-1.33437539344842,1.,1.17501305787994));
#31878=CARTESIAN_POINT('Ctrl Pts',(-1.32428080720544,1.,1.16589330092532));
#31879=CARTESIAN_POINT('Ctrl Pts',(-1.3172297721596,1.,1.15950888730433));
#31880=CARTESIAN_POINT('Ctrl Pts',(-1.31362392696033,1.,1.15624053661742));
#31881=CARTESIAN_POINT('',(-1.73811241238545,0.,1.34869019493419));
#31882=CARTESIAN_POINT('Origin',(-1.81978687191668,0.,1.23627494547115));
#31883=CARTESIAN_POINT('',(-1.81978687191668,1.,1.23627494547115));
#31884=CARTESIAN_POINT('',(-1.73811241238545,1.,1.34869019493419));
#31885=CARTESIAN_POINT('',(-1.81978687191668,0.,1.23627494547115));
#31886=CARTESIAN_POINT('Ctrl Pts',(-1.5055822144029,-1.,0.892032620296855));
#31887=CARTESIAN_POINT('Ctrl Pts',(-1.5055822144029,1.,0.892032620296855));
#31888=CARTESIAN_POINT('Ctrl Pts',(-1.50980486807181,-1.,0.894452006967538));
#31889=CARTESIAN_POINT('Ctrl Pts',(-1.50980486807181,1.,0.894452006967538));
#31890=CARTESIAN_POINT('Ctrl Pts',(-1.51805569591479,-1.,0.89918504749193));
#31891=CARTESIAN_POINT('Ctrl Pts',(-1.51805569591479,1.,0.89918504749193));
#31892=CARTESIAN_POINT('Ctrl Pts',(-1.52984849890434,-1.,0.905967409640499));
#31893=CARTESIAN_POINT('Ctrl Pts',(-1.52984849890434,1.,0.905967409640499));
#31894=CARTESIAN_POINT('Ctrl Pts',(-1.54440491152808,-1.,0.91437591904658));
#31895=CARTESIAN_POINT('Ctrl Pts',(-1.54440491152808,1.,0.91437591904658));
#31896=CARTESIAN_POINT('Ctrl Pts',(-1.56065988582509,-1.,0.923832188966322));
#31897=CARTESIAN_POINT('Ctrl Pts',(-1.56065988582509,1.,0.923832188966322));
#31898=CARTESIAN_POINT('Ctrl Pts',(-1.57499388385561,-1.,0.932246680128849));
#31899=CARTESIAN_POINT('Ctrl Pts',(-1.57499388385561,1.,0.932246680128849));
#31900=CARTESIAN_POINT('Ctrl Pts',(-1.58744937489796,-1.,0.939646377909319));
#31901=CARTESIAN_POINT('Ctrl Pts',(-1.58744937489796,1.,0.939646377909319));
#31902=CARTESIAN_POINT('Ctrl Pts',(-1.59810042045408,-1.,0.946078063325796));
#31903=CARTESIAN_POINT('Ctrl Pts',(-1.59810042045408,1.,0.946078063325796));
#31904=CARTESIAN_POINT('Ctrl Pts',(-1.60706069897794,-1.,0.951613284361248));
#31905=CARTESIAN_POINT('Ctrl Pts',(-1.60706069897794,1.,0.951613284361248));
#31906=CARTESIAN_POINT('Ctrl Pts',(-1.61449324337233,-1.,0.956354422921573));
#31907=CARTESIAN_POINT('Ctrl Pts',(-1.61449324337233,1.,0.956354422921573));
#31908=CARTESIAN_POINT('Ctrl Pts',(-1.62061638139929,-1.,0.960438326099958));
#31909=CARTESIAN_POINT('Ctrl Pts',(-1.62061638139929,1.,0.960438326099958));
#31910=CARTESIAN_POINT('Ctrl Pts',(-1.6257193066974,-1.,0.964046107037821));
#31911=CARTESIAN_POINT('Ctrl Pts',(-1.6257193066974,1.,0.964046107037821));
#31912=CARTESIAN_POINT('Ctrl Pts',(-1.63013849959083,-1.,0.967387853228041));
#31913=CARTESIAN_POINT('Ctrl Pts',(-1.63013849959083,1.,0.967387853228041));
#31914=CARTESIAN_POINT('Ctrl Pts',(-1.63420665729609,-1.,0.970669715996356));
#31915=CARTESIAN_POINT('Ctrl Pts',(-1.63420665729609,1.,0.970669715996356));
#31916=CARTESIAN_POINT('Ctrl Pts',(-1.63820952658157,-1.,0.974066058287501));
#31917=CARTESIAN_POINT('Ctrl Pts',(-1.63820952658157,1.,0.974066058287501));
#31918=CARTESIAN_POINT('Ctrl Pts',(-1.64233990826831,-1.,0.977689794120297));
#31919=CARTESIAN_POINT('Ctrl Pts',(-1.64233990826831,1.,0.977689794120297));
#31920=CARTESIAN_POINT('Ctrl Pts',(-1.64665139190834,-1.,0.981562530940574));
#31921=CARTESIAN_POINT('Ctrl Pts',(-1.64665139190834,1.,0.981562530940574));
#31922=CARTESIAN_POINT('Ctrl Pts',(-1.6511001661277,-1.,0.985642622921626));
#31923=CARTESIAN_POINT('Ctrl Pts',(-1.6511001661277,1.,0.985642622921626));
#31924=CARTESIAN_POINT('Ctrl Pts',(-1.65559044289746,-1.,0.98985562785445));
#31925=CARTESIAN_POINT('Ctrl Pts',(-1.65559044289746,1.,0.98985562785445));
#31926=CARTESIAN_POINT('Ctrl Pts',(-1.66001553809916,-1.,0.994121836661116));
#31927=CARTESIAN_POINT('Ctrl Pts',(-1.66001553809916,1.,0.994121836661116));
#31928=CARTESIAN_POINT('Ctrl Pts',(-1.66430758030304,-1.,0.998389654952317));
#31929=CARTESIAN_POINT('Ctrl Pts',(-1.66430758030304,1.,0.998389654952317));
#31930=CARTESIAN_POINT('Ctrl Pts',(-1.66846059277231,-1.,1.00265091003682));
#31931=CARTESIAN_POINT('Ctrl Pts',(-1.66846059277231,1.,1.00265091003682));
#31932=CARTESIAN_POINT('Ctrl Pts',(-1.67250335383248,-1.,1.00692206696387));
#31933=CARTESIAN_POINT('Ctrl Pts',(-1.67250335383248,1.,1.00692206696387));
#31934=CARTESIAN_POINT('Ctrl Pts',(-1.67648246776457,-1.,1.01123236493507));
#31935=CARTESIAN_POINT('Ctrl Pts',(-1.67648246776457,1.,1.01123236493507));
#31936=CARTESIAN_POINT('Ctrl Pts',(-1.6804428989482,-1.,1.01561026162787));
#31937=CARTESIAN_POINT('Ctrl Pts',(-1.6804428989482,1.,1.01561026162787));
#31938=CARTESIAN_POINT('Ctrl Pts',(-1.68440578021739,-1.,1.02006795074222));
#31939=CARTESIAN_POINT('Ctrl Pts',(-1.68440578021739,1.,1.02006795074222));
#31940=CARTESIAN_POINT('Ctrl Pts',(-1.68836910178475,-1.,1.02460180535272));
#31941=CARTESIAN_POINT('Ctrl Pts',(-1.68836910178475,1.,1.02460180535272));
#31942=CARTESIAN_POINT('Ctrl Pts',(-1.69231840863471,-1.,1.02919977579155));
#31943=CARTESIAN_POINT('Ctrl Pts',(-1.69231840863471,1.,1.02919977579155));
#31944=CARTESIAN_POINT('Ctrl Pts',(-1.69623414782769,-1.,1.03384646003587));
#31945=CARTESIAN_POINT('Ctrl Pts',(-1.69623414782769,1.,1.03384646003587));
#31946=CARTESIAN_POINT('Ctrl Pts',(-1.70010052930951,-1.,1.03852922490782));
#31947=CARTESIAN_POINT('Ctrl Pts',(-1.70010052930951,1.,1.03852922490782));
#31948=CARTESIAN_POINT('Ctrl Pts',(-1.70391338707969,-1.,1.04324363334546));
#31949=CARTESIAN_POINT('Ctrl Pts',(-1.70391338707969,1.,1.04324363334546));
#31950=CARTESIAN_POINT('Ctrl Pts',(-1.70767646263641,-1.,1.0479908540499));
#31951=CARTESIAN_POINT('Ctrl Pts',(-1.70767646263641,1.,1.0479908540499));
#31952=CARTESIAN_POINT('Ctrl Pts',(-1.71139783543986,-1.,1.05277517202854));
#31953=CARTESIAN_POINT('Ctrl Pts',(-1.71139783543986,1.,1.05277517202854));
#31954=CARTESIAN_POINT('Ctrl Pts',(-1.71508654427022,-1.,1.05760163192481));
#31955=CARTESIAN_POINT('Ctrl Pts',(-1.71508654427022,1.,1.05760163192481));
#31956=CARTESIAN_POINT('Ctrl Pts',(-1.71874858456908,-1.,1.0624732468065));
#31957=CARTESIAN_POINT('Ctrl Pts',(-1.71874858456908,1.,1.0624732468065));
#31958=CARTESIAN_POINT('Ctrl Pts',(-1.72238500928456,-1.,1.06738966975463));
#31959=CARTESIAN_POINT('Ctrl Pts',(-1.72238500928456,1.,1.06738966975463));
#31960=CARTESIAN_POINT('Ctrl Pts',(-1.72599406198489,-1.,1.07234866990252));
#31961=CARTESIAN_POINT('Ctrl Pts',(-1.72599406198489,1.,1.07234866990252));
#31962=CARTESIAN_POINT('Ctrl Pts',(-1.72957248977424,-1.,1.0773470373727));
#31963=CARTESIAN_POINT('Ctrl Pts',(-1.72957248977424,1.,1.0773470373727));
#31964=CARTESIAN_POINT('Ctrl Pts',(-1.73311705663407,-1.,1.08238162784749));
#31965=CARTESIAN_POINT('Ctrl Pts',(-1.73311705663407,1.,1.08238162784749));
#31966=CARTESIAN_POINT('Ctrl Pts',(-1.73662628326093,-1.,1.08745056285429));
#31967=CARTESIAN_POINT('Ctrl Pts',(-1.73662628326093,1.,1.08745056285429));
#31968=CARTESIAN_POINT('Ctrl Pts',(-1.74010053962252,-1.,1.09255329056496));
#31969=CARTESIAN_POINT('Ctrl Pts',(-1.74010053962252,1.,1.09255329056496));
#31970=CARTESIAN_POINT('Ctrl Pts',(-1.74354119236212,-1.,1.09768999241229));
#31971=CARTESIAN_POINT('Ctrl Pts',(-1.74354119236212,1.,1.09768999241229));
#31972=CARTESIAN_POINT('Ctrl Pts',(-1.74695004214924,-1.,1.10286118991144));
#31973=CARTESIAN_POINT('Ctrl Pts',(-1.74695004214924,1.,1.10286118991144));
#31974=CARTESIAN_POINT('Ctrl Pts',(-1.75032866075914,-1.,1.10806728183003));
#31975=CARTESIAN_POINT('Ctrl Pts',(-1.75032866075914,1.,1.10806728183003));
#31976=CARTESIAN_POINT('Ctrl Pts',(-1.75367772094617,-1.,1.11330807582542));
#31977=CARTESIAN_POINT('Ctrl Pts',(-1.75367772094617,1.,1.11330807582542));
#31978=CARTESIAN_POINT('Ctrl Pts',(-1.75699720772089,-1.,1.11858293216752));
#31979=CARTESIAN_POINT('Ctrl Pts',(-1.75699720772089,1.,1.11858293216752));
#31980=CARTESIAN_POINT('Ctrl Pts',(-1.76028671825084,-1.,1.12389096855078));
#31981=CARTESIAN_POINT('Ctrl Pts',(-1.76028671825084,1.,1.12389096855078));
#31982=CARTESIAN_POINT('Ctrl Pts',(-1.76354571966171,-1.,1.12923123555076));
#31983=CARTESIAN_POINT('Ctrl Pts',(-1.76354571966171,1.,1.12923123555076));
#31984=CARTESIAN_POINT('Ctrl Pts',(-1.76677384551883,-1.,1.13460291804635));
#31985=CARTESIAN_POINT('Ctrl Pts',(-1.76677384551883,1.,1.13460291804635));
#31986=CARTESIAN_POINT('Ctrl Pts',(-1.76997111386806,-1.,1.14000548337));
#31987=CARTESIAN_POINT('Ctrl Pts',(-1.76997111386806,1.,1.14000548337));
#31988=CARTESIAN_POINT('Ctrl Pts',(-1.77313777896234,-1.,1.14543858226948));
#31989=CARTESIAN_POINT('Ctrl Pts',(-1.77313777896234,1.,1.14543858226948));
#31990=CARTESIAN_POINT('Ctrl Pts',(-1.77627422557034,-1.,1.15090197841531));
#31991=CARTESIAN_POINT('Ctrl Pts',(-1.77627422557034,1.,1.15090197841531));
#31992=CARTESIAN_POINT('Ctrl Pts',(-1.77938085564261,-1.,1.15639547194689));
#31993=CARTESIAN_POINT('Ctrl Pts',(-1.77938085564261,1.,1.15639547194689));
#31994=CARTESIAN_POINT('Ctrl Pts',(-1.78245795880949,-1.,1.16191881298458));
#31995=CARTESIAN_POINT('Ctrl Pts',(-1.78245795880949,1.,1.16191881298458));
#31996=CARTESIAN_POINT('Ctrl Pts',(-1.78550566040349,-1.,1.16747166312239));
#31997=CARTESIAN_POINT('Ctrl Pts',(-1.78550566040349,1.,1.16747166312239));
#31998=CARTESIAN_POINT('Ctrl Pts',(-1.78852398877523,-1.,1.17305363177265));
#31999=CARTESIAN_POINT('Ctrl Pts',(-1.78852398877523,1.,1.17305363177265));
#32000=CARTESIAN_POINT('Ctrl Pts',(-1.79151291552646,-1.,1.17866429440781));
#32001=CARTESIAN_POINT('Ctrl Pts',(-1.79151291552646,1.,1.17866429440781));
#32002=CARTESIAN_POINT('Ctrl Pts',(-1.79447240321572,-1.,1.18430321697471));
#32003=CARTESIAN_POINT('Ctrl Pts',(-1.79447240321572,1.,1.18430321697471));
#32004=CARTESIAN_POINT('Ctrl Pts',(-1.79740245923649,-1.,1.1899699793456));
#32005=CARTESIAN_POINT('Ctrl Pts',(-1.79740245923649,1.,1.1899699793456));
#32006=CARTESIAN_POINT('Ctrl Pts',(-1.80030314370121,-1.,1.19566418930405));
#32007=CARTESIAN_POINT('Ctrl Pts',(-1.80030314370121,1.,1.19566418930405));
#32008=CARTESIAN_POINT('Ctrl Pts',(-1.8031745483882,-1.,1.2013854893912));
#32009=CARTESIAN_POINT('Ctrl Pts',(-1.8031745483882,1.,1.2013854893912));
#32010=CARTESIAN_POINT('Ctrl Pts',(-1.80601678480772,-1.,1.20713356605519));
#32011=CARTESIAN_POINT('Ctrl Pts',(-1.80601678480772,1.,1.20713356605519));
#32012=CARTESIAN_POINT('Ctrl Pts',(-1.80882996916931,-1.,1.2129081570818));
#32013=CARTESIAN_POINT('Ctrl Pts',(-1.80882996916931,1.,1.2129081570818));
#32014=CARTESIAN_POINT('Ctrl Pts',(-1.81161420806172,-1.,1.2187090610323));
#32015=CARTESIAN_POINT('Ctrl Pts',(-1.81161420806172,1.,1.2187090610323));
#32016=CARTESIAN_POINT('Ctrl Pts',(-1.81436959209778,-1.,1.22453613304507));
#32017=CARTESIAN_POINT('Ctrl Pts',(-1.81436959209778,1.,1.22453613304507));
#32018=CARTESIAN_POINT('Ctrl Pts',(-1.81655087183054,-1.,1.22921864890975));
#32019=CARTESIAN_POINT('Ctrl Pts',(-1.81655087183054,1.,1.22921864890975));
#32020=CARTESIAN_POINT('Ctrl Pts',(-1.81817389920914,-1.,1.23274224526804));
#32021=CARTESIAN_POINT('Ctrl Pts',(-1.81817389920914,1.,1.23274224526804));
#32022=CARTESIAN_POINT('Ctrl Pts',(-1.81925017193531,-1.,1.23509651170384));
#32023=CARTESIAN_POINT('Ctrl Pts',(-1.81925017193531,1.,1.23509651170384));
#32024=CARTESIAN_POINT('Ctrl Pts',(-1.81978687191668,-1.,1.23627494547115));
#32025=CARTESIAN_POINT('Ctrl Pts',(-1.81978687191668,1.,1.23627494547115));
#32026=CARTESIAN_POINT('',(-1.5055822144029,1.,0.892032620296855));
#32027=CARTESIAN_POINT('Ctrl Pts',(-1.5055822144029,1.,0.892032620296855));
#32028=CARTESIAN_POINT('Ctrl Pts',(-1.50980486807181,1.,0.894452006967538));
#32029=CARTESIAN_POINT('Ctrl Pts',(-1.51805569591479,1.,0.89918504749193));
#32030=CARTESIAN_POINT('Ctrl Pts',(-1.52984849890434,1.,0.905967409640499));
#32031=CARTESIAN_POINT('Ctrl Pts',(-1.54440491152808,1.,0.91437591904658));
#32032=CARTESIAN_POINT('Ctrl Pts',(-1.56065988582509,1.,0.923832188966322));
#32033=CARTESIAN_POINT('Ctrl Pts',(-1.57499388385561,1.,0.932246680128849));
#32034=CARTESIAN_POINT('Ctrl Pts',(-1.58744937489796,1.,0.939646377909319));
#32035=CARTESIAN_POINT('Ctrl Pts',(-1.59810042045408,1.,0.946078063325796));
#32036=CARTESIAN_POINT('Ctrl Pts',(-1.60706069897794,1.,0.951613284361248));
#32037=CARTESIAN_POINT('Ctrl Pts',(-1.61449324337233,1.,0.956354422921573));
#32038=CARTESIAN_POINT('Ctrl Pts',(-1.62061638139929,1.,0.960438326099958));
#32039=CARTESIAN_POINT('Ctrl Pts',(-1.6257193066974,1.,0.964046107037821));
#32040=CARTESIAN_POINT('Ctrl Pts',(-1.63013849959083,1.,0.967387853228041));
#32041=CARTESIAN_POINT('Ctrl Pts',(-1.63420665729609,1.,0.970669715996356));
#32042=CARTESIAN_POINT('Ctrl Pts',(-1.63820952658157,1.,0.974066058287501));
#32043=CARTESIAN_POINT('Ctrl Pts',(-1.64233990826831,1.,0.977689794120297));
#32044=CARTESIAN_POINT('Ctrl Pts',(-1.64665139190834,1.,0.981562530940574));
#32045=CARTESIAN_POINT('Ctrl Pts',(-1.6511001661277,1.,0.985642622921626));
#32046=CARTESIAN_POINT('Ctrl Pts',(-1.65559044289746,1.,0.98985562785445));
#32047=CARTESIAN_POINT('Ctrl Pts',(-1.66001553809916,1.,0.994121836661116));
#32048=CARTESIAN_POINT('Ctrl Pts',(-1.66430758030304,1.,0.998389654952317));
#32049=CARTESIAN_POINT('Ctrl Pts',(-1.66846059277231,1.,1.00265091003682));
#32050=CARTESIAN_POINT('Ctrl Pts',(-1.67250335383248,1.,1.00692206696387));
#32051=CARTESIAN_POINT('Ctrl Pts',(-1.67648246776457,1.,1.01123236493507));
#32052=CARTESIAN_POINT('Ctrl Pts',(-1.6804428989482,1.,1.01561026162787));
#32053=CARTESIAN_POINT('Ctrl Pts',(-1.68440578021739,1.,1.02006795074222));
#32054=CARTESIAN_POINT('Ctrl Pts',(-1.68836910178475,1.,1.02460180535272));
#32055=CARTESIAN_POINT('Ctrl Pts',(-1.69231840863471,1.,1.02919977579155));
#32056=CARTESIAN_POINT('Ctrl Pts',(-1.69623414782769,1.,1.03384646003587));
#32057=CARTESIAN_POINT('Ctrl Pts',(-1.70010052930951,1.,1.03852922490782));
#32058=CARTESIAN_POINT('Ctrl Pts',(-1.70391338707969,1.,1.04324363334546));
#32059=CARTESIAN_POINT('Ctrl Pts',(-1.70767646263641,1.,1.0479908540499));
#32060=CARTESIAN_POINT('Ctrl Pts',(-1.71139783543986,1.,1.05277517202854));
#32061=CARTESIAN_POINT('Ctrl Pts',(-1.71508654427022,1.,1.05760163192481));
#32062=CARTESIAN_POINT('Ctrl Pts',(-1.71874858456908,1.,1.0624732468065));
#32063=CARTESIAN_POINT('Ctrl Pts',(-1.72238500928456,1.,1.06738966975463));
#32064=CARTESIAN_POINT('Ctrl Pts',(-1.72599406198489,1.,1.07234866990252));
#32065=CARTESIAN_POINT('Ctrl Pts',(-1.72957248977424,1.,1.0773470373727));
#32066=CARTESIAN_POINT('Ctrl Pts',(-1.73311705663407,1.,1.08238162784749));
#32067=CARTESIAN_POINT('Ctrl Pts',(-1.73662628326093,1.,1.08745056285429));
#32068=CARTESIAN_POINT('Ctrl Pts',(-1.74010053962252,1.,1.09255329056496));
#32069=CARTESIAN_POINT('Ctrl Pts',(-1.74354119236212,1.,1.09768999241229));
#32070=CARTESIAN_POINT('Ctrl Pts',(-1.74695004214924,1.,1.10286118991144));
#32071=CARTESIAN_POINT('Ctrl Pts',(-1.75032866075914,1.,1.10806728183003));
#32072=CARTESIAN_POINT('Ctrl Pts',(-1.75367772094617,1.,1.11330807582542));
#32073=CARTESIAN_POINT('Ctrl Pts',(-1.75699720772089,1.,1.11858293216752));
#32074=CARTESIAN_POINT('Ctrl Pts',(-1.76028671825084,1.,1.12389096855078));
#32075=CARTESIAN_POINT('Ctrl Pts',(-1.76354571966171,1.,1.12923123555076));
#32076=CARTESIAN_POINT('Ctrl Pts',(-1.76677384551883,1.,1.13460291804635));
#32077=CARTESIAN_POINT('Ctrl Pts',(-1.76997111386806,1.,1.14000548337));
#32078=CARTESIAN_POINT('Ctrl Pts',(-1.77313777896234,1.,1.14543858226948));
#32079=CARTESIAN_POINT('Ctrl Pts',(-1.77627422557034,1.,1.15090197841531));
#32080=CARTESIAN_POINT('Ctrl Pts',(-1.77938085564261,1.,1.15639547194689));
#32081=CARTESIAN_POINT('Ctrl Pts',(-1.78245795880949,1.,1.16191881298458));
#32082=CARTESIAN_POINT('Ctrl Pts',(-1.78550566040349,1.,1.16747166312239));
#32083=CARTESIAN_POINT('Ctrl Pts',(-1.78852398877523,1.,1.17305363177265));
#32084=CARTESIAN_POINT('Ctrl Pts',(-1.79151291552646,1.,1.17866429440781));
#32085=CARTESIAN_POINT('Ctrl Pts',(-1.79447240321572,1.,1.18430321697471));
#32086=CARTESIAN_POINT('Ctrl Pts',(-1.79740245923649,1.,1.1899699793456));
#32087=CARTESIAN_POINT('Ctrl Pts',(-1.80030314370121,1.,1.19566418930405));
#32088=CARTESIAN_POINT('Ctrl Pts',(-1.8031745483882,1.,1.2013854893912));
#32089=CARTESIAN_POINT('Ctrl Pts',(-1.80601678480772,1.,1.20713356605519));
#32090=CARTESIAN_POINT('Ctrl Pts',(-1.80882996916931,1.,1.2129081570818));
#32091=CARTESIAN_POINT('Ctrl Pts',(-1.81161420806172,1.,1.2187090610323));
#32092=CARTESIAN_POINT('Ctrl Pts',(-1.81436959209778,1.,1.22453613304507));
#32093=CARTESIAN_POINT('Ctrl Pts',(-1.81655087183054,1.,1.22921864890975));
#32094=CARTESIAN_POINT('Ctrl Pts',(-1.81817389920914,1.,1.23274224526804));
#32095=CARTESIAN_POINT('Ctrl Pts',(-1.81925017193531,1.,1.23509651170384));
#32096=CARTESIAN_POINT('Ctrl Pts',(-1.81978687191668,1.,1.23627494547115));
#32097=CARTESIAN_POINT('',(-1.5055822144029,0.,0.892032620296856));
#32098=CARTESIAN_POINT('Origin',(0.,0.,0.));
#32099=CARTESIAN_POINT('',(-1.60662857109684,1.,0.693717979106305));
#32100=CARTESIAN_POINT('Origin',(0.,1.,0.));
#32101=CARTESIAN_POINT('',(-1.60662857109684,0.,0.693717979106306));
#32102=CARTESIAN_POINT('Ctrl Pts',(-2.0698113262342,-1.,0.7455743247944));
#32103=CARTESIAN_POINT('Ctrl Pts',(-2.0698113262342,1.,0.7455743247944));
#32104=CARTESIAN_POINT('Ctrl Pts',(-2.06854248895728,-1.,0.745832791378367));
#32105=CARTESIAN_POINT('Ctrl Pts',(-2.06854248895728,1.,0.745832791378367));
#32106=CARTESIAN_POINT('Ctrl Pts',(-2.06600523016815,-1.,0.7463458715442));
#32107=CARTESIAN_POINT('Ctrl Pts',(-2.06600523016815,1.,0.7463458715442));
#32108=CARTESIAN_POINT('Ctrl Pts',(-2.06220058927826,-1.,0.747103932787919));
#32109=CARTESIAN_POINT('Ctrl Pts',(-2.06220058927826,1.,0.747103932787919));
#32110=CARTESIAN_POINT('Ctrl Pts',(-2.05713023031006,-1.,0.748091554183802));
#32111=CARTESIAN_POINT('Ctrl Pts',(-2.05713023031006,1.,0.748091554183802));
#32112=CARTESIAN_POINT('Ctrl Pts',(-2.05079645592154,-1.,0.749287468665046));
#32113=CARTESIAN_POINT('Ctrl Pts',(-2.05079645592154,1.,0.749287468665046));
#32114=CARTESIAN_POINT('Ctrl Pts',(-2.04446689147979,-1.,0.750444657875576));
#32115=CARTESIAN_POINT('Ctrl Pts',(-2.04446689147979,1.,0.750444657875576));
#32116=CARTESIAN_POINT('Ctrl Pts',(-2.03814160092099,-1.,0.751562963361115));
#32117=CARTESIAN_POINT('Ctrl Pts',(-2.03814160092099,1.,0.751562963361115));
#32118=CARTESIAN_POINT('Ctrl Pts',(-2.03182068456221,-1.,0.752642180487211));
#32119=CARTESIAN_POINT('Ctrl Pts',(-2.03182068456221,1.,0.752642180487211));
#32120=CARTESIAN_POINT('Ctrl Pts',(-2.02550428623313,-1.,0.753682061112768));
#32121=CARTESIAN_POINT('Ctrl Pts',(-2.02550428623313,1.,0.753682061112768));
#32122=CARTESIAN_POINT('Ctrl Pts',(-2.01919259405809,-1.,0.754682330722816));
#32123=CARTESIAN_POINT('Ctrl Pts',(-2.01919259405809,1.,0.754682330722816));
#32124=CARTESIAN_POINT('Ctrl Pts',(-2.01288584328084,-1.,0.755642704957865));
#32125=CARTESIAN_POINT('Ctrl Pts',(-2.01288584328084,1.,0.755642704957865));
#32126=CARTESIAN_POINT('Ctrl Pts',(-2.0065843158773,-1.,0.75656290464667));
#32127=CARTESIAN_POINT('Ctrl Pts',(-2.0065843158773,1.,0.75656290464667));
#32128=CARTESIAN_POINT('Ctrl Pts',(-2.00028834739178,-1.,0.757442676862724));
#32129=CARTESIAN_POINT('Ctrl Pts',(-2.00028834739178,1.,0.757442676862724));
#32130=CARTESIAN_POINT('Ctrl Pts',(-1.99399831098817,-1.,0.758281796766761));
#32131=CARTESIAN_POINT('Ctrl Pts',(-1.99399831098817,1.,0.758281796766761));
#32132=CARTESIAN_POINT('Ctrl Pts',(-1.98771456680874,-1.,0.759080037802488));
#32133=CARTESIAN_POINT('Ctrl Pts',(-1.98771456680874,1.,0.759080037802488));
#32134=CARTESIAN_POINT('Ctrl Pts',(-1.98143741418172,-1.,0.75983714745219));
#32135=CARTESIAN_POINT('Ctrl Pts',(-1.98143741418172,1.,0.75983714745219));
#32136=CARTESIAN_POINT('Ctrl Pts',(-1.97516705321494,-1.,0.760552825409757));
#32137=CARTESIAN_POINT('Ctrl Pts',(-1.97516705321494,1.,0.760552825409757));
#32138=CARTESIAN_POINT('Ctrl Pts',(-1.96890351582499,-1.,0.76122669048382));
#32139=CARTESIAN_POINT('Ctrl Pts',(-1.96890351582499,1.,0.76122669048382));
#32140=CARTESIAN_POINT('Ctrl Pts',(-1.96264672744186,-1.,0.761858300014423));
#32141=CARTESIAN_POINT('Ctrl Pts',(-1.96264672744186,1.,0.761858300014423));
#32142=CARTESIAN_POINT('Ctrl Pts',(-1.95639665309869,-1.,0.762447203806179));
#32143=CARTESIAN_POINT('Ctrl Pts',(-1.95639665309869,1.,0.762447203806179));
#32144=CARTESIAN_POINT('Ctrl Pts',(-1.95015342590024,-1.,0.762992990878769));
#32145=CARTESIAN_POINT('Ctrl Pts',(-1.95015342590024,1.,0.762992990878769));
#32146=CARTESIAN_POINT('Ctrl Pts',(-1.9439174661764,-1.,0.763495333538629));
#32147=CARTESIAN_POINT('Ctrl Pts',(-1.9439174661764,1.,0.763495333538629));
#32148=CARTESIAN_POINT('Ctrl Pts',(-1.93768964875886,-1.,0.763954049121458));
#32149=CARTESIAN_POINT('Ctrl Pts',(-1.93768964875886,1.,0.763954049121458));
#32150=CARTESIAN_POINT('Ctrl Pts',(-1.93147105496382,-1.,0.76436901067394));
#32151=CARTESIAN_POINT('Ctrl Pts',(-1.93147105496382,1.,0.76436901067394));
#32152=CARTESIAN_POINT('Ctrl Pts',(-1.92526263537048,-1.,0.764740025488211));
#32153=CARTESIAN_POINT('Ctrl Pts',(-1.92526263537048,1.,0.764740025488211));
#32154=CARTESIAN_POINT('Ctrl Pts',(-1.91906491634196,-1.,0.765066729667088));
#32155=CARTESIAN_POINT('Ctrl Pts',(-1.91906491634196,1.,0.765066729667088));
#32156=CARTESIAN_POINT('Ctrl Pts',(-1.91287765805169,-1.,0.765348465884722));
#32157=CARTESIAN_POINT('Ctrl Pts',(-1.91287765805169,1.,0.765348465884722));
#32158=CARTESIAN_POINT('Ctrl Pts',(-1.90669961402356,-1.,0.765584196937919));
#32159=CARTESIAN_POINT('Ctrl Pts',(-1.90669961402356,1.,0.765584196937919));
#32160=CARTESIAN_POINT('Ctrl Pts',(-1.90052930393596,-1.,0.765772772593386));
#32161=CARTESIAN_POINT('Ctrl Pts',(-1.90052930393596,1.,0.765772772593386));
#32162=CARTESIAN_POINT('Ctrl Pts',(-1.89436577771388,-1.,0.765913193856978));
#32163=CARTESIAN_POINT('Ctrl Pts',(-1.89436577771388,1.,0.765913193856978));
#32164=CARTESIAN_POINT('Ctrl Pts',(-1.88820926433409,-1.,0.766004837062091));
#32165=CARTESIAN_POINT('Ctrl Pts',(-1.88820926433409,1.,0.766004837062091));
#32166=CARTESIAN_POINT('Ctrl Pts',(-1.88206215302561,-1.,0.766047794851864));
#32167=CARTESIAN_POINT('Ctrl Pts',(-1.88206215302561,1.,0.766047794851864));
#32168=CARTESIAN_POINT('Ctrl Pts',(-1.87592888967883,-1.,0.766042837036744));
#32169=CARTESIAN_POINT('Ctrl Pts',(-1.87592888967883,1.,0.766042837036744));
#32170=CARTESIAN_POINT('Ctrl Pts',(-1.86981398314341,-1.,0.765990708546091));
#32171=CARTESIAN_POINT('Ctrl Pts',(-1.86981398314341,1.,0.765990708546091));
#32172=CARTESIAN_POINT('Ctrl Pts',(-1.86372027063312,-1.,0.765891519092547));
#32173=CARTESIAN_POINT('Ctrl Pts',(-1.86372027063312,1.,0.765891519092547));
#32174=CARTESIAN_POINT('Ctrl Pts',(-1.85764741390394,-1.,0.765744212909318));
#32175=CARTESIAN_POINT('Ctrl Pts',(-1.85764741390394,1.,0.765744212909318));
#32176=CARTESIAN_POINT('Ctrl Pts',(-1.85158945130063,-1.,0.765545710619062));
#32177=CARTESIAN_POINT('Ctrl Pts',(-1.85158945130063,1.,0.765545710619062));
#32178=CARTESIAN_POINT('Ctrl Pts',(-1.84553698875924,-1.,0.765291664862029));
#32179=CARTESIAN_POINT('Ctrl Pts',(-1.84553698875924,1.,0.765291664862029));
#32180=CARTESIAN_POINT('Ctrl Pts',(-1.83948181064835,-1.,0.764978057881737));
#32181=CARTESIAN_POINT('Ctrl Pts',(-1.83948181064835,1.,0.764978057881737));
#32182=CARTESIAN_POINT('Ctrl Pts',(-1.83342077227142,-1.,0.764602549687853));
#32183=CARTESIAN_POINT('Ctrl Pts',(-1.83342077227142,1.,0.764602549687853));
#32184=CARTESIAN_POINT('Ctrl Pts',(-1.82735991200065,-1.,0.764165902605995));
#32185=CARTESIAN_POINT('Ctrl Pts',(-1.82735991200065,1.,0.764165902605995));
#32186=CARTESIAN_POINT('Ctrl Pts',(-1.82131873145266,-1.,0.763673465462726));
#32187=CARTESIAN_POINT('Ctrl Pts',(-1.82131873145266,1.,0.763673465462726));
#32188=CARTESIAN_POINT('Ctrl Pts',(-1.8153211840553,-1.,0.763132003836634));
#32189=CARTESIAN_POINT('Ctrl Pts',(-1.8153211840553,1.,0.763132003836634));
#32190=CARTESIAN_POINT('Ctrl Pts',(-1.80938551463965,-1.,0.762546129463938));
#32191=CARTESIAN_POINT('Ctrl Pts',(-1.80938551463965,1.,0.762546129463938));
#32192=CARTESIAN_POINT('Ctrl Pts',(-1.80351583877342,-1.,0.761915336443547));
#32193=CARTESIAN_POINT('Ctrl Pts',(-1.80351583877342,1.,0.761915336443547));
#32194=CARTESIAN_POINT('Ctrl Pts',(-1.79768986997783,-1.,0.761229695230558));
#32195=CARTESIAN_POINT('Ctrl Pts',(-1.79768986997783,1.,0.761229695230558));
#32196=CARTESIAN_POINT('Ctrl Pts',(-1.7918581561088,-1.,0.760469555880749));
#32197=CARTESIAN_POINT('Ctrl Pts',(-1.7918581561088,1.,0.760469555880749));
#32198=CARTESIAN_POINT('Ctrl Pts',(-1.78596964884604,-1.,0.759614401110189));
#32199=CARTESIAN_POINT('Ctrl Pts',(-1.78596964884604,1.,0.759614401110189));
#32200=CARTESIAN_POINT('Ctrl Pts',(-1.77999411220945,-1.,0.758650626677518));
#32201=CARTESIAN_POINT('Ctrl Pts',(-1.77999411220945,1.,0.758650626677518));
#32202=CARTESIAN_POINT('Ctrl Pts',(-1.77394167108292,-1.,0.757578264077029));
#32203=CARTESIAN_POINT('Ctrl Pts',(-1.77394167108292,1.,0.757578264077029));
#32204=CARTESIAN_POINT('Ctrl Pts',(-1.76789396002998,-1.,0.75642189602781));
#32205=CARTESIAN_POINT('Ctrl Pts',(-1.76789396002998,1.,0.75642189602781));
#32206=CARTESIAN_POINT('Ctrl Pts',(-1.76197817240128,-1.,0.755220979974461));
#32207=CARTESIAN_POINT('Ctrl Pts',(-1.76197817240128,1.,0.755220979974461));
#32208=CARTESIAN_POINT('Ctrl Pts',(-1.75631083600019,-1.,0.754009254027829));
#32209=CARTESIAN_POINT('Ctrl Pts',(-1.75631083600019,1.,0.754009254027829));
#32210=CARTESIAN_POINT('Ctrl Pts',(-1.75095139468794,-1.,0.752797683531314));
#32211=CARTESIAN_POINT('Ctrl Pts',(-1.75095139468794,1.,0.752797683531314));
#32212=CARTESIAN_POINT('Ctrl Pts',(-1.74585086852502,-1.,0.751555614164482));
#32213=CARTESIAN_POINT('Ctrl Pts',(-1.74585086852502,1.,0.751555614164482));
#32214=CARTESIAN_POINT('Ctrl Pts',(-1.74080458267114,-1.,0.750193435981249));
#32215=CARTESIAN_POINT('Ctrl Pts',(-1.74080458267114,1.,0.750193435981249));
#32216=CARTESIAN_POINT('Ctrl Pts',(-1.7355035168033,-1.,0.74858246295687));
#32217=CARTESIAN_POINT('Ctrl Pts',(-1.7355035168033,1.,0.74858246295687));
#32218=CARTESIAN_POINT('Ctrl Pts',(-1.72958533647714,-1.,0.746574710097752));
#32219=CARTESIAN_POINT('Ctrl Pts',(-1.72958533647714,1.,0.746574710097752));
#32220=CARTESIAN_POINT('Ctrl Pts',(-1.72268229916769,-1.,0.744021445433093));
#32221=CARTESIAN_POINT('Ctrl Pts',(-1.72268229916769,1.,0.744021445433093));
#32222=CARTESIAN_POINT('Ctrl Pts',(-1.71447789751001,-1.,0.74079516202821));
#32223=CARTESIAN_POINT('Ctrl Pts',(-1.71447789751001,1.,0.74079516202821));
#32224=CARTESIAN_POINT('Ctrl Pts',(-1.70473309004249,-1.,0.736799665716932));
#32225=CARTESIAN_POINT('Ctrl Pts',(-1.70473309004249,1.,0.736799665716932));
#32226=CARTESIAN_POINT('Ctrl Pts',(-1.69326921972915,-1.,0.731963238685357));
#32227=CARTESIAN_POINT('Ctrl Pts',(-1.69326921972915,1.,0.731963238685357));
#32228=CARTESIAN_POINT('Ctrl Pts',(-1.67996158451922,-1.,0.726235967982445));
#32229=CARTESIAN_POINT('Ctrl Pts',(-1.67996158451922,1.,0.726235967982445));
#32230=CARTESIAN_POINT('Ctrl Pts',(-1.66472880551777,-1.,0.71958543378795));
#32231=CARTESIAN_POINT('Ctrl Pts',(-1.66472880551777,1.,0.71958543378795));
#32232=CARTESIAN_POINT('Ctrl Pts',(-1.64752408828442,-1.,0.711993139340447));
#32233=CARTESIAN_POINT('Ctrl Pts',(-1.64752408828442,1.,0.711993139340447));
#32234=CARTESIAN_POINT('Ctrl Pts',(-1.6321654166204,-1.,0.705159151977294));
#32235=CARTESIAN_POINT('Ctrl Pts',(-1.6321654166204,1.,0.705159151977294));
#32236=CARTESIAN_POINT('Ctrl Pts',(-1.61974673471117,-1.,0.699605146398837));
#32237=CARTESIAN_POINT('Ctrl Pts',(-1.61974673471117,1.,0.699605146398837));
#32238=CARTESIAN_POINT('Ctrl Pts',(-1.61106790957619,-1.,0.69571209787897));
#32239=CARTESIAN_POINT('Ctrl Pts',(-1.61106790957619,1.,0.69571209787897));
#32240=CARTESIAN_POINT('Ctrl Pts',(-1.60662857109684,-1.,0.693717979106305));
#32241=CARTESIAN_POINT('Ctrl Pts',(-1.60662857109684,1.,0.693717979106305));
#32242=CARTESIAN_POINT('',(-2.0698113262342,1.,0.7455743247944));
#32243=CARTESIAN_POINT('Ctrl Pts',(-2.0698113262342,1.,0.7455743247944));
#32244=CARTESIAN_POINT('Ctrl Pts',(-2.06854248895728,1.,0.745832791378367));
#32245=CARTESIAN_POINT('Ctrl Pts',(-2.06600523016815,1.,0.7463458715442));
#32246=CARTESIAN_POINT('Ctrl Pts',(-2.06220058927826,1.,0.747103932787919));
#32247=CARTESIAN_POINT('Ctrl Pts',(-2.05713023031006,1.,0.748091554183802));
#32248=CARTESIAN_POINT('Ctrl Pts',(-2.05079645592154,1.,0.749287468665046));
#32249=CARTESIAN_POINT('Ctrl Pts',(-2.04446689147979,1.,0.750444657875576));
#32250=CARTESIAN_POINT('Ctrl Pts',(-2.03814160092099,1.,0.751562963361115));
#32251=CARTESIAN_POINT('Ctrl Pts',(-2.03182068456221,1.,0.752642180487211));
#32252=CARTESIAN_POINT('Ctrl Pts',(-2.02550428623313,1.,0.753682061112768));
#32253=CARTESIAN_POINT('Ctrl Pts',(-2.01919259405809,1.,0.754682330722816));
#32254=CARTESIAN_POINT('Ctrl Pts',(-2.01288584328084,1.,0.755642704957865));
#32255=CARTESIAN_POINT('Ctrl Pts',(-2.0065843158773,1.,0.75656290464667));
#32256=CARTESIAN_POINT('Ctrl Pts',(-2.00028834739178,1.,0.757442676862724));
#32257=CARTESIAN_POINT('Ctrl Pts',(-1.99399831098817,1.,0.758281796766761));
#32258=CARTESIAN_POINT('Ctrl Pts',(-1.98771456680874,1.,0.759080037802488));
#32259=CARTESIAN_POINT('Ctrl Pts',(-1.98143741418172,1.,0.75983714745219));
#32260=CARTESIAN_POINT('Ctrl Pts',(-1.97516705321494,1.,0.760552825409757));
#32261=CARTESIAN_POINT('Ctrl Pts',(-1.96890351582499,1.,0.76122669048382));
#32262=CARTESIAN_POINT('Ctrl Pts',(-1.96264672744186,1.,0.761858300014423));
#32263=CARTESIAN_POINT('Ctrl Pts',(-1.95639665309869,1.,0.762447203806179));
#32264=CARTESIAN_POINT('Ctrl Pts',(-1.95015342590024,1.,0.762992990878769));
#32265=CARTESIAN_POINT('Ctrl Pts',(-1.9439174661764,1.,0.763495333538629));
#32266=CARTESIAN_POINT('Ctrl Pts',(-1.93768964875886,1.,0.763954049121458));
#32267=CARTESIAN_POINT('Ctrl Pts',(-1.93147105496382,1.,0.76436901067394));
#32268=CARTESIAN_POINT('Ctrl Pts',(-1.92526263537048,1.,0.764740025488211));
#32269=CARTESIAN_POINT('Ctrl Pts',(-1.91906491634196,1.,0.765066729667088));
#32270=CARTESIAN_POINT('Ctrl Pts',(-1.91287765805169,1.,0.765348465884722));
#32271=CARTESIAN_POINT('Ctrl Pts',(-1.90669961402356,1.,0.765584196937919));
#32272=CARTESIAN_POINT('Ctrl Pts',(-1.90052930393596,1.,0.765772772593386));
#32273=CARTESIAN_POINT('Ctrl Pts',(-1.89436577771388,1.,0.765913193856978));
#32274=CARTESIAN_POINT('Ctrl Pts',(-1.88820926433409,1.,0.766004837062091));
#32275=CARTESIAN_POINT('Ctrl Pts',(-1.88206215302561,1.,0.766047794851864));
#32276=CARTESIAN_POINT('Ctrl Pts',(-1.87592888967883,1.,0.766042837036744));
#32277=CARTESIAN_POINT('Ctrl Pts',(-1.86981398314341,1.,0.765990708546091));
#32278=CARTESIAN_POINT('Ctrl Pts',(-1.86372027063312,1.,0.765891519092547));
#32279=CARTESIAN_POINT('Ctrl Pts',(-1.85764741390394,1.,0.765744212909318));
#32280=CARTESIAN_POINT('Ctrl Pts',(-1.85158945130063,1.,0.765545710619062));
#32281=CARTESIAN_POINT('Ctrl Pts',(-1.84553698875924,1.,0.765291664862029));
#32282=CARTESIAN_POINT('Ctrl Pts',(-1.83948181064835,1.,0.764978057881737));
#32283=CARTESIAN_POINT('Ctrl Pts',(-1.83342077227142,1.,0.764602549687853));
#32284=CARTESIAN_POINT('Ctrl Pts',(-1.82735991200065,1.,0.764165902605995));
#32285=CARTESIAN_POINT('Ctrl Pts',(-1.82131873145266,1.,0.763673465462726));
#32286=CARTESIAN_POINT('Ctrl Pts',(-1.8153211840553,1.,0.763132003836634));
#32287=CARTESIAN_POINT('Ctrl Pts',(-1.80938551463965,1.,0.762546129463938));
#32288=CARTESIAN_POINT('Ctrl Pts',(-1.80351583877342,1.,0.761915336443547));
#32289=CARTESIAN_POINT('Ctrl Pts',(-1.79768986997783,1.,0.761229695230558));
#32290=CARTESIAN_POINT('Ctrl Pts',(-1.7918581561088,1.,0.760469555880749));
#32291=CARTESIAN_POINT('Ctrl Pts',(-1.78596964884604,1.,0.759614401110189));
#32292=CARTESIAN_POINT('Ctrl Pts',(-1.77999411220945,1.,0.758650626677518));
#32293=CARTESIAN_POINT('Ctrl Pts',(-1.77394167108292,1.,0.757578264077029));
#32294=CARTESIAN_POINT('Ctrl Pts',(-1.76789396002998,1.,0.75642189602781));
#32295=CARTESIAN_POINT('Ctrl Pts',(-1.76197817240128,1.,0.755220979974461));
#32296=CARTESIAN_POINT('Ctrl Pts',(-1.75631083600019,1.,0.754009254027829));
#32297=CARTESIAN_POINT('Ctrl Pts',(-1.75095139468794,1.,0.752797683531314));
#32298=CARTESIAN_POINT('Ctrl Pts',(-1.74585086852502,1.,0.751555614164482));
#32299=CARTESIAN_POINT('Ctrl Pts',(-1.74080458267114,1.,0.750193435981249));
#32300=CARTESIAN_POINT('Ctrl Pts',(-1.7355035168033,1.,0.74858246295687));
#32301=CARTESIAN_POINT('Ctrl Pts',(-1.72958533647714,1.,0.746574710097752));
#32302=CARTESIAN_POINT('Ctrl Pts',(-1.72268229916769,1.,0.744021445433093));
#32303=CARTESIAN_POINT('Ctrl Pts',(-1.71447789751001,1.,0.74079516202821));
#32304=CARTESIAN_POINT('Ctrl Pts',(-1.70473309004249,1.,0.736799665716932));
#32305=CARTESIAN_POINT('Ctrl Pts',(-1.69326921972915,1.,0.731963238685357));
#32306=CARTESIAN_POINT('Ctrl Pts',(-1.67996158451922,1.,0.726235967982445));
#32307=CARTESIAN_POINT('Ctrl Pts',(-1.66472880551777,1.,0.71958543378795));
#32308=CARTESIAN_POINT('Ctrl Pts',(-1.64752408828442,1.,0.711993139340447));
#32309=CARTESIAN_POINT('Ctrl Pts',(-1.6321654166204,1.,0.705159151977294));
#32310=CARTESIAN_POINT('Ctrl Pts',(-1.61974673471117,1.,0.699605146398837));
#32311=CARTESIAN_POINT('Ctrl Pts',(-1.61106790957619,1.,0.69571209787897));
#32312=CARTESIAN_POINT('Ctrl Pts',(-1.60662857109684,1.,0.693717979106305));
#32313=CARTESIAN_POINT('',(-2.0698113262342,0.,0.7455743247944));
#32314=CARTESIAN_POINT('Origin',(-2.11275013067528,0.,0.61342227326009));
#32315=CARTESIAN_POINT('',(-2.11275013067528,1.,0.61342227326009));
#32316=CARTESIAN_POINT('',(-2.0698113262342,1.,0.7455743247944));
#32317=CARTESIAN_POINT('',(-2.11275013067528,0.,0.61342227326009));
#32318=CARTESIAN_POINT('Ctrl Pts',(-1.7075470150345,-1.,0.383122945602004));
#32319=CARTESIAN_POINT('Ctrl Pts',(-1.7075470150345,1.,0.383122945602004));
#32320=CARTESIAN_POINT('Ctrl Pts',(-1.71231062891958,-1.,0.384119047315542));
#32321=CARTESIAN_POINT('Ctrl Pts',(-1.71231062891958,1.,0.384119047315542));
#32322=CARTESIAN_POINT('Ctrl Pts',(-1.72162022246158,-1.,0.38607079032701));
#32323=CARTESIAN_POINT('Ctrl Pts',(-1.72162022246158,1.,0.38607079032701));
#32324=CARTESIAN_POINT('Ctrl Pts',(-1.7349317097561,-1.,0.388877023509191));
#32325=CARTESIAN_POINT('Ctrl Pts',(-1.7349317097561,1.,0.388877023509191));
#32326=CARTESIAN_POINT('Ctrl Pts',(-1.75137405313962,-1.,0.392375812294307));
#32327=CARTESIAN_POINT('Ctrl Pts',(-1.75137405313962,1.,0.392375812294307));
#32328=CARTESIAN_POINT('Ctrl Pts',(-1.7697556004756,-1.,0.39634619612042));
#32329=CARTESIAN_POINT('Ctrl Pts',(-1.7697556004756,1.,0.39634619612042));
#32330=CARTESIAN_POINT('Ctrl Pts',(-1.78598826347533,-1.,0.39991940378308));
#32331=CARTESIAN_POINT('Ctrl Pts',(-1.78598826347533,1.,0.39991940378308));
#32332=CARTESIAN_POINT('Ctrl Pts',(-1.80012077176221,-1.,0.403107976170441));
#32333=CARTESIAN_POINT('Ctrl Pts',(-1.80012077176221,1.,0.403107976170441));
#32334=CARTESIAN_POINT('Ctrl Pts',(-1.81223801813988,-1.,0.405933518411838));
#32335=CARTESIAN_POINT('Ctrl Pts',(-1.81223801813988,1.,0.405933518411838));
#32336=CARTESIAN_POINT('Ctrl Pts',(-1.8224702267854,-1.,0.408428948108533));
#32337=CARTESIAN_POINT('Ctrl Pts',(-1.8224702267854,1.,0.408428948108533));
#32338=CARTESIAN_POINT('Ctrl Pts',(-1.83100408895216,-1.,0.410641256301675));
#32339=CARTESIAN_POINT('Ctrl Pts',(-1.83100408895216,1.,0.410641256301675));
#32340=CARTESIAN_POINT('Ctrl Pts',(-1.83808953475839,-1.,0.412633125322161));
#32341=CARTESIAN_POINT('Ctrl Pts',(-1.83808953475839,1.,0.412633125322161));
#32342=CARTESIAN_POINT('Ctrl Pts',(-1.8440575707371,-1.,0.41448743825434));
#32343=CARTESIAN_POINT('Ctrl Pts',(-1.8440575707371,1.,0.41448743825434));
#32344=CARTESIAN_POINT('Ctrl Pts',(-1.84929312929882,-1.,0.416300022038864));
#32345=CARTESIAN_POINT('Ctrl Pts',(-1.84929312929882,1.,0.416300022038864));
#32346=CARTESIAN_POINT('Ctrl Pts',(-1.85417632856234,-1.,0.418164129143534));
#32347=CARTESIAN_POINT('Ctrl Pts',(-1.85417632856234,1.,0.418164129143534));
#32348=CARTESIAN_POINT('Ctrl Pts',(-1.85903281096686,-1.,0.420157287975619));
#32349=CARTESIAN_POINT('Ctrl Pts',(-1.85903281096686,1.,0.420157287975619));
#32350=CARTESIAN_POINT('Ctrl Pts',(-1.86408083334028,-1.,0.422327307418275));
#32351=CARTESIAN_POINT('Ctrl Pts',(-1.86408083334028,1.,0.422327307418275));
#32352=CARTESIAN_POINT('Ctrl Pts',(-1.86937803944323,-1.,0.424678177291359));
#32353=CARTESIAN_POINT('Ctrl Pts',(-1.86937803944323,1.,0.424678177291359));
#32354=CARTESIAN_POINT('Ctrl Pts',(-1.87486989291484,-1.,0.427183828519102));
#32355=CARTESIAN_POINT('Ctrl Pts',(-1.87486989291484,1.,0.427183828519102));
#32356=CARTESIAN_POINT('Ctrl Pts',(-1.88044229001832,-1.,0.429803062482344));
#32357=CARTESIAN_POINT('Ctrl Pts',(-1.88044229001832,1.,0.429803062482344));
#32358=CARTESIAN_POINT('Ctrl Pts',(-1.88596913666793,-1.,0.432493038548748));
#32359=CARTESIAN_POINT('Ctrl Pts',(-1.88596913666793,1.,0.432493038548748));
#32360=CARTESIAN_POINT('Ctrl Pts',(-1.89136993975504,-1.,0.435225660963383));
#32361=CARTESIAN_POINT('Ctrl Pts',(-1.89136993975504,1.,0.435225660963383));
#32362=CARTESIAN_POINT('Ctrl Pts',(-1.89663648956466,-1.,0.437995003948244));
#32363=CARTESIAN_POINT('Ctrl Pts',(-1.89663648956466,1.,0.437995003948244));
#32364=CARTESIAN_POINT('Ctrl Pts',(-1.90180124389086,-1.,0.440807833704038));
#32365=CARTESIAN_POINT('Ctrl Pts',(-1.90180124389086,1.,0.440807833704038));
#32366=CARTESIAN_POINT('Ctrl Pts',(-1.90691756144898,-1.,0.44367755684915));
#32367=CARTESIAN_POINT('Ctrl Pts',(-1.90691756144898,1.,0.44367755684915));
#32368=CARTESIAN_POINT('Ctrl Pts',(-1.9120369998112,-1.,0.446617343485711));
#32369=CARTESIAN_POINT('Ctrl Pts',(-1.9120369998112,1.,0.446617343485711));
#32370=CARTESIAN_POINT('Ctrl Pts',(-1.91718342555755,-1.,0.449632260106662));
#32371=CARTESIAN_POINT('Ctrl Pts',(-1.91718342555755,1.,0.449632260106662));
#32372=CARTESIAN_POINT('Ctrl Pts',(-1.92235380648502,-1.,0.452719478359432));
#32373=CARTESIAN_POINT('Ctrl Pts',(-1.92235380648502,1.,0.452719478359432));
#32374=CARTESIAN_POINT('Ctrl Pts',(-1.92753067150476,-1.,0.455872005174371));
#32375=CARTESIAN_POINT('Ctrl Pts',(-1.92753067150476,1.,0.455872005174371));
#32376=CARTESIAN_POINT('Ctrl Pts',(-1.93269066517934,-1.,0.459081234547926));
#32377=CARTESIAN_POINT('Ctrl Pts',(-1.93269066517934,1.,0.459081234547926));
#32378=CARTESIAN_POINT('Ctrl Pts',(-1.93781486640821,-1.,0.462340031009056));
#32379=CARTESIAN_POINT('Ctrl Pts',(-1.93781486640821,1.,0.462340031009056));
#32380=CARTESIAN_POINT('Ctrl Pts',(-1.9428979419619,-1.,0.46564546202603));
#32381=CARTESIAN_POINT('Ctrl Pts',(-1.9428979419619,1.,0.46564546202603));
#32382=CARTESIAN_POINT('Ctrl Pts',(-1.94794381136514,-1.,0.468997482913135));
#32383=CARTESIAN_POINT('Ctrl Pts',(-1.94794381136514,1.,0.468997482913135));
#32384=CARTESIAN_POINT('Ctrl Pts',(-1.95296148278133,-1.,0.472397672264072));
#32385=CARTESIAN_POINT('Ctrl Pts',(-1.95296148278133,1.,0.472397672264072));
#32386=CARTESIAN_POINT('Ctrl Pts',(-1.95796111148177,-1.,0.475848034683176));
#32387=CARTESIAN_POINT('Ctrl Pts',(-1.95796111148177,1.,0.475848034683176));
#32388=CARTESIAN_POINT('Ctrl Pts',(-1.96294933055943,-1.,0.479349583074855));
#32389=CARTESIAN_POINT('Ctrl Pts',(-1.96294933055943,1.,0.479349583074855));
#32390=CARTESIAN_POINT('Ctrl Pts',(-1.96792703422362,-1.,0.48290166212069));
#32391=CARTESIAN_POINT('Ctrl Pts',(-1.96792703422362,1.,0.48290166212069));
#32392=CARTESIAN_POINT('Ctrl Pts',(-1.97289186263272,-1.,0.486502692907659));
#32393=CARTESIAN_POINT('Ctrl Pts',(-1.97289186263272,1.,0.486502692907659));
#32394=CARTESIAN_POINT('Ctrl Pts',(-1.97783973019229,-1.,0.490150627860952));
#32395=CARTESIAN_POINT('Ctrl Pts',(-1.97783973019229,1.,0.490150627860952));
#32396=CARTESIAN_POINT('Ctrl Pts',(-1.98276658761821,-1.,0.493843476541494));
#32397=CARTESIAN_POINT('Ctrl Pts',(-1.98276658761821,1.,0.493843476541494));
#32398=CARTESIAN_POINT('Ctrl Pts',(-1.98767044752932,-1.,0.497579909545574));
#32399=CARTESIAN_POINT('Ctrl Pts',(-1.98767044752932,1.,0.497579909545574));
#32400=CARTESIAN_POINT('Ctrl Pts',(-1.99255149126155,-1.,0.501359287727146));
#32401=CARTESIAN_POINT('Ctrl Pts',(-1.99255149126155,1.,0.501359287727146));
#32402=CARTESIAN_POINT('Ctrl Pts',(-1.99741107463572,-1.,0.505181361323026));
#32403=CARTESIAN_POINT('Ctrl Pts',(-1.99741107463572,1.,0.505181361323026));
#32404=CARTESIAN_POINT('Ctrl Pts',(-2.00225107134734,-1.,0.509046069886157));
#32405=CARTESIAN_POINT('Ctrl Pts',(-2.00225107134734,1.,0.509046069886157));
#32406=CARTESIAN_POINT('Ctrl Pts',(-2.00707309946949,-1.,0.512953306961792));
#32407=CARTESIAN_POINT('Ctrl Pts',(-2.00707309946949,1.,0.512953306961792));
#32408=CARTESIAN_POINT('Ctrl Pts',(-2.01187773939242,-1.,0.516902681728687));
#32409=CARTESIAN_POINT('Ctrl Pts',(-2.01187773939242,1.,0.516902681728687));
#32410=CARTESIAN_POINT('Ctrl Pts',(-2.01666477917286,-1.,0.52089359039937));
#32411=CARTESIAN_POINT('Ctrl Pts',(-2.01666477917286,1.,0.52089359039937));
#32412=CARTESIAN_POINT('Ctrl Pts',(-2.02143356304698,-1.,0.524925318333476));
#32413=CARTESIAN_POINT('Ctrl Pts',(-2.02143356304698,1.,0.524925318333476));
#32414=CARTESIAN_POINT('Ctrl Pts',(-2.0261832908329,-1.,0.528997127241914));
#32415=CARTESIAN_POINT('Ctrl Pts',(-2.0261832908329,1.,0.528997127241914));
#32416=CARTESIAN_POINT('Ctrl Pts',(-2.03091336214426,-1.,0.533108355132976));
#32417=CARTESIAN_POINT('Ctrl Pts',(-2.03091336214426,1.,0.533108355132976));
#32418=CARTESIAN_POINT('Ctrl Pts',(-2.03562362954037,-1.,0.537258489833262));
#32419=CARTESIAN_POINT('Ctrl Pts',(-2.03562362954037,1.,0.537258489833262));
#32420=CARTESIAN_POINT('Ctrl Pts',(-2.04031422690527,-1.,0.541447120615659));
#32421=CARTESIAN_POINT('Ctrl Pts',(-2.04031422690527,1.,0.541447120615659));
#32422=CARTESIAN_POINT('Ctrl Pts',(-2.04498544714588,-1.,0.54567390381743));
#32423=CARTESIAN_POINT('Ctrl Pts',(-2.04498544714588,1.,0.54567390381743));
#32424=CARTESIAN_POINT('Ctrl Pts',(-2.04963761077958,-1.,0.549938525150295));
#32425=CARTESIAN_POINT('Ctrl Pts',(-2.04963761077958,1.,0.549938525150295));
#32426=CARTESIAN_POINT('Ctrl Pts',(-2.05427091604413,-1.,0.554240657463906));
#32427=CARTESIAN_POINT('Ctrl Pts',(-2.05427091604413,1.,0.554240657463906));
#32428=CARTESIAN_POINT('Ctrl Pts',(-2.05888537756462,-1.,0.558579940185151));
#32429=CARTESIAN_POINT('Ctrl Pts',(-2.05888537756462,1.,0.558579940185151));
#32430=CARTESIAN_POINT('Ctrl Pts',(-2.06348090160589,-1.,0.562955993082261));
#32431=CARTESIAN_POINT('Ctrl Pts',(-2.06348090160589,1.,0.562955993082261));
#32432=CARTESIAN_POINT('Ctrl Pts',(-2.06805732997334,-1.,0.567368421181087));
#32433=CARTESIAN_POINT('Ctrl Pts',(-2.06805732997334,1.,0.567368421181087));
#32434=CARTESIAN_POINT('Ctrl Pts',(-2.07261449292824,-1.,0.571816823242603));
#32435=CARTESIAN_POINT('Ctrl Pts',(-2.07261449292824,1.,0.571816823242603));
#32436=CARTESIAN_POINT('Ctrl Pts',(-2.07715226767559,-1.,0.576300797416844));
#32437=CARTESIAN_POINT('Ctrl Pts',(-2.07715226767559,1.,0.576300797416844));
#32438=CARTESIAN_POINT('Ctrl Pts',(-2.08167059018418,-1.,0.580819952108063));
#32439=CARTESIAN_POINT('Ctrl Pts',(-2.08167059018418,1.,0.580819952108063));
#32440=CARTESIAN_POINT('Ctrl Pts',(-2.08616943727951,-1.,0.585373918991617));
#32441=CARTESIAN_POINT('Ctrl Pts',(-2.08616943727951,1.,0.585373918991617));
#32442=CARTESIAN_POINT('Ctrl Pts',(-2.09064881812129,-1.,0.589962365403406));
#32443=CARTESIAN_POINT('Ctrl Pts',(-2.09064881812129,1.,0.589962365403406));
#32444=CARTESIAN_POINT('Ctrl Pts',(-2.0951087622027,-1.,0.594585006052162));
#32445=CARTESIAN_POINT('Ctrl Pts',(-2.0951087622027,1.,0.594585006052162));
#32446=CARTESIAN_POINT('Ctrl Pts',(-2.0995493086477,-1.,0.599241616420533));
#32447=CARTESIAN_POINT('Ctrl Pts',(-2.0995493086477,1.,0.599241616420533));
#32448=CARTESIAN_POINT('Ctrl Pts',(-2.10397049886949,-1.,0.60393203073603));
#32449=CARTESIAN_POINT('Ctrl Pts',(-2.10397049886949,1.,0.60393203073603));
#32450=CARTESIAN_POINT('Ctrl Pts',(-2.1074919961518,-1.,0.607711315454876));
#32451=CARTESIAN_POINT('Ctrl Pts',(-2.1074919961518,1.,0.607711315454876));
#32452=CARTESIAN_POINT('Ctrl Pts',(-2.11012443807238,-1.,0.610560911689899));
#32453=CARTESIAN_POINT('Ctrl Pts',(-2.11012443807238,1.,0.610560911689899));
#32454=CARTESIAN_POINT('Ctrl Pts',(-2.11187554259986,-1.,0.6124673655618));
#32455=CARTESIAN_POINT('Ctrl Pts',(-2.11187554259986,1.,0.6124673655618));
#32456=CARTESIAN_POINT('Ctrl Pts',(-2.11275013067528,-1.,0.61342227326009));
#32457=CARTESIAN_POINT('Ctrl Pts',(-2.11275013067528,1.,0.61342227326009));
#32458=CARTESIAN_POINT('',(-1.7075470150345,1.,0.383122945602004));
#32459=CARTESIAN_POINT('Ctrl Pts',(-1.7075470150345,1.,0.383122945602004));
#32460=CARTESIAN_POINT('Ctrl Pts',(-1.71231062891958,1.,0.384119047315542));
#32461=CARTESIAN_POINT('Ctrl Pts',(-1.72162022246158,1.,0.38607079032701));
#32462=CARTESIAN_POINT('Ctrl Pts',(-1.7349317097561,1.,0.388877023509191));
#32463=CARTESIAN_POINT('Ctrl Pts',(-1.75137405313962,1.,0.392375812294307));
#32464=CARTESIAN_POINT('Ctrl Pts',(-1.7697556004756,1.,0.39634619612042));
#32465=CARTESIAN_POINT('Ctrl Pts',(-1.78598826347533,1.,0.39991940378308));
#32466=CARTESIAN_POINT('Ctrl Pts',(-1.80012077176221,1.,0.403107976170441));
#32467=CARTESIAN_POINT('Ctrl Pts',(-1.81223801813988,1.,0.405933518411838));
#32468=CARTESIAN_POINT('Ctrl Pts',(-1.8224702267854,1.,0.408428948108533));
#32469=CARTESIAN_POINT('Ctrl Pts',(-1.83100408895216,1.,0.410641256301675));
#32470=CARTESIAN_POINT('Ctrl Pts',(-1.83808953475839,1.,0.412633125322161));
#32471=CARTESIAN_POINT('Ctrl Pts',(-1.8440575707371,1.,0.41448743825434));
#32472=CARTESIAN_POINT('Ctrl Pts',(-1.84929312929882,1.,0.416300022038864));
#32473=CARTESIAN_POINT('Ctrl Pts',(-1.85417632856234,1.,0.418164129143534));
#32474=CARTESIAN_POINT('Ctrl Pts',(-1.85903281096686,1.,0.420157287975619));
#32475=CARTESIAN_POINT('Ctrl Pts',(-1.86408083334028,1.,0.422327307418275));
#32476=CARTESIAN_POINT('Ctrl Pts',(-1.86937803944323,1.,0.424678177291359));
#32477=CARTESIAN_POINT('Ctrl Pts',(-1.87486989291484,1.,0.427183828519102));
#32478=CARTESIAN_POINT('Ctrl Pts',(-1.88044229001832,1.,0.429803062482344));
#32479=CARTESIAN_POINT('Ctrl Pts',(-1.88596913666793,1.,0.432493038548748));
#32480=CARTESIAN_POINT('Ctrl Pts',(-1.89136993975504,1.,0.435225660963383));
#32481=CARTESIAN_POINT('Ctrl Pts',(-1.89663648956466,1.,0.437995003948244));
#32482=CARTESIAN_POINT('Ctrl Pts',(-1.90180124389086,1.,0.440807833704038));
#32483=CARTESIAN_POINT('Ctrl Pts',(-1.90691756144898,1.,0.44367755684915));
#32484=CARTESIAN_POINT('Ctrl Pts',(-1.9120369998112,1.,0.446617343485711));
#32485=CARTESIAN_POINT('Ctrl Pts',(-1.91718342555755,1.,0.449632260106662));
#32486=CARTESIAN_POINT('Ctrl Pts',(-1.92235380648502,1.,0.452719478359432));
#32487=CARTESIAN_POINT('Ctrl Pts',(-1.92753067150476,1.,0.455872005174371));
#32488=CARTESIAN_POINT('Ctrl Pts',(-1.93269066517934,1.,0.459081234547926));
#32489=CARTESIAN_POINT('Ctrl Pts',(-1.93781486640821,1.,0.462340031009056));
#32490=CARTESIAN_POINT('Ctrl Pts',(-1.9428979419619,1.,0.46564546202603));
#32491=CARTESIAN_POINT('Ctrl Pts',(-1.94794381136514,1.,0.468997482913135));
#32492=CARTESIAN_POINT('Ctrl Pts',(-1.95296148278133,1.,0.472397672264072));
#32493=CARTESIAN_POINT('Ctrl Pts',(-1.95796111148177,1.,0.475848034683176));
#32494=CARTESIAN_POINT('Ctrl Pts',(-1.96294933055943,1.,0.479349583074855));
#32495=CARTESIAN_POINT('Ctrl Pts',(-1.96792703422362,1.,0.48290166212069));
#32496=CARTESIAN_POINT('Ctrl Pts',(-1.97289186263272,1.,0.486502692907659));
#32497=CARTESIAN_POINT('Ctrl Pts',(-1.97783973019229,1.,0.490150627860952));
#32498=CARTESIAN_POINT('Ctrl Pts',(-1.98276658761821,1.,0.493843476541494));
#32499=CARTESIAN_POINT('Ctrl Pts',(-1.98767044752932,1.,0.497579909545574));
#32500=CARTESIAN_POINT('Ctrl Pts',(-1.99255149126155,1.,0.501359287727146));
#32501=CARTESIAN_POINT('Ctrl Pts',(-1.99741107463572,1.,0.505181361323026));
#32502=CARTESIAN_POINT('Ctrl Pts',(-2.00225107134734,1.,0.509046069886157));
#32503=CARTESIAN_POINT('Ctrl Pts',(-2.00707309946949,1.,0.512953306961792));
#32504=CARTESIAN_POINT('Ctrl Pts',(-2.01187773939242,1.,0.516902681728687));
#32505=CARTESIAN_POINT('Ctrl Pts',(-2.01666477917286,1.,0.52089359039937));
#32506=CARTESIAN_POINT('Ctrl Pts',(-2.02143356304698,1.,0.524925318333476));
#32507=CARTESIAN_POINT('Ctrl Pts',(-2.0261832908329,1.,0.528997127241914));
#32508=CARTESIAN_POINT('Ctrl Pts',(-2.03091336214426,1.,0.533108355132976));
#32509=CARTESIAN_POINT('Ctrl Pts',(-2.03562362954037,1.,0.537258489833262));
#32510=CARTESIAN_POINT('Ctrl Pts',(-2.04031422690527,1.,0.541447120615659));
#32511=CARTESIAN_POINT('Ctrl Pts',(-2.04498544714588,1.,0.54567390381743));
#32512=CARTESIAN_POINT('Ctrl Pts',(-2.04963761077958,1.,0.549938525150295));
#32513=CARTESIAN_POINT('Ctrl Pts',(-2.05427091604413,1.,0.554240657463906));
#32514=CARTESIAN_POINT('Ctrl Pts',(-2.05888537756462,1.,0.558579940185151));
#32515=CARTESIAN_POINT('Ctrl Pts',(-2.06348090160589,1.,0.562955993082261));
#32516=CARTESIAN_POINT('Ctrl Pts',(-2.06805732997334,1.,0.567368421181087));
#32517=CARTESIAN_POINT('Ctrl Pts',(-2.07261449292824,1.,0.571816823242603));
#32518=CARTESIAN_POINT('Ctrl Pts',(-2.07715226767559,1.,0.576300797416844));
#32519=CARTESIAN_POINT('Ctrl Pts',(-2.08167059018418,1.,0.580819952108063));
#32520=CARTESIAN_POINT('Ctrl Pts',(-2.08616943727951,1.,0.585373918991617));
#32521=CARTESIAN_POINT('Ctrl Pts',(-2.09064881812129,1.,0.589962365403406));
#32522=CARTESIAN_POINT('Ctrl Pts',(-2.0951087622027,1.,0.594585006052162));
#32523=CARTESIAN_POINT('Ctrl Pts',(-2.0995493086477,1.,0.599241616420533));
#32524=CARTESIAN_POINT('Ctrl Pts',(-2.10397049886949,1.,0.60393203073603));
#32525=CARTESIAN_POINT('Ctrl Pts',(-2.1074919961518,1.,0.607711315454876));
#32526=CARTESIAN_POINT('Ctrl Pts',(-2.11012443807238,1.,0.610560911689899));
#32527=CARTESIAN_POINT('Ctrl Pts',(-2.11187554259986,1.,0.6124673655618));
#32528=CARTESIAN_POINT('Ctrl Pts',(-2.11275013067528,1.,0.61342227326009));
#32529=CARTESIAN_POINT('',(-1.7075470150345,0.,0.383122945602003));
#32530=CARTESIAN_POINT('Origin',(0.,0.,0.));
#32531=CARTESIAN_POINT('',(-1.74236521665491,1.,0.163289472382896));
#32532=CARTESIAN_POINT('Origin',(0.,1.,0.));
#32533=CARTESIAN_POINT('',(-1.74236521665491,0.,0.163289472382896));
#32534=CARTESIAN_POINT('Ctrl Pts',(-2.19890268624765,-1.,0.069476445021958));
#32535=CARTESIAN_POINT('Ctrl Pts',(-2.19890268624765,1.,0.069476445021958));
#32536=CARTESIAN_POINT('Ctrl Pts',(-2.19777582085423,-1.,0.0701143536325489));
#32537=CARTESIAN_POINT('Ctrl Pts',(-2.19777582085423,1.,0.0701143536325489));
#32538=CARTESIAN_POINT('Ctrl Pts',(-2.19552129484002,-1.,0.0713863779526153));
#32539=CARTESIAN_POINT('Ctrl Pts',(-2.19552129484002,1.,0.0713863779526153));
#32540=CARTESIAN_POINT('Ctrl Pts',(-2.19213712013662,-1.,0.0732830357306724));
#32541=CARTESIAN_POINT('Ctrl Pts',(-2.19213712013662,1.,0.0732830357306724));
#32542=CARTESIAN_POINT('Ctrl Pts',(-2.1876201139953,-1.,0.0757891465836146));
#32543=CARTESIAN_POINT('Ctrl Pts',(-2.1876201139953,1.,0.0757891465836146));
#32544=CARTESIAN_POINT('Ctrl Pts',(-2.18196589448887,-1.,0.0788837727685241));
#32545=CARTESIAN_POINT('Ctrl Pts',(-2.18196589448887,1.,0.0788837727685241));
#32546=CARTESIAN_POINT('Ctrl Pts',(-2.176303712113,-1.,0.0819402680872764));
#32547=CARTESIAN_POINT('Ctrl Pts',(-2.176303712113,1.,0.0819402680872764));
#32548=CARTESIAN_POINT('Ctrl Pts',(-2.17063357870952,-1.,0.0849584620835371));
#32549=CARTESIAN_POINT('Ctrl Pts',(-2.17063357870952,1.,0.0849584620835371));
#32550=CARTESIAN_POINT('Ctrl Pts',(-2.16495552645014,-1.,0.0879381291386921));
#32551=CARTESIAN_POINT('Ctrl Pts',(-2.16495552645014,1.,0.0879381291386921));
#32552=CARTESIAN_POINT('Ctrl Pts',(-2.15926961544516,-1.,0.0908789888107264));
#32553=CARTESIAN_POINT('Ctrl Pts',(-2.15926961544516,1.,0.0908789888107264));
#32554=CARTESIAN_POINT('Ctrl Pts',(-2.1535759397817,-1.,0.0937807218867642));
#32555=CARTESIAN_POINT('Ctrl Pts',(-2.1535759397817,1.,0.0937807218867642));
#32556=CARTESIAN_POINT('Ctrl Pts',(-2.14787463531795,-1.,0.0966429852305457));
#32557=CARTESIAN_POINT('Ctrl Pts',(-2.14787463531795,1.,0.0966429852305457));
#32558=CARTESIAN_POINT('Ctrl Pts',(-2.14216588396025,-1.,0.0994654261990914));
#32559=CARTESIAN_POINT('Ctrl Pts',(-2.14216588396025,1.,0.0994654261990914));
#32560=CARTESIAN_POINT('Ctrl Pts',(-2.13644992667165,-1.,0.1022477005561));
#32561=CARTESIAN_POINT('Ctrl Pts',(-2.13644992667165,1.,0.1022477005561));
#32562=CARTESIAN_POINT('Ctrl Pts',(-2.13072704887293,-1.,0.104989479152739));
#32563=CARTESIAN_POINT('Ctrl Pts',(-2.13072704887293,1.,0.104989479152739));
#32564=CARTESIAN_POINT('Ctrl Pts',(-2.12499752307,-1.,0.10769043523109));
#32565=CARTESIAN_POINT('Ctrl Pts',(-2.12499752307,1.,0.10769043523109));
#32566=CARTESIAN_POINT('Ctrl Pts',(-2.11926155590865,-1.,0.110350236135025));
#32567=CARTESIAN_POINT('Ctrl Pts',(-2.11926155590865,1.,0.110350236135025));
#32568=CARTESIAN_POINT('Ctrl Pts',(-2.11351924490306,-1.,0.112968534419737));
#32569=CARTESIAN_POINT('Ctrl Pts',(-2.11351924490306,1.,0.112968534419737));
#32570=CARTESIAN_POINT('Ctrl Pts',(-2.10777050261309,-1.,0.115544957687926));
#32571=CARTESIAN_POINT('Ctrl Pts',(-2.10777050261309,1.,0.115544957687926));
#32572=CARTESIAN_POINT('Ctrl Pts',(-2.102015121329,-1.,0.118079107988355));
#32573=CARTESIAN_POINT('Ctrl Pts',(-2.102015121329,1.,0.118079107988355));
#32574=CARTESIAN_POINT('Ctrl Pts',(-2.0962529286773,-1.,0.120570567965122));
#32575=CARTESIAN_POINT('Ctrl Pts',(-2.0962529286773,1.,0.120570567965122));
#32576=CARTESIAN_POINT('Ctrl Pts',(-2.09048392424825,-1.,0.123018905621083));
#32577=CARTESIAN_POINT('Ctrl Pts',(-2.09048392424825,1.,0.123018905621083));
#32578=CARTESIAN_POINT('Ctrl Pts',(-2.08470840653643,-1.,0.125423679412061));
#32579=CARTESIAN_POINT('Ctrl Pts',(-2.08470840653643,1.,0.125423679412061));
#32580=CARTESIAN_POINT('Ctrl Pts',(-2.07892715110987,-1.,0.12778444527612));
#32581=CARTESIAN_POINT('Ctrl Pts',(-2.07892715110987,1.,0.12778444527612));
#32582=CARTESIAN_POINT('Ctrl Pts',(-2.07314114713063,-1.,0.130100748328403));
#32583=CARTESIAN_POINT('Ctrl Pts',(-2.07314114713063,1.,0.130100748328403));
#32584=CARTESIAN_POINT('Ctrl Pts',(-2.06735123910326,-1.,0.13237211154771));
#32585=CARTESIAN_POINT('Ctrl Pts',(-2.06735123910326,1.,0.13237211154771));
#32586=CARTESIAN_POINT('Ctrl Pts',(-2.06155781517842,-1.,0.134598026192106));
#32587=CARTESIAN_POINT('Ctrl Pts',(-2.06155781517842,1.,0.134598026192106));
#32588=CARTESIAN_POINT('Ctrl Pts',(-2.05576044414264,-1.,0.136777941218043));
#32589=CARTESIAN_POINT('Ctrl Pts',(-2.05576044414264,1.,0.136777941218043));
#32590=CARTESIAN_POINT('Ctrl Pts',(-2.04995762001328,-1.,0.138911255368966));
#32591=CARTESIAN_POINT('Ctrl Pts',(-2.04995762001328,1.,0.138911255368966));
#32592=CARTESIAN_POINT('Ctrl Pts',(-2.04414757947916,-1.,0.140997332152546));
#32593=CARTESIAN_POINT('Ctrl Pts',(-2.04414757947916,1.,0.140997332152546));
#32594=CARTESIAN_POINT('Ctrl Pts',(-2.03832911025912,-1.,0.143035515058209));
#32595=CARTESIAN_POINT('Ctrl Pts',(-2.03832911025912,1.,0.143035515058209));
#32596=CARTESIAN_POINT('Ctrl Pts',(-2.03250223739942,-1.,0.145025140186057));
#32597=CARTESIAN_POINT('Ctrl Pts',(-2.03250223739942,1.,0.145025140186057));
#32598=CARTESIAN_POINT('Ctrl Pts',(-2.02666926182017,-1.,0.146965557332583));
#32599=CARTESIAN_POINT('Ctrl Pts',(-2.02666926182017,1.,0.146965557332583));
#32600=CARTESIAN_POINT('Ctrl Pts',(-2.02083464969894,-1.,0.148856124775337));
#32601=CARTESIAN_POINT('Ctrl Pts',(-2.02083464969894,1.,0.148856124775337));
#32602=CARTESIAN_POINT('Ctrl Pts',(-2.01500291940238,-1.,0.150696157673078));
#32603=CARTESIAN_POINT('Ctrl Pts',(-2.01500291940238,1.,0.150696157673078));
#32604=CARTESIAN_POINT('Ctrl Pts',(-2.00917680318424,-1.,0.15248488362145));
#32605=CARTESIAN_POINT('Ctrl Pts',(-2.00917680318424,1.,0.15248488362145));
#32606=CARTESIAN_POINT('Ctrl Pts',(-2.00335565310543,-1.,0.154221403049722));
#32607=CARTESIAN_POINT('Ctrl Pts',(-2.00335565310543,1.,0.154221403049722));
#32608=CARTESIAN_POINT('Ctrl Pts',(-1.99753284771497,-1.,0.155904629548783));
#32609=CARTESIAN_POINT('Ctrl Pts',(-1.99753284771497,1.,0.155904629548783));
#32610=CARTESIAN_POINT('Ctrl Pts',(-1.99169810931908,-1.,0.157533331459227));
#32611=CARTESIAN_POINT('Ctrl Pts',(-1.99169810931908,1.,0.157533331459227));
#32612=CARTESIAN_POINT('Ctrl Pts',(-1.98584238283292,-1.,0.159106226437299));
#32613=CARTESIAN_POINT('Ctrl Pts',(-1.98584238283292,1.,0.159106226437299));
#32614=CARTESIAN_POINT('Ctrl Pts',(-1.97996195437559,-1.,0.160622060784611));
#32615=CARTESIAN_POINT('Ctrl Pts',(-1.97996195437559,1.,0.160622060784611));
#32616=CARTESIAN_POINT('Ctrl Pts',(-1.97406280235188,-1.,0.162079693556288));
#32617=CARTESIAN_POINT('Ctrl Pts',(-1.97406280235188,1.,0.162079693556288));
#32618=CARTESIAN_POINT('Ctrl Pts',(-1.96816512677967,-1.,0.163478185457734));
#32619=CARTESIAN_POINT('Ctrl Pts',(-1.96816512677967,1.,0.163478185457734));
#32620=CARTESIAN_POINT('Ctrl Pts',(-1.96229379940136,-1.,0.164816568920269));
#32621=CARTESIAN_POINT('Ctrl Pts',(-1.96229379940136,1.,0.164816568920269));
#32622=CARTESIAN_POINT('Ctrl Pts',(-1.9564675971873,-1.,0.166093592002812));
#32623=CARTESIAN_POINT('Ctrl Pts',(-1.9564675971873,1.,0.166093592002812));
#32624=CARTESIAN_POINT('Ctrl Pts',(-1.95069027794294,-1.,0.167307501784475));
#32625=CARTESIAN_POINT('Ctrl Pts',(-1.95069027794294,1.,0.167307501784475));
#32626=CARTESIAN_POINT('Ctrl Pts',(-1.94493757756931,-1.,0.168455741607556));
#32627=CARTESIAN_POINT('Ctrl Pts',(-1.94493757756931,1.,0.168455741607556));
#32628=CARTESIAN_POINT('Ctrl Pts',(-1.93915639211581,-1.,0.169534904817491));
#32629=CARTESIAN_POINT('Ctrl Pts',(-1.93915639211581,1.,0.169534904817491));
#32630=CARTESIAN_POINT('Ctrl Pts',(-1.93329183155539,-1.,0.170541253116201));
#32631=CARTESIAN_POINT('Ctrl Pts',(-1.93329183155539,1.,0.170541253116201));
#32632=CARTESIAN_POINT('Ctrl Pts',(-1.92731093582036,-1.,0.171471191532988));
#32633=CARTESIAN_POINT('Ctrl Pts',(-1.92731093582036,1.,0.171471191532988));
#32634=CARTESIAN_POINT('Ctrl Pts',(-1.9212233439798,-1.,0.172321621259514));
#32635=CARTESIAN_POINT('Ctrl Pts',(-1.9212233439798,1.,0.172321621259514));
#32636=CARTESIAN_POINT('Ctrl Pts',(-1.91511429159527,-1.,0.173090695383496));
#32637=CARTESIAN_POINT('Ctrl Pts',(-1.91511429159527,1.,0.173090695383496));
#32638=CARTESIAN_POINT('Ctrl Pts',(-1.90911693975267,-1.,0.173776635257817));
#32639=CARTESIAN_POINT('Ctrl Pts',(-1.90911693975267,1.,0.173776635257817));
#32640=CARTESIAN_POINT('Ctrl Pts',(-1.90335253862834,-1.,0.174375518661085));
#32641=CARTESIAN_POINT('Ctrl Pts',(-1.90335253862834,1.,0.174375518661085));
#32642=CARTESIAN_POINT('Ctrl Pts',(-1.89788101117132,-1.,0.174879405091263));
#32643=CARTESIAN_POINT('Ctrl Pts',(-1.89788101117132,1.,0.174879405091263));
#32644=CARTESIAN_POINT('Ctrl Pts',(-1.892646301985,-1.,0.175274276190844));
#32645=CARTESIAN_POINT('Ctrl Pts',(-1.892646301985,1.,0.175274276190844));
#32646=CARTESIAN_POINT('Ctrl Pts',(-1.88742606273259,-1.,0.175538155840648));
#32647=CARTESIAN_POINT('Ctrl Pts',(-1.88742606273259,1.,0.175538155840648));
#32648=CARTESIAN_POINT('Ctrl Pts',(-1.88188663145367,-1.,0.175644148889698));
#32649=CARTESIAN_POINT('Ctrl Pts',(-1.88188663145367,1.,0.175644148889698));
#32650=CARTESIAN_POINT('Ctrl Pts',(-1.87563767773588,-1.,0.175563480746485));
#32651=CARTESIAN_POINT('Ctrl Pts',(-1.87563767773588,1.,0.175563480746485));
#32652=CARTESIAN_POINT('Ctrl Pts',(-1.86828349694799,-1.,0.175268337590758));
#32653=CARTESIAN_POINT('Ctrl Pts',(-1.86828349694799,1.,0.175268337590758));
#32654=CARTESIAN_POINT('Ctrl Pts',(-1.85948367088837,-1.,0.17473525927603));
#32655=CARTESIAN_POINT('Ctrl Pts',(-1.85948367088837,1.,0.17473525927603));
#32656=CARTESIAN_POINT('Ctrl Pts',(-1.8489811319852,-1.,0.173946627587731));
#32657=CARTESIAN_POINT('Ctrl Pts',(-1.8489811319852,1.,0.173946627587731));
#32658=CARTESIAN_POINT('Ctrl Pts',(-1.83658380527692,-1.,0.1728894428919));
#32659=CARTESIAN_POINT('Ctrl Pts',(-1.83658380527692,1.,0.1728894428919));
#32660=CARTESIAN_POINT('Ctrl Pts',(-1.82215766811545,-1.,0.171554770204119));
#32661=CARTESIAN_POINT('Ctrl Pts',(-1.82215766811545,1.,0.171554770204119));
#32662=CARTESIAN_POINT('Ctrl Pts',(-1.80561530629706,-1.,0.169936923904608));
#32663=CARTESIAN_POINT('Ctrl Pts',(-1.80561530629706,1.,0.169936923904608));
#32664=CARTESIAN_POINT('Ctrl Pts',(-1.7869064998507,-1.,0.168032772805197));
#32665=CARTESIAN_POINT('Ctrl Pts',(-1.7869064998507,1.,0.168032772805197));
#32666=CARTESIAN_POINT('Ctrl Pts',(-1.77018771684844,-1.,0.1662793551464));
#32667=CARTESIAN_POINT('Ctrl Pts',(-1.77018771684844,1.,0.1662793551464));
#32668=CARTESIAN_POINT('Ctrl Pts',(-1.75666056638427,-1.,0.164834765707158));
#32669=CARTESIAN_POINT('Ctrl Pts',(-1.75666056638427,1.,0.164834765707158));
#32670=CARTESIAN_POINT('Ctrl Pts',(-1.7472034950333,-1.,0.163814161002002));
#32671=CARTESIAN_POINT('Ctrl Pts',(-1.7472034950333,1.,0.163814161002002));
#32672=CARTESIAN_POINT('Ctrl Pts',(-1.74236521665491,-1.,0.163289472382896));
#32673=CARTESIAN_POINT('Ctrl Pts',(-1.74236521665491,1.,0.163289472382896));
#32674=CARTESIAN_POINT('',(-2.19890268624765,1.,0.069476445021958));
#32675=CARTESIAN_POINT('Ctrl Pts',(-2.19890268624765,1.,0.069476445021958));
#32676=CARTESIAN_POINT('Ctrl Pts',(-2.19777582085423,1.,0.0701143536325489));
#32677=CARTESIAN_POINT('Ctrl Pts',(-2.19552129484002,1.,0.0713863779526153));
#32678=CARTESIAN_POINT('Ctrl Pts',(-2.19213712013662,1.,0.0732830357306724));
#32679=CARTESIAN_POINT('Ctrl Pts',(-2.1876201139953,1.,0.0757891465836146));
#32680=CARTESIAN_POINT('Ctrl Pts',(-2.18196589448887,1.,0.0788837727685241));
#32681=CARTESIAN_POINT('Ctrl Pts',(-2.176303712113,1.,0.0819402680872764));
#32682=CARTESIAN_POINT('Ctrl Pts',(-2.17063357870952,1.,0.0849584620835371));
#32683=CARTESIAN_POINT('Ctrl Pts',(-2.16495552645014,1.,0.0879381291386921));
#32684=CARTESIAN_POINT('Ctrl Pts',(-2.15926961544516,1.,0.0908789888107264));
#32685=CARTESIAN_POINT('Ctrl Pts',(-2.1535759397817,1.,0.0937807218867642));
#32686=CARTESIAN_POINT('Ctrl Pts',(-2.14787463531795,1.,0.0966429852305457));
#32687=CARTESIAN_POINT('Ctrl Pts',(-2.14216588396025,1.,0.0994654261990914));
#32688=CARTESIAN_POINT('Ctrl Pts',(-2.13644992667165,1.,0.1022477005561));
#32689=CARTESIAN_POINT('Ctrl Pts',(-2.13072704887293,1.,0.104989479152739));
#32690=CARTESIAN_POINT('Ctrl Pts',(-2.12499752307,1.,0.10769043523109));
#32691=CARTESIAN_POINT('Ctrl Pts',(-2.11926155590865,1.,0.110350236135025));
#32692=CARTESIAN_POINT('Ctrl Pts',(-2.11351924490306,1.,0.112968534419737));
#32693=CARTESIAN_POINT('Ctrl Pts',(-2.10777050261309,1.,0.115544957687926));
#32694=CARTESIAN_POINT('Ctrl Pts',(-2.102015121329,1.,0.118079107988355));
#32695=CARTESIAN_POINT('Ctrl Pts',(-2.0962529286773,1.,0.120570567965122));
#32696=CARTESIAN_POINT('Ctrl Pts',(-2.09048392424825,1.,0.123018905621083));
#32697=CARTESIAN_POINT('Ctrl Pts',(-2.08470840653643,1.,0.125423679412061));
#32698=CARTESIAN_POINT('Ctrl Pts',(-2.07892715110987,1.,0.12778444527612));
#32699=CARTESIAN_POINT('Ctrl Pts',(-2.07314114713063,1.,0.130100748328403));
#32700=CARTESIAN_POINT('Ctrl Pts',(-2.06735123910326,1.,0.13237211154771));
#32701=CARTESIAN_POINT('Ctrl Pts',(-2.06155781517842,1.,0.134598026192106));
#32702=CARTESIAN_POINT('Ctrl Pts',(-2.05576044414264,1.,0.136777941218043));
#32703=CARTESIAN_POINT('Ctrl Pts',(-2.04995762001328,1.,0.138911255368966));
#32704=CARTESIAN_POINT('Ctrl Pts',(-2.04414757947916,1.,0.140997332152546));
#32705=CARTESIAN_POINT('Ctrl Pts',(-2.03832911025912,1.,0.143035515058209));
#32706=CARTESIAN_POINT('Ctrl Pts',(-2.03250223739942,1.,0.145025140186057));
#32707=CARTESIAN_POINT('Ctrl Pts',(-2.02666926182017,1.,0.146965557332583));
#32708=CARTESIAN_POINT('Ctrl Pts',(-2.02083464969894,1.,0.148856124775337));
#32709=CARTESIAN_POINT('Ctrl Pts',(-2.01500291940238,1.,0.150696157673078));
#32710=CARTESIAN_POINT('Ctrl Pts',(-2.00917680318424,1.,0.15248488362145));
#32711=CARTESIAN_POINT('Ctrl Pts',(-2.00335565310543,1.,0.154221403049722));
#32712=CARTESIAN_POINT('Ctrl Pts',(-1.99753284771497,1.,0.155904629548783));
#32713=CARTESIAN_POINT('Ctrl Pts',(-1.99169810931908,1.,0.157533331459227));
#32714=CARTESIAN_POINT('Ctrl Pts',(-1.98584238283292,1.,0.159106226437299));
#32715=CARTESIAN_POINT('Ctrl Pts',(-1.97996195437559,1.,0.160622060784611));
#32716=CARTESIAN_POINT('Ctrl Pts',(-1.97406280235188,1.,0.162079693556288));
#32717=CARTESIAN_POINT('Ctrl Pts',(-1.96816512677967,1.,0.163478185457734));
#32718=CARTESIAN_POINT('Ctrl Pts',(-1.96229379940136,1.,0.164816568920269));
#32719=CARTESIAN_POINT('Ctrl Pts',(-1.9564675971873,1.,0.166093592002812));
#32720=CARTESIAN_POINT('Ctrl Pts',(-1.95069027794294,1.,0.167307501784475));
#32721=CARTESIAN_POINT('Ctrl Pts',(-1.94493757756931,1.,0.168455741607556));
#32722=CARTESIAN_POINT('Ctrl Pts',(-1.93915639211581,1.,0.169534904817491));
#32723=CARTESIAN_POINT('Ctrl Pts',(-1.93329183155539,1.,0.170541253116201));
#32724=CARTESIAN_POINT('Ctrl Pts',(-1.92731093582036,1.,0.171471191532988));
#32725=CARTESIAN_POINT('Ctrl Pts',(-1.9212233439798,1.,0.172321621259514));
#32726=CARTESIAN_POINT('Ctrl Pts',(-1.91511429159527,1.,0.173090695383496));
#32727=CARTESIAN_POINT('Ctrl Pts',(-1.90911693975267,1.,0.173776635257817));
#32728=CARTESIAN_POINT('Ctrl Pts',(-1.90335253862834,1.,0.174375518661085));
#32729=CARTESIAN_POINT('Ctrl Pts',(-1.89788101117132,1.,0.174879405091263));
#32730=CARTESIAN_POINT('Ctrl Pts',(-1.892646301985,1.,0.175274276190844));
#32731=CARTESIAN_POINT('Ctrl Pts',(-1.88742606273259,1.,0.175538155840648));
#32732=CARTESIAN_POINT('Ctrl Pts',(-1.88188663145367,1.,0.175644148889698));
#32733=CARTESIAN_POINT('Ctrl Pts',(-1.87563767773588,1.,0.175563480746485));
#32734=CARTESIAN_POINT('Ctrl Pts',(-1.86828349694799,1.,0.175268337590758));
#32735=CARTESIAN_POINT('Ctrl Pts',(-1.85948367088837,1.,0.17473525927603));
#32736=CARTESIAN_POINT('Ctrl Pts',(-1.8489811319852,1.,0.173946627587731));
#32737=CARTESIAN_POINT('Ctrl Pts',(-1.83658380527692,1.,0.1728894428919));
#32738=CARTESIAN_POINT('Ctrl Pts',(-1.82215766811545,1.,0.171554770204119));
#32739=CARTESIAN_POINT('Ctrl Pts',(-1.80561530629706,1.,0.169936923904608));
#32740=CARTESIAN_POINT('Ctrl Pts',(-1.7869064998507,1.,0.168032772805197));
#32741=CARTESIAN_POINT('Ctrl Pts',(-1.77018771684844,1.,0.1662793551464));
#32742=CARTESIAN_POINT('Ctrl Pts',(-1.75666056638427,1.,0.164834765707158));
#32743=CARTESIAN_POINT('Ctrl Pts',(-1.7472034950333,1.,0.163814161002002));
#32744=CARTESIAN_POINT('Ctrl Pts',(-1.74236521665491,1.,0.163289472382896));
#32745=CARTESIAN_POINT('',(-2.19890268624765,0.,0.069476445021958));
#32746=CARTESIAN_POINT('Origin',(-2.19890268624765,0.,-0.0694764450219585));
#32747=CARTESIAN_POINT('',(-2.19890268624765,1.,-0.0694764450219585));
#32748=CARTESIAN_POINT('',(-2.19890268624765,1.,0.069476445021958));
#32749=CARTESIAN_POINT('',(-2.19890268624765,0.,-0.0694764450219585));
#32750=CARTESIAN_POINT('Ctrl Pts',(-1.74236521665491,-1.,-0.163289472382896));
#32751=CARTESIAN_POINT('Ctrl Pts',(-1.74236521665491,1.,-0.163289472382896));
#32752=CARTESIAN_POINT('Ctrl Pts',(-1.74720349503904,-1.,-0.163814161002474));
#32753=CARTESIAN_POINT('Ctrl Pts',(-1.74720349503904,1.,-0.163814161002474));
#32754=CARTESIAN_POINT('Ctrl Pts',(-1.75666056640041,-1.,-0.164834765708484));
#32755=CARTESIAN_POINT('Ctrl Pts',(-1.75666056640041,1.,-0.164834765708484));
#32756=CARTESIAN_POINT('Ctrl Pts',(-1.77018771687692,-1.,-0.166279355148738));
#32757=CARTESIAN_POINT('Ctrl Pts',(-1.77018771687692,1.,-0.166279355148738));
#32758=CARTESIAN_POINT('Ctrl Pts',(-1.78690649988931,-1.,-0.16803277280837));
#32759=CARTESIAN_POINT('Ctrl Pts',(-1.78690649988931,1.,-0.16803277280837));
#32760=CARTESIAN_POINT('Ctrl Pts',(-1.80561530633924,-1.,-0.169936923908078));
#32761=CARTESIAN_POINT('Ctrl Pts',(-1.80561530633924,1.,-0.169936923908078));
#32762=CARTESIAN_POINT('Ctrl Pts',(-1.82215766815414,-1.,-0.171554770207306));
#32763=CARTESIAN_POINT('Ctrl Pts',(-1.82215766815414,1.,-0.171554770207306));
#32764=CARTESIAN_POINT('Ctrl Pts',(-1.83658380530747,-1.,-0.17288944289442));
#32765=CARTESIAN_POINT('Ctrl Pts',(-1.83658380530747,1.,-0.17288944289442));
#32766=CARTESIAN_POINT('Ctrl Pts',(-1.84898113200543,-1.,-0.173946627589401));
#32767=CARTESIAN_POINT('Ctrl Pts',(-1.84898113200543,1.,-0.173946627589401));
#32768=CARTESIAN_POINT('Ctrl Pts',(-1.85948367089838,-1.,-0.174735259276856));
#32769=CARTESIAN_POINT('Ctrl Pts',(-1.85948367089838,1.,-0.174735259276856));
#32770=CARTESIAN_POINT('Ctrl Pts',(-1.86828349694972,-1.,-0.175268337590901));
#32771=CARTESIAN_POINT('Ctrl Pts',(-1.86828349694972,1.,-0.175268337590901));
#32772=CARTESIAN_POINT('Ctrl Pts',(-1.87563767773249,-1.,-0.175563480746205));
#32773=CARTESIAN_POINT('Ctrl Pts',(-1.87563767773249,1.,-0.175563480746205));
#32774=CARTESIAN_POINT('Ctrl Pts',(-1.88188663144846,-1.,-0.175644148889271));
#32775=CARTESIAN_POINT('Ctrl Pts',(-1.88188663144846,1.,-0.175644148889271));
#32776=CARTESIAN_POINT('Ctrl Pts',(-1.88742606272818,-1.,-0.175538155840286));
#32777=CARTESIAN_POINT('Ctrl Pts',(-1.88742606272818,1.,-0.175538155840286));
#32778=CARTESIAN_POINT('Ctrl Pts',(-1.89264630198279,-1.,-0.175274276190664));
#32779=CARTESIAN_POINT('Ctrl Pts',(-1.89264630198279,1.,-0.175274276190664));
#32780=CARTESIAN_POINT('Ctrl Pts',(-1.89788101117148,-1.,-0.174879405091277));
#32781=CARTESIAN_POINT('Ctrl Pts',(-1.89788101117148,1.,-0.174879405091277));
#32782=CARTESIAN_POINT('Ctrl Pts',(-1.90335253863003,-1.,-0.174375518661222));
#32783=CARTESIAN_POINT('Ctrl Pts',(-1.90335253863003,1.,-0.174375518661222));
#32784=CARTESIAN_POINT('Ctrl Pts',(-1.90911693975475,-1.,-0.173776635257984));
#32785=CARTESIAN_POINT('Ctrl Pts',(-1.90911693975475,1.,-0.173776635257984));
#32786=CARTESIAN_POINT('Ctrl Pts',(-1.91511429159681,-1.,-0.173090695383619));
#32787=CARTESIAN_POINT('Ctrl Pts',(-1.91511429159681,1.,-0.173090695383619));
#32788=CARTESIAN_POINT('Ctrl Pts',(-1.92122334398034,-1.,-0.172321621259557));
#32789=CARTESIAN_POINT('Ctrl Pts',(-1.92122334398034,1.,-0.172321621259557));
#32790=CARTESIAN_POINT('Ctrl Pts',(-1.92731093582,-1.,-0.17147119153296));
#32791=CARTESIAN_POINT('Ctrl Pts',(-1.92731093582,1.,-0.17147119153296));
#32792=CARTESIAN_POINT('Ctrl Pts',(-1.93329183155455,-1.,-0.170541253116136));
#32793=CARTESIAN_POINT('Ctrl Pts',(-1.93329183155455,1.,-0.170541253116136));
#32794=CARTESIAN_POINT('Ctrl Pts',(-1.93915639211497,-1.,-0.169534904817425));
#32795=CARTESIAN_POINT('Ctrl Pts',(-1.93915639211497,1.,-0.169534904817425));
#32796=CARTESIAN_POINT('Ctrl Pts',(-1.94493757756879,-1.,-0.168455741607516));
#32797=CARTESIAN_POINT('Ctrl Pts',(-1.94493757756879,1.,-0.168455741607516));
#32798=CARTESIAN_POINT('Ctrl Pts',(-1.95069027794286,-1.,-0.167307501784469));
#32799=CARTESIAN_POINT('Ctrl Pts',(-1.95069027794286,1.,-0.167307501784469));
#32800=CARTESIAN_POINT('Ctrl Pts',(-1.95646759718755,-1.,-0.166093592002833));
#32801=CARTESIAN_POINT('Ctrl Pts',(-1.95646759718755,1.,-0.166093592002833));
#32802=CARTESIAN_POINT('Ctrl Pts',(-1.96229379940174,-1.,-0.1648165689203));
#32803=CARTESIAN_POINT('Ctrl Pts',(-1.96229379940174,1.,-0.1648165689203));
#32804=CARTESIAN_POINT('Ctrl Pts',(-1.96816512678,-1.,-0.16347818545776));
#32805=CARTESIAN_POINT('Ctrl Pts',(-1.96816512678,1.,-0.16347818545776));
#32806=CARTESIAN_POINT('Ctrl Pts',(-1.97406280235204,-1.,-0.162079693556302));
#32807=CARTESIAN_POINT('Ctrl Pts',(-1.97406280235204,1.,-0.162079693556302));
#32808=CARTESIAN_POINT('Ctrl Pts',(-1.97996195437557,-1.,-0.16062206078461));
#32809=CARTESIAN_POINT('Ctrl Pts',(-1.97996195437557,1.,-0.16062206078461));
#32810=CARTESIAN_POINT('Ctrl Pts',(-1.98584238283279,-1.,-0.159106226437289));
#32811=CARTESIAN_POINT('Ctrl Pts',(-1.98584238283279,1.,-0.159106226437289));
#32812=CARTESIAN_POINT('Ctrl Pts',(-1.99169810931893,-1.,-0.157533331459215));
#32813=CARTESIAN_POINT('Ctrl Pts',(-1.99169810931893,1.,-0.157533331459215));
#32814=CARTESIAN_POINT('Ctrl Pts',(-1.99753284771487,-1.,-0.155904629548775));
#32815=CARTESIAN_POINT('Ctrl Pts',(-1.99753284771487,1.,-0.155904629548775));
#32816=CARTESIAN_POINT('Ctrl Pts',(-2.00335565310539,-1.,-0.154221403049719));
#32817=CARTESIAN_POINT('Ctrl Pts',(-2.00335565310539,1.,-0.154221403049719));
#32818=CARTESIAN_POINT('Ctrl Pts',(-2.00917680318426,-1.,-0.152484883621452));
#32819=CARTESIAN_POINT('Ctrl Pts',(-2.00917680318426,1.,-0.152484883621452));
#32820=CARTESIAN_POINT('Ctrl Pts',(-2.01500291940243,-1.,-0.150696157673084));
#32821=CARTESIAN_POINT('Ctrl Pts',(-2.01500291940243,1.,-0.150696157673084));
#32822=CARTESIAN_POINT('Ctrl Pts',(-2.02083464969897,-1.,-0.148856124775343));
#32823=CARTESIAN_POINT('Ctrl Pts',(-2.02083464969897,1.,-0.148856124775343));
#32824=CARTESIAN_POINT('Ctrl Pts',(-2.02666926182017,-1.,-0.146965557332586));
#32825=CARTESIAN_POINT('Ctrl Pts',(-2.02666926182017,1.,-0.146965557332586));
#32826=CARTESIAN_POINT('Ctrl Pts',(-2.03250223739941,-1.,-0.145025140186058));
#32827=CARTESIAN_POINT('Ctrl Pts',(-2.03250223739941,1.,-0.145025140186058));
#32828=CARTESIAN_POINT('Ctrl Pts',(-2.03832911025913,-1.,-0.143035515058208));
#32829=CARTESIAN_POINT('Ctrl Pts',(-2.03832911025913,1.,-0.143035515058208));
#32830=CARTESIAN_POINT('Ctrl Pts',(-2.04414757947919,-1.,-0.140997332152545));
#32831=CARTESIAN_POINT('Ctrl Pts',(-2.04414757947919,1.,-0.140997332152545));
#32832=CARTESIAN_POINT('Ctrl Pts',(-2.04995762001333,-1.,-0.138911255368966));
#32833=CARTESIAN_POINT('Ctrl Pts',(-2.04995762001333,1.,-0.138911255368966));
#32834=CARTESIAN_POINT('Ctrl Pts',(-2.0557604441427,-1.,-0.136777941218044));
#32835=CARTESIAN_POINT('Ctrl Pts',(-2.0557604441427,1.,-0.136777941218044));
#32836=CARTESIAN_POINT('Ctrl Pts',(-2.06155781517844,-1.,-0.134598026192107));
#32837=CARTESIAN_POINT('Ctrl Pts',(-2.06155781517844,1.,-0.134598026192107));
#32838=CARTESIAN_POINT('Ctrl Pts',(-2.06735123910319,-1.,-0.13237211154771));
#32839=CARTESIAN_POINT('Ctrl Pts',(-2.06735123910319,1.,-0.13237211154771));
#32840=CARTESIAN_POINT('Ctrl Pts',(-2.07314114713047,-1.,-0.130100748328401));
#32841=CARTESIAN_POINT('Ctrl Pts',(-2.07314114713047,1.,-0.130100748328401));
#32842=CARTESIAN_POINT('Ctrl Pts',(-2.07892715110967,-1.,-0.127784445276116));
#32843=CARTESIAN_POINT('Ctrl Pts',(-2.07892715110967,1.,-0.127784445276116));
#32844=CARTESIAN_POINT('Ctrl Pts',(-2.08470840653628,-1.,-0.125423679412058));
#32845=CARTESIAN_POINT('Ctrl Pts',(-2.08470840653628,1.,-0.125423679412058));
#32846=CARTESIAN_POINT('Ctrl Pts',(-2.09048392424826,-1.,-0.123018905621083));
#32847=CARTESIAN_POINT('Ctrl Pts',(-2.09048392424826,1.,-0.123018905621083));
#32848=CARTESIAN_POINT('Ctrl Pts',(-2.09625292867756,-1.,-0.120570567965129));
#32849=CARTESIAN_POINT('Ctrl Pts',(-2.09625292867756,1.,-0.120570567965129));
#32850=CARTESIAN_POINT('Ctrl Pts',(-2.10201512132945,-1.,-0.118079107988368));
#32851=CARTESIAN_POINT('Ctrl Pts',(-2.10201512132945,1.,-0.118079107988368));
#32852=CARTESIAN_POINT('Ctrl Pts',(-2.10777050261359,-1.,-0.11554495768794));
#32853=CARTESIAN_POINT('Ctrl Pts',(-2.10777050261359,1.,-0.11554495768794));
#32854=CARTESIAN_POINT('Ctrl Pts',(-2.11351924490335,-1.,-0.112968534419746));
#32855=CARTESIAN_POINT('Ctrl Pts',(-2.11351924490335,1.,-0.112968534419746));
#32856=CARTESIAN_POINT('Ctrl Pts',(-2.11926155590849,-1.,-0.11035023613502));
#32857=CARTESIAN_POINT('Ctrl Pts',(-2.11926155590849,1.,-0.11035023613502));
#32858=CARTESIAN_POINT('Ctrl Pts',(-2.12499752306927,-1.,-0.107690435231068));
#32859=CARTESIAN_POINT('Ctrl Pts',(-2.12499752306927,1.,-0.107690435231068));
#32860=CARTESIAN_POINT('Ctrl Pts',(-2.1307270488718,-1.,-0.104989479152703));
#32861=CARTESIAN_POINT('Ctrl Pts',(-2.1307270488718,1.,-0.104989479152703));
#32862=CARTESIAN_POINT('Ctrl Pts',(-2.13644992667052,-1.,-0.102247700556064));
#32863=CARTESIAN_POINT('Ctrl Pts',(-2.13644992667052,1.,-0.102247700556064));
#32864=CARTESIAN_POINT('Ctrl Pts',(-2.14216588395974,-1.,-0.0994654261990744));
#32865=CARTESIAN_POINT('Ctrl Pts',(-2.14216588395974,1.,-0.0994654261990744));
#32866=CARTESIAN_POINT('Ctrl Pts',(-2.14787463531864,-1.,-0.096642985230569));
#32867=CARTESIAN_POINT('Ctrl Pts',(-2.14787463531864,1.,-0.096642985230569));
#32868=CARTESIAN_POINT('Ctrl Pts',(-2.15357593978377,-1.,-0.0937807218868346));
#32869=CARTESIAN_POINT('Ctrl Pts',(-2.15357593978377,1.,-0.0937807218868346));
#32870=CARTESIAN_POINT('Ctrl Pts',(-2.15926961544808,-1.,-0.0908789888108267));
#32871=CARTESIAN_POINT('Ctrl Pts',(-2.15926961544808,1.,-0.0908789888108267));
#32872=CARTESIAN_POINT('Ctrl Pts',(-2.16495552645275,-1.,-0.0879381291387824));
#32873=CARTESIAN_POINT('Ctrl Pts',(-2.16495552645275,1.,-0.0879381291387824));
#32874=CARTESIAN_POINT('Ctrl Pts',(-2.17063357871031,-1.,-0.0849584620835644));
#32875=CARTESIAN_POINT('Ctrl Pts',(-2.17063357871031,1.,-0.0849584620835644));
#32876=CARTESIAN_POINT('Ctrl Pts',(-2.1763037121106,-1.,-0.0819402680871941));
#32877=CARTESIAN_POINT('Ctrl Pts',(-2.1763037121106,1.,-0.0819402680871941));
#32878=CARTESIAN_POINT('Ctrl Pts',(-2.18196589448304,-1.,-0.0788837727683229));
#32879=CARTESIAN_POINT('Ctrl Pts',(-2.18196589448304,1.,-0.0788837727683229));
#32880=CARTESIAN_POINT('Ctrl Pts',(-2.1876201139874,-1.,-0.0757891465833413));
#32881=CARTESIAN_POINT('Ctrl Pts',(-2.1876201139874,1.,-0.0757891465833413));
#32882=CARTESIAN_POINT('Ctrl Pts',(-2.19213712012956,-1.,-0.0732830357304277));
#32883=CARTESIAN_POINT('Ctrl Pts',(-2.19213712012956,1.,-0.0732830357304277));
#32884=CARTESIAN_POINT('Ctrl Pts',(-2.19552129483562,-1.,-0.0713863779524629));
#32885=CARTESIAN_POINT('Ctrl Pts',(-2.19552129483562,1.,-0.0713863779524629));
#32886=CARTESIAN_POINT('Ctrl Pts',(-2.19777582085261,-1.,-0.0701143536324927));
#32887=CARTESIAN_POINT('Ctrl Pts',(-2.19777582085261,1.,-0.0701143536324927));
#32888=CARTESIAN_POINT('Ctrl Pts',(-2.19890268624765,-1.,-0.0694764450219585));
#32889=CARTESIAN_POINT('Ctrl Pts',(-2.19890268624765,1.,-0.0694764450219585));
#32890=CARTESIAN_POINT('',(-1.74236521665491,1.,-0.163289472382896));
#32891=CARTESIAN_POINT('Ctrl Pts',(-1.74236521665491,1.,-0.163289472382896));
#32892=CARTESIAN_POINT('Ctrl Pts',(-1.74720349503904,1.,-0.163814161002474));
#32893=CARTESIAN_POINT('Ctrl Pts',(-1.75666056640041,1.,-0.164834765708484));
#32894=CARTESIAN_POINT('Ctrl Pts',(-1.77018771687692,1.,-0.166279355148738));
#32895=CARTESIAN_POINT('Ctrl Pts',(-1.78690649988931,1.,-0.16803277280837));
#32896=CARTESIAN_POINT('Ctrl Pts',(-1.80561530633924,1.,-0.169936923908078));
#32897=CARTESIAN_POINT('Ctrl Pts',(-1.82215766815414,1.,-0.171554770207306));
#32898=CARTESIAN_POINT('Ctrl Pts',(-1.83658380530747,1.,-0.17288944289442));
#32899=CARTESIAN_POINT('Ctrl Pts',(-1.84898113200543,1.,-0.173946627589401));
#32900=CARTESIAN_POINT('Ctrl Pts',(-1.85948367089838,1.,-0.174735259276856));
#32901=CARTESIAN_POINT('Ctrl Pts',(-1.86828349694972,1.,-0.175268337590901));
#32902=CARTESIAN_POINT('Ctrl Pts',(-1.87563767773249,1.,-0.175563480746205));
#32903=CARTESIAN_POINT('Ctrl Pts',(-1.88188663144846,1.,-0.175644148889271));
#32904=CARTESIAN_POINT('Ctrl Pts',(-1.88742606272818,1.,-0.175538155840286));
#32905=CARTESIAN_POINT('Ctrl Pts',(-1.89264630198279,1.,-0.175274276190664));
#32906=CARTESIAN_POINT('Ctrl Pts',(-1.89788101117148,1.,-0.174879405091277));
#32907=CARTESIAN_POINT('Ctrl Pts',(-1.90335253863003,1.,-0.174375518661222));
#32908=CARTESIAN_POINT('Ctrl Pts',(-1.90911693975475,1.,-0.173776635257984));
#32909=CARTESIAN_POINT('Ctrl Pts',(-1.91511429159681,1.,-0.173090695383619));
#32910=CARTESIAN_POINT('Ctrl Pts',(-1.92122334398034,1.,-0.172321621259557));
#32911=CARTESIAN_POINT('Ctrl Pts',(-1.92731093582,1.,-0.17147119153296));
#32912=CARTESIAN_POINT('Ctrl Pts',(-1.93329183155455,1.,-0.170541253116136));
#32913=CARTESIAN_POINT('Ctrl Pts',(-1.93915639211497,1.,-0.169534904817425));
#32914=CARTESIAN_POINT('Ctrl Pts',(-1.94493757756879,1.,-0.168455741607516));
#32915=CARTESIAN_POINT('Ctrl Pts',(-1.95069027794286,1.,-0.167307501784469));
#32916=CARTESIAN_POINT('Ctrl Pts',(-1.95646759718755,1.,-0.166093592002833));
#32917=CARTESIAN_POINT('Ctrl Pts',(-1.96229379940174,1.,-0.1648165689203));
#32918=CARTESIAN_POINT('Ctrl Pts',(-1.96816512678,1.,-0.16347818545776));
#32919=CARTESIAN_POINT('Ctrl Pts',(-1.97406280235204,1.,-0.162079693556302));
#32920=CARTESIAN_POINT('Ctrl Pts',(-1.97996195437557,1.,-0.16062206078461));
#32921=CARTESIAN_POINT('Ctrl Pts',(-1.98584238283279,1.,-0.159106226437289));
#32922=CARTESIAN_POINT('Ctrl Pts',(-1.99169810931893,1.,-0.157533331459215));
#32923=CARTESIAN_POINT('Ctrl Pts',(-1.99753284771487,1.,-0.155904629548775));
#32924=CARTESIAN_POINT('Ctrl Pts',(-2.00335565310539,1.,-0.154221403049719));
#32925=CARTESIAN_POINT('Ctrl Pts',(-2.00917680318426,1.,-0.152484883621452));
#32926=CARTESIAN_POINT('Ctrl Pts',(-2.01500291940243,1.,-0.150696157673084));
#32927=CARTESIAN_POINT('Ctrl Pts',(-2.02083464969897,1.,-0.148856124775343));
#32928=CARTESIAN_POINT('Ctrl Pts',(-2.02666926182017,1.,-0.146965557332586));
#32929=CARTESIAN_POINT('Ctrl Pts',(-2.03250223739941,1.,-0.145025140186058));
#32930=CARTESIAN_POINT('Ctrl Pts',(-2.03832911025913,1.,-0.143035515058208));
#32931=CARTESIAN_POINT('Ctrl Pts',(-2.04414757947919,1.,-0.140997332152545));
#32932=CARTESIAN_POINT('Ctrl Pts',(-2.04995762001333,1.,-0.138911255368966));
#32933=CARTESIAN_POINT('Ctrl Pts',(-2.0557604441427,1.,-0.136777941218044));
#32934=CARTESIAN_POINT('Ctrl Pts',(-2.06155781517844,1.,-0.134598026192107));
#32935=CARTESIAN_POINT('Ctrl Pts',(-2.06735123910319,1.,-0.13237211154771));
#32936=CARTESIAN_POINT('Ctrl Pts',(-2.07314114713047,1.,-0.130100748328401));
#32937=CARTESIAN_POINT('Ctrl Pts',(-2.07892715110967,1.,-0.127784445276116));
#32938=CARTESIAN_POINT('Ctrl Pts',(-2.08470840653628,1.,-0.125423679412058));
#32939=CARTESIAN_POINT('Ctrl Pts',(-2.09048392424826,1.,-0.123018905621083));
#32940=CARTESIAN_POINT('Ctrl Pts',(-2.09625292867756,1.,-0.120570567965129));
#32941=CARTESIAN_POINT('Ctrl Pts',(-2.10201512132945,1.,-0.118079107988368));
#32942=CARTESIAN_POINT('Ctrl Pts',(-2.10777050261359,1.,-0.11554495768794));
#32943=CARTESIAN_POINT('Ctrl Pts',(-2.11351924490335,1.,-0.112968534419746));
#32944=CARTESIAN_POINT('Ctrl Pts',(-2.11926155590849,1.,-0.11035023613502));
#32945=CARTESIAN_POINT('Ctrl Pts',(-2.12499752306927,1.,-0.107690435231068));
#32946=CARTESIAN_POINT('Ctrl Pts',(-2.1307270488718,1.,-0.104989479152703));
#32947=CARTESIAN_POINT('Ctrl Pts',(-2.13644992667052,1.,-0.102247700556064));
#32948=CARTESIAN_POINT('Ctrl Pts',(-2.14216588395974,1.,-0.0994654261990744));
#32949=CARTESIAN_POINT('Ctrl Pts',(-2.14787463531864,1.,-0.096642985230569));
#32950=CARTESIAN_POINT('Ctrl Pts',(-2.15357593978377,1.,-0.0937807218868346));
#32951=CARTESIAN_POINT('Ctrl Pts',(-2.15926961544808,1.,-0.0908789888108267));
#32952=CARTESIAN_POINT('Ctrl Pts',(-2.16495552645275,1.,-0.0879381291387824));
#32953=CARTESIAN_POINT('Ctrl Pts',(-2.17063357871031,1.,-0.0849584620835644));
#32954=CARTESIAN_POINT('Ctrl Pts',(-2.1763037121106,1.,-0.0819402680871941));
#32955=CARTESIAN_POINT('Ctrl Pts',(-2.18196589448304,1.,-0.0788837727683229));
#32956=CARTESIAN_POINT('Ctrl Pts',(-2.1876201139874,1.,-0.0757891465833413));
#32957=CARTESIAN_POINT('Ctrl Pts',(-2.19213712012956,1.,-0.0732830357304277));
#32958=CARTESIAN_POINT('Ctrl Pts',(-2.19552129483562,1.,-0.0713863779524629));
#32959=CARTESIAN_POINT('Ctrl Pts',(-2.19777582085261,1.,-0.0701143536324927));
#32960=CARTESIAN_POINT('Ctrl Pts',(-2.19890268624765,1.,-0.0694764450219585));
#32961=CARTESIAN_POINT('',(-1.74236521665491,0.,-0.163289472382896));
#32962=CARTESIAN_POINT('Origin',(0.,0.,0.));
#32963=CARTESIAN_POINT('',(-1.7075470150345,1.,-0.383122945602004));
#32964=CARTESIAN_POINT('Origin',(0.,1.,0.));
#32965=CARTESIAN_POINT('',(-1.7075470150345,0.,-0.383122945602004));
#32966=CARTESIAN_POINT('Ctrl Pts',(-2.11275013067528,-1.,-0.61342227326009));
#32967=CARTESIAN_POINT('Ctrl Pts',(-2.11275013067528,1.,-0.61342227326009));
#32968=CARTESIAN_POINT('Ctrl Pts',(-2.11187554260142,-1.,-0.61246736556225));
#32969=CARTESIAN_POINT('Ctrl Pts',(-2.11187554260142,1.,-0.61246736556225));
#32970=CARTESIAN_POINT('Ctrl Pts',(-2.11012443807661,-1.,-0.610560911691113));
#32971=CARTESIAN_POINT('Ctrl Pts',(-2.11012443807661,1.,-0.610560911691113));
#32972=CARTESIAN_POINT('Ctrl Pts',(-2.10749199615859,-1.,-0.607711315456826));
#32973=CARTESIAN_POINT('Ctrl Pts',(-2.10749199615859,1.,-0.607711315456826));
#32974=CARTESIAN_POINT('Ctrl Pts',(-2.10397049887709,-1.,-0.603932030738212));
#32975=CARTESIAN_POINT('Ctrl Pts',(-2.10397049887709,1.,-0.603932030738212));
#32976=CARTESIAN_POINT('Ctrl Pts',(-2.09954930865331,-1.,-0.599241616422144));
#32977=CARTESIAN_POINT('Ctrl Pts',(-2.09954930865331,1.,-0.599241616422144));
#32978=CARTESIAN_POINT('Ctrl Pts',(-2.09510876220501,-1.,-0.594585006052823));
#32979=CARTESIAN_POINT('Ctrl Pts',(-2.09510876220501,1.,-0.594585006052823));
#32980=CARTESIAN_POINT('Ctrl Pts',(-2.09064881812053,-1.,-0.589962365403189));
#32981=CARTESIAN_POINT('Ctrl Pts',(-2.09064881812053,1.,-0.589962365403189));
#32982=CARTESIAN_POINT('Ctrl Pts',(-2.086169437277,-1.,-0.585373918990895));
#32983=CARTESIAN_POINT('Ctrl Pts',(-2.086169437277,1.,-0.585373918990895));
#32984=CARTESIAN_POINT('Ctrl Pts',(-2.08167059018138,-1.,-0.580819952107257));
#32985=CARTESIAN_POINT('Ctrl Pts',(-2.08167059018138,1.,-0.580819952107257));
#32986=CARTESIAN_POINT('Ctrl Pts',(-2.07715226767361,-1.,-0.576300797416274));
#32987=CARTESIAN_POINT('Ctrl Pts',(-2.07715226767361,1.,-0.576300797416274));
#32988=CARTESIAN_POINT('Ctrl Pts',(-2.07261449292757,-1.,-0.571816823242411));
#32989=CARTESIAN_POINT('Ctrl Pts',(-2.07261449292757,1.,-0.571816823242411));
#32990=CARTESIAN_POINT('Ctrl Pts',(-2.06805732997383,-1.,-0.567368421181229));
#32991=CARTESIAN_POINT('Ctrl Pts',(-2.06805732997383,1.,-0.567368421181229));
#32992=CARTESIAN_POINT('Ctrl Pts',(-2.06348090160697,-1.,-0.562955993082574));
#32993=CARTESIAN_POINT('Ctrl Pts',(-2.06348090160697,1.,-0.562955993082574));
#32994=CARTESIAN_POINT('Ctrl Pts',(-2.05888537756571,-1.,-0.558579940185467));
#32995=CARTESIAN_POINT('Ctrl Pts',(-2.05888537756571,1.,-0.558579940185467));
#32996=CARTESIAN_POINT('Ctrl Pts',(-2.05427091604482,-1.,-0.554240657464109));
#32997=CARTESIAN_POINT('Ctrl Pts',(-2.05427091604482,1.,-0.554240657464109));
#32998=CARTESIAN_POINT('Ctrl Pts',(-2.04963761077974,-1.,-0.549938525150342));
#32999=CARTESIAN_POINT('Ctrl Pts',(-2.04963761077974,1.,-0.549938525150342));
#33000=CARTESIAN_POINT('Ctrl Pts',(-2.0449854471456,-1.,-0.545673903817348));
#33001=CARTESIAN_POINT('Ctrl Pts',(-2.0449854471456,1.,-0.545673903817348));
#33002=CARTESIAN_POINT('Ctrl Pts',(-2.0403142269048,-1.,-0.54144712061552));
#33003=CARTESIAN_POINT('Ctrl Pts',(-2.0403142269048,1.,-0.54144712061552));
#33004=CARTESIAN_POINT('Ctrl Pts',(-2.03562362953993,-1.,-0.537258489833134));
#33005=CARTESIAN_POINT('Ctrl Pts',(-2.03562362953993,1.,-0.537258489833134));
#33006=CARTESIAN_POINT('Ctrl Pts',(-2.03091336214401,-1.,-0.533108355132905));
#33007=CARTESIAN_POINT('Ctrl Pts',(-2.03091336214401,1.,-0.533108355132905));
#33008=CARTESIAN_POINT('Ctrl Pts',(-2.02618329083289,-1.,-0.52899712724191));
#33009=CARTESIAN_POINT('Ctrl Pts',(-2.02618329083289,1.,-0.52899712724191));
#33010=CARTESIAN_POINT('Ctrl Pts',(-2.02143356304712,-1.,-0.524925318333518));
#33011=CARTESIAN_POINT('Ctrl Pts',(-2.02143356304712,1.,-0.524925318333518));
#33012=CARTESIAN_POINT('Ctrl Pts',(-2.01666477917305,-1.,-0.520893590399428));
#33013=CARTESIAN_POINT('Ctrl Pts',(-2.01666477917305,1.,-0.520893590399428));
#33014=CARTESIAN_POINT('Ctrl Pts',(-2.01187773939257,-1.,-0.516902681728733));
#33015=CARTESIAN_POINT('Ctrl Pts',(-2.01187773939257,1.,-0.516902681728733));
#33016=CARTESIAN_POINT('Ctrl Pts',(-2.00707309946955,-1.,-0.512953306961813));
#33017=CARTESIAN_POINT('Ctrl Pts',(-2.00707309946955,1.,-0.512953306961813));
#33018=CARTESIAN_POINT('Ctrl Pts',(-2.00225107134733,-1.,-0.509046069886152));
#33019=CARTESIAN_POINT('Ctrl Pts',(-2.00225107134733,1.,-0.509046069886152));
#33020=CARTESIAN_POINT('Ctrl Pts',(-1.99741107463567,-1.,-0.505181361323011));
#33021=CARTESIAN_POINT('Ctrl Pts',(-1.99741107463567,1.,-0.505181361323011));
#33022=CARTESIAN_POINT('Ctrl Pts',(-1.9925514912615,-1.,-0.501359287727129));
#33023=CARTESIAN_POINT('Ctrl Pts',(-1.9925514912615,1.,-0.501359287727129));
#33024=CARTESIAN_POINT('Ctrl Pts',(-1.98767044752929,-1.,-0.497579909545564));
#33025=CARTESIAN_POINT('Ctrl Pts',(-1.98767044752929,1.,-0.497579909545564));
#33026=CARTESIAN_POINT('Ctrl Pts',(-1.9827665876182,-1.,-0.493843476541492));
#33027=CARTESIAN_POINT('Ctrl Pts',(-1.9827665876182,1.,-0.493843476541492));
#33028=CARTESIAN_POINT('Ctrl Pts',(-1.97783973019229,-1.,-0.490150627860955));
#33029=CARTESIAN_POINT('Ctrl Pts',(-1.97783973019229,1.,-0.490150627860955));
#33030=CARTESIAN_POINT('Ctrl Pts',(-1.97289186263272,-1.,-0.486502692907661));
#33031=CARTESIAN_POINT('Ctrl Pts',(-1.97289186263272,1.,-0.486502692907661));
#33032=CARTESIAN_POINT('Ctrl Pts',(-1.96792703422358,-1.,-0.482901662120686));
#33033=CARTESIAN_POINT('Ctrl Pts',(-1.96792703422358,1.,-0.482901662120686));
#33034=CARTESIAN_POINT('Ctrl Pts',(-1.96294933055938,-1.,-0.479349583074846));
#33035=CARTESIAN_POINT('Ctrl Pts',(-1.96294933055938,1.,-0.479349583074846));
#33036=CARTESIAN_POINT('Ctrl Pts',(-1.95796111148175,-1.,-0.475848034683171));
#33037=CARTESIAN_POINT('Ctrl Pts',(-1.95796111148175,1.,-0.475848034683171));
#33038=CARTESIAN_POINT('Ctrl Pts',(-1.95296148278136,-1.,-0.472397672264079));
#33039=CARTESIAN_POINT('Ctrl Pts',(-1.95296148278136,1.,-0.472397672264079));
#33040=CARTESIAN_POINT('Ctrl Pts',(-1.94794381136524,-1.,-0.468997482913158));
#33041=CARTESIAN_POINT('Ctrl Pts',(-1.94794381136524,1.,-0.468997482913158));
#33042=CARTESIAN_POINT('Ctrl Pts',(-1.94289794196205,-1.,-0.465645462026064));
#33043=CARTESIAN_POINT('Ctrl Pts',(-1.94289794196205,1.,-0.465645462026064));
#33044=CARTESIAN_POINT('Ctrl Pts',(-1.93781486640834,-1.,-0.462340031009087));
#33045=CARTESIAN_POINT('Ctrl Pts',(-1.93781486640834,1.,-0.462340031009087));
#33046=CARTESIAN_POINT('Ctrl Pts',(-1.93269066517936,-1.,-0.459081234547931));
#33047=CARTESIAN_POINT('Ctrl Pts',(-1.93269066517936,1.,-0.459081234547931));
#33048=CARTESIAN_POINT('Ctrl Pts',(-1.92753067150461,-1.,-0.455872005174335));
#33049=CARTESIAN_POINT('Ctrl Pts',(-1.92753067150461,1.,-0.455872005174335));
#33050=CARTESIAN_POINT('Ctrl Pts',(-1.9223538064847,-1.,-0.452719478359356));
#33051=CARTESIAN_POINT('Ctrl Pts',(-1.9223538064847,1.,-0.452719478359356));
#33052=CARTESIAN_POINT('Ctrl Pts',(-1.91718342555717,-1.,-0.449632260106572));
#33053=CARTESIAN_POINT('Ctrl Pts',(-1.91718342555717,1.,-0.449632260106572));
#33054=CARTESIAN_POINT('Ctrl Pts',(-1.91203699981095,-1.,-0.446617343485651));
#33055=CARTESIAN_POINT('Ctrl Pts',(-1.91203699981095,1.,-0.446617343485651));
#33056=CARTESIAN_POINT('Ctrl Pts',(-1.90691756144906,-1.,-0.44367755684917));
#33057=CARTESIAN_POINT('Ctrl Pts',(-1.90691756144906,1.,-0.44367755684917));
#33058=CARTESIAN_POINT('Ctrl Pts',(-1.90180124389137,-1.,-0.44080783370416));
#33059=CARTESIAN_POINT('Ctrl Pts',(-1.90180124389137,1.,-0.44080783370416));
#33060=CARTESIAN_POINT('Ctrl Pts',(-1.89663648956549,-1.,-0.437995003948443));
#33061=CARTESIAN_POINT('Ctrl Pts',(-1.89663648956549,1.,-0.437995003948443));
#33062=CARTESIAN_POINT('Ctrl Pts',(-1.89136993975585,-1.,-0.43522566096358));
#33063=CARTESIAN_POINT('Ctrl Pts',(-1.89136993975585,1.,-0.43522566096358));
#33064=CARTESIAN_POINT('Ctrl Pts',(-1.88596913666828,-1.,-0.432493038548833));
#33065=CARTESIAN_POINT('Ctrl Pts',(-1.88596913666828,1.,-0.432493038548833));
#33066=CARTESIAN_POINT('Ctrl Pts',(-1.88044229001778,-1.,-0.429803062482217));
#33067=CARTESIAN_POINT('Ctrl Pts',(-1.88044229001778,1.,-0.429803062482217));
#33068=CARTESIAN_POINT('Ctrl Pts',(-1.87486989291333,-1.,-0.427183828518743));
#33069=CARTESIAN_POINT('Ctrl Pts',(-1.87486989291333,1.,-0.427183828518743));
#33070=CARTESIAN_POINT('Ctrl Pts',(-1.8693780394412,-1.,-0.424678177290876));
#33071=CARTESIAN_POINT('Ctrl Pts',(-1.8693780394412,1.,-0.424678177290876));
#33072=CARTESIAN_POINT('Ctrl Pts',(-1.86408083333863,-1.,-0.422327307417884));
#33073=CARTESIAN_POINT('Ctrl Pts',(-1.86408083333863,1.,-0.422327307417884));
#33074=CARTESIAN_POINT('Ctrl Pts',(-1.8590328109667,-1.,-0.420157287975583));
#33075=CARTESIAN_POINT('Ctrl Pts',(-1.8590328109667,1.,-0.420157287975583));
#33076=CARTESIAN_POINT('Ctrl Pts',(-1.8541763285645,-1.,-0.418164129144045));
#33077=CARTESIAN_POINT('Ctrl Pts',(-1.8541763285645,1.,-0.418164129144045));
#33078=CARTESIAN_POINT('Ctrl Pts',(-1.84929312930314,-1.,-0.416300022039885));
#33079=CARTESIAN_POINT('Ctrl Pts',(-1.84929312930314,1.,-0.416300022039885));
#33080=CARTESIAN_POINT('Ctrl Pts',(-1.84405757074218,-1.,-0.414487438255542));
#33081=CARTESIAN_POINT('Ctrl Pts',(-1.84405757074218,1.,-0.414487438255542));
#33082=CARTESIAN_POINT('Ctrl Pts',(-1.8380895347617,-1.,-0.412633125322945));
#33083=CARTESIAN_POINT('Ctrl Pts',(-1.8380895347617,1.,-0.412633125322945));
#33084=CARTESIAN_POINT('Ctrl Pts',(-1.83100408895047,-1.,-0.410641256301276));
#33085=CARTESIAN_POINT('Ctrl Pts',(-1.83100408895047,1.,-0.410641256301276));
#33086=CARTESIAN_POINT('Ctrl Pts',(-1.82247022677562,-1.,-0.408428948106227));
#33087=CARTESIAN_POINT('Ctrl Pts',(-1.82247022677562,1.,-0.408428948106227));
#33088=CARTESIAN_POINT('Ctrl Pts',(-1.81223801812013,-1.,-0.405933518407175));
#33089=CARTESIAN_POINT('Ctrl Pts',(-1.81223801812013,1.,-0.405933518407175));
#33090=CARTESIAN_POINT('Ctrl Pts',(-1.80012077173238,-1.,-0.403107976163396));
#33091=CARTESIAN_POINT('Ctrl Pts',(-1.80012077173238,1.,-0.403107976163396));
#33092=CARTESIAN_POINT('Ctrl Pts',(-1.78598826343754,-1.,-0.399919403774155));
#33093=CARTESIAN_POINT('Ctrl Pts',(-1.78598826343754,1.,-0.399919403774155));
#33094=CARTESIAN_POINT('Ctrl Pts',(-1.76975560043442,-1.,-0.396346196110688));
#33095=CARTESIAN_POINT('Ctrl Pts',(-1.76975560043442,1.,-0.396346196110688));
#33096=CARTESIAN_POINT('Ctrl Pts',(-1.75137405310193,-1.,-0.392375812285395));
#33097=CARTESIAN_POINT('Ctrl Pts',(-1.75137405310193,1.,-0.392375812285395));
#33098=CARTESIAN_POINT('Ctrl Pts',(-1.73493170972829,-1.,-0.388877023502615));
#33099=CARTESIAN_POINT('Ctrl Pts',(-1.73493170972829,1.,-0.388877023502615));
#33100=CARTESIAN_POINT('Ctrl Pts',(-1.72162022244582,-1.,-0.386070790323281));
#33101=CARTESIAN_POINT('Ctrl Pts',(-1.72162022244582,1.,-0.386070790323281));
#33102=CARTESIAN_POINT('Ctrl Pts',(-1.71231062891398,-1.,-0.384119047314215));
#33103=CARTESIAN_POINT('Ctrl Pts',(-1.71231062891398,1.,-0.384119047314215));
#33104=CARTESIAN_POINT('Ctrl Pts',(-1.7075470150345,-1.,-0.383122945602004));
#33105=CARTESIAN_POINT('Ctrl Pts',(-1.7075470150345,1.,-0.383122945602004));
#33106=CARTESIAN_POINT('',(-2.11275013067528,1.,-0.61342227326009));
#33107=CARTESIAN_POINT('Ctrl Pts',(-2.11275013067528,1.,-0.61342227326009));
#33108=CARTESIAN_POINT('Ctrl Pts',(-2.11187554260142,1.,-0.61246736556225));
#33109=CARTESIAN_POINT('Ctrl Pts',(-2.11012443807661,1.,-0.610560911691113));
#33110=CARTESIAN_POINT('Ctrl Pts',(-2.10749199615859,1.,-0.607711315456826));
#33111=CARTESIAN_POINT('Ctrl Pts',(-2.10397049887709,1.,-0.603932030738212));
#33112=CARTESIAN_POINT('Ctrl Pts',(-2.09954930865331,1.,-0.599241616422144));
#33113=CARTESIAN_POINT('Ctrl Pts',(-2.09510876220501,1.,-0.594585006052823));
#33114=CARTESIAN_POINT('Ctrl Pts',(-2.09064881812053,1.,-0.589962365403189));
#33115=CARTESIAN_POINT('Ctrl Pts',(-2.086169437277,1.,-0.585373918990895));
#33116=CARTESIAN_POINT('Ctrl Pts',(-2.08167059018138,1.,-0.580819952107257));
#33117=CARTESIAN_POINT('Ctrl Pts',(-2.07715226767361,1.,-0.576300797416274));
#33118=CARTESIAN_POINT('Ctrl Pts',(-2.07261449292757,1.,-0.571816823242411));
#33119=CARTESIAN_POINT('Ctrl Pts',(-2.06805732997383,1.,-0.567368421181229));
#33120=CARTESIAN_POINT('Ctrl Pts',(-2.06348090160697,1.,-0.562955993082574));
#33121=CARTESIAN_POINT('Ctrl Pts',(-2.05888537756571,1.,-0.558579940185467));
#33122=CARTESIAN_POINT('Ctrl Pts',(-2.05427091604482,1.,-0.554240657464109));
#33123=CARTESIAN_POINT('Ctrl Pts',(-2.04963761077974,1.,-0.549938525150342));
#33124=CARTESIAN_POINT('Ctrl Pts',(-2.0449854471456,1.,-0.545673903817348));
#33125=CARTESIAN_POINT('Ctrl Pts',(-2.0403142269048,1.,-0.54144712061552));
#33126=CARTESIAN_POINT('Ctrl Pts',(-2.03562362953993,1.,-0.537258489833134));
#33127=CARTESIAN_POINT('Ctrl Pts',(-2.03091336214401,1.,-0.533108355132905));
#33128=CARTESIAN_POINT('Ctrl Pts',(-2.02618329083289,1.,-0.52899712724191));
#33129=CARTESIAN_POINT('Ctrl Pts',(-2.02143356304712,1.,-0.524925318333518));
#33130=CARTESIAN_POINT('Ctrl Pts',(-2.01666477917305,1.,-0.520893590399428));
#33131=CARTESIAN_POINT('Ctrl Pts',(-2.01187773939257,1.,-0.516902681728733));
#33132=CARTESIAN_POINT('Ctrl Pts',(-2.00707309946955,1.,-0.512953306961813));
#33133=CARTESIAN_POINT('Ctrl Pts',(-2.00225107134733,1.,-0.509046069886152));
#33134=CARTESIAN_POINT('Ctrl Pts',(-1.99741107463567,1.,-0.505181361323011));
#33135=CARTESIAN_POINT('Ctrl Pts',(-1.9925514912615,1.,-0.501359287727129));
#33136=CARTESIAN_POINT('Ctrl Pts',(-1.98767044752929,1.,-0.497579909545564));
#33137=CARTESIAN_POINT('Ctrl Pts',(-1.9827665876182,1.,-0.493843476541492));
#33138=CARTESIAN_POINT('Ctrl Pts',(-1.97783973019229,1.,-0.490150627860955));
#33139=CARTESIAN_POINT('Ctrl Pts',(-1.97289186263272,1.,-0.486502692907661));
#33140=CARTESIAN_POINT('Ctrl Pts',(-1.96792703422358,1.,-0.482901662120686));
#33141=CARTESIAN_POINT('Ctrl Pts',(-1.96294933055938,1.,-0.479349583074846));
#33142=CARTESIAN_POINT('Ctrl Pts',(-1.95796111148175,1.,-0.475848034683171));
#33143=CARTESIAN_POINT('Ctrl Pts',(-1.95296148278136,1.,-0.472397672264079));
#33144=CARTESIAN_POINT('Ctrl Pts',(-1.94794381136524,1.,-0.468997482913158));
#33145=CARTESIAN_POINT('Ctrl Pts',(-1.94289794196205,1.,-0.465645462026064));
#33146=CARTESIAN_POINT('Ctrl Pts',(-1.93781486640834,1.,-0.462340031009087));
#33147=CARTESIAN_POINT('Ctrl Pts',(-1.93269066517936,1.,-0.459081234547931));
#33148=CARTESIAN_POINT('Ctrl Pts',(-1.92753067150461,1.,-0.455872005174335));
#33149=CARTESIAN_POINT('Ctrl Pts',(-1.9223538064847,1.,-0.452719478359356));
#33150=CARTESIAN_POINT('Ctrl Pts',(-1.91718342555717,1.,-0.449632260106572));
#33151=CARTESIAN_POINT('Ctrl Pts',(-1.91203699981095,1.,-0.446617343485651));
#33152=CARTESIAN_POINT('Ctrl Pts',(-1.90691756144906,1.,-0.44367755684917));
#33153=CARTESIAN_POINT('Ctrl Pts',(-1.90180124389137,1.,-0.44080783370416));
#33154=CARTESIAN_POINT('Ctrl Pts',(-1.89663648956549,1.,-0.437995003948443));
#33155=CARTESIAN_POINT('Ctrl Pts',(-1.89136993975585,1.,-0.43522566096358));
#33156=CARTESIAN_POINT('Ctrl Pts',(-1.88596913666828,1.,-0.432493038548833));
#33157=CARTESIAN_POINT('Ctrl Pts',(-1.88044229001778,1.,-0.429803062482217));
#33158=CARTESIAN_POINT('Ctrl Pts',(-1.87486989291333,1.,-0.427183828518743));
#33159=CARTESIAN_POINT('Ctrl Pts',(-1.8693780394412,1.,-0.424678177290876));
#33160=CARTESIAN_POINT('Ctrl Pts',(-1.86408083333863,1.,-0.422327307417884));
#33161=CARTESIAN_POINT('Ctrl Pts',(-1.8590328109667,1.,-0.420157287975583));
#33162=CARTESIAN_POINT('Ctrl Pts',(-1.8541763285645,1.,-0.418164129144045));
#33163=CARTESIAN_POINT('Ctrl Pts',(-1.84929312930314,1.,-0.416300022039885));
#33164=CARTESIAN_POINT('Ctrl Pts',(-1.84405757074218,1.,-0.414487438255542));
#33165=CARTESIAN_POINT('Ctrl Pts',(-1.8380895347617,1.,-0.412633125322945));
#33166=CARTESIAN_POINT('Ctrl Pts',(-1.83100408895047,1.,-0.410641256301276));
#33167=CARTESIAN_POINT('Ctrl Pts',(-1.82247022677562,1.,-0.408428948106227));
#33168=CARTESIAN_POINT('Ctrl Pts',(-1.81223801812013,1.,-0.405933518407175));
#33169=CARTESIAN_POINT('Ctrl Pts',(-1.80012077173238,1.,-0.403107976163396));
#33170=CARTESIAN_POINT('Ctrl Pts',(-1.78598826343754,1.,-0.399919403774155));
#33171=CARTESIAN_POINT('Ctrl Pts',(-1.76975560043442,1.,-0.396346196110688));
#33172=CARTESIAN_POINT('Ctrl Pts',(-1.75137405310193,1.,-0.392375812285395));
#33173=CARTESIAN_POINT('Ctrl Pts',(-1.73493170972829,1.,-0.388877023502615));
#33174=CARTESIAN_POINT('Ctrl Pts',(-1.72162022244582,1.,-0.386070790323281));
#33175=CARTESIAN_POINT('Ctrl Pts',(-1.71231062891398,1.,-0.384119047314215));
#33176=CARTESIAN_POINT('Ctrl Pts',(-1.7075470150345,1.,-0.383122945602004));
#33177=CARTESIAN_POINT('',(-2.11275013067528,0.,-0.61342227326009));
#33178=CARTESIAN_POINT('Origin',(-2.0698113262342,0.,-0.745574324794401));
#33179=CARTESIAN_POINT('',(-2.0698113262342,1.,-0.745574324794401));
#33180=CARTESIAN_POINT('',(-2.11275013067528,1.,-0.61342227326009));
#33181=CARTESIAN_POINT('',(-2.0698113262342,0.,-0.745574324794401));
#33182=CARTESIAN_POINT('Ctrl Pts',(-1.60662857109684,-1.,-0.693717979106306));
#33183=CARTESIAN_POINT('Ctrl Pts',(-1.60662857109684,1.,-0.693717979106306));
#33184=CARTESIAN_POINT('Ctrl Pts',(-1.61106790958151,-1.,-0.695712097881194));
#33185=CARTESIAN_POINT('Ctrl Pts',(-1.61106790958151,1.,-0.695712097881194));
#33186=CARTESIAN_POINT('Ctrl Pts',(-1.61974673472612,-1.,-0.699605146405088));
#33187=CARTESIAN_POINT('Ctrl Pts',(-1.61974673472612,1.,-0.699605146405088));
#33188=CARTESIAN_POINT('Ctrl Pts',(-1.63216541664676,-1.,-0.705159151988319));
#33189=CARTESIAN_POINT('Ctrl Pts',(-1.63216541664676,1.,-0.705159151988319));
#33190=CARTESIAN_POINT('Ctrl Pts',(-1.64752408832016,-1.,-0.711993139355394));
#33191=CARTESIAN_POINT('Ctrl Pts',(-1.64752408832016,1.,-0.711993139355394));
#33192=CARTESIAN_POINT('Ctrl Pts',(-1.6647288055568,-1.,-0.719585433804282));
#33193=CARTESIAN_POINT('Ctrl Pts',(-1.6647288055568,1.,-0.719585433804282));
#33194=CARTESIAN_POINT('Ctrl Pts',(-1.67996158455503,-1.,-0.726235967997433));
#33195=CARTESIAN_POINT('Ctrl Pts',(-1.67996158455503,1.,-0.726235967997433));
#33196=CARTESIAN_POINT('Ctrl Pts',(-1.69326921975743,-1.,-0.731963238697195));
#33197=CARTESIAN_POINT('Ctrl Pts',(-1.69326921975743,1.,-0.731963238697195));
#33198=CARTESIAN_POINT('Ctrl Pts',(-1.70473309006121,-1.,-0.736799665724771));
#33199=CARTESIAN_POINT('Ctrl Pts',(-1.70473309006121,1.,-0.736799665724771));
#33200=CARTESIAN_POINT('Ctrl Pts',(-1.71447789751927,-1.,-0.740795162032087));
#33201=CARTESIAN_POINT('Ctrl Pts',(-1.71447789751927,1.,-0.740795162032087));
#33202=CARTESIAN_POINT('Ctrl Pts',(-1.7226822991693,-1.,-0.744021445433764));
#33203=CARTESIAN_POINT('Ctrl Pts',(-1.7226822991693,1.,-0.744021445433764));
#33204=CARTESIAN_POINT('Ctrl Pts',(-1.72958533647399,-1.,-0.746574710096436));
#33205=CARTESIAN_POINT('Ctrl Pts',(-1.72958533647399,1.,-0.746574710096436));
#33206=CARTESIAN_POINT('Ctrl Pts',(-1.73550351679848,-1.,-0.748582462954854));
#33207=CARTESIAN_POINT('Ctrl Pts',(-1.73550351679848,1.,-0.748582462954854));
#33208=CARTESIAN_POINT('Ctrl Pts',(-1.74080458266705,-1.,-0.75019343597954));
#33209=CARTESIAN_POINT('Ctrl Pts',(-1.74080458266705,1.,-0.75019343597954));
#33210=CARTESIAN_POINT('Ctrl Pts',(-1.74585086852298,-1.,-0.751555614163629));
#33211=CARTESIAN_POINT('Ctrl Pts',(-1.74585086852298,1.,-0.751555614163629));
#33212=CARTESIAN_POINT('Ctrl Pts',(-1.75095139468809,-1.,-0.752797683531377));
#33213=CARTESIAN_POINT('Ctrl Pts',(-1.75095139468809,1.,-0.752797683531377));
#33214=CARTESIAN_POINT('Ctrl Pts',(-1.75631083600175,-1.,-0.75400925402848));
#33215=CARTESIAN_POINT('Ctrl Pts',(-1.75631083600175,1.,-0.75400925402848));
#33216=CARTESIAN_POINT('Ctrl Pts',(-1.7619781724032,-1.,-0.755220979975262));
#33217=CARTESIAN_POINT('Ctrl Pts',(-1.7619781724032,1.,-0.755220979975262));
#33218=CARTESIAN_POINT('Ctrl Pts',(-1.76789396003141,-1.,-0.756421896028403));
#33219=CARTESIAN_POINT('Ctrl Pts',(-1.76789396003141,1.,-0.756421896028403));
#33220=CARTESIAN_POINT('Ctrl Pts',(-1.77394167108342,-1.,-0.757578264077238));
#33221=CARTESIAN_POINT('Ctrl Pts',(-1.77394167108342,1.,-0.757578264077238));
#33222=CARTESIAN_POINT('Ctrl Pts',(-1.77999411220912,-1.,-0.75865062667738));
#33223=CARTESIAN_POINT('Ctrl Pts',(-1.77999411220912,1.,-0.75865062667738));
#33224=CARTESIAN_POINT('Ctrl Pts',(-1.78596964884526,-1.,-0.759614401109868));
#33225=CARTESIAN_POINT('Ctrl Pts',(-1.78596964884526,1.,-0.759614401109868));
#33226=CARTESIAN_POINT('Ctrl Pts',(-1.79185815610802,-1.,-0.760469555880425));
#33227=CARTESIAN_POINT('Ctrl Pts',(-1.79185815610802,1.,-0.760469555880425));
#33228=CARTESIAN_POINT('Ctrl Pts',(-1.79768986997735,-1.,-0.761229695230359));
#33229=CARTESIAN_POINT('Ctrl Pts',(-1.79768986997735,1.,-0.761229695230359));
#33230=CARTESIAN_POINT('Ctrl Pts',(-1.80351583877334,-1.,-0.761915336443515));
#33231=CARTESIAN_POINT('Ctrl Pts',(-1.80351583877334,1.,-0.761915336443515));
#33232=CARTESIAN_POINT('Ctrl Pts',(-1.80938551463989,-1.,-0.762546129464036));
#33233=CARTESIAN_POINT('Ctrl Pts',(-1.80938551463989,1.,-0.762546129464036));
#33234=CARTESIAN_POINT('Ctrl Pts',(-1.81532118405566,-1.,-0.763132003836783));
#33235=CARTESIAN_POINT('Ctrl Pts',(-1.81532118405566,1.,-0.763132003836783));
#33236=CARTESIAN_POINT('Ctrl Pts',(-1.82131873145297,-1.,-0.763673465462854));
#33237=CARTESIAN_POINT('Ctrl Pts',(-1.82131873145297,1.,-0.763673465462854));
#33238=CARTESIAN_POINT('Ctrl Pts',(-1.8273599120008,-1.,-0.764165902606055));
#33239=CARTESIAN_POINT('Ctrl Pts',(-1.8273599120008,1.,-0.764165902606055));
#33240=CARTESIAN_POINT('Ctrl Pts',(-1.8334207722714,-1.,-0.764602549687845));
#33241=CARTESIAN_POINT('Ctrl Pts',(-1.8334207722714,1.,-0.764602549687845));
#33242=CARTESIAN_POINT('Ctrl Pts',(-1.83948181064823,-1.,-0.764978057881687));
#33243=CARTESIAN_POINT('Ctrl Pts',(-1.83948181064823,1.,-0.764978057881687));
#33244=CARTESIAN_POINT('Ctrl Pts',(-1.8455369887591,-1.,-0.765291664861971));
#33245=CARTESIAN_POINT('Ctrl Pts',(-1.8455369887591,1.,-0.765291664861971));
#33246=CARTESIAN_POINT('Ctrl Pts',(-1.85158945130054,-1.,-0.765545710619023));
#33247=CARTESIAN_POINT('Ctrl Pts',(-1.85158945130054,1.,-0.765545710619023));
#33248=CARTESIAN_POINT('Ctrl Pts',(-1.85764741390391,-1.,-0.765744212909305));
#33249=CARTESIAN_POINT('Ctrl Pts',(-1.85764741390391,1.,-0.765744212909305));
#33250=CARTESIAN_POINT('Ctrl Pts',(-1.86372027063314,-1.,-0.765891519092557));
#33251=CARTESIAN_POINT('Ctrl Pts',(-1.86372027063314,1.,-0.765891519092557));
#33252=CARTESIAN_POINT('Ctrl Pts',(-1.86981398314345,-1.,-0.765990708546111));
#33253=CARTESIAN_POINT('Ctrl Pts',(-1.86981398314345,1.,-0.765990708546111));
#33254=CARTESIAN_POINT('Ctrl Pts',(-1.87592888967886,-1.,-0.766042837036759));
#33255=CARTESIAN_POINT('Ctrl Pts',(-1.87592888967886,1.,-0.766042837036759));
#33256=CARTESIAN_POINT('Ctrl Pts',(-1.88206215302561,-1.,-0.766047794851868));
#33257=CARTESIAN_POINT('Ctrl Pts',(-1.88206215302561,1.,-0.766047794851868));
#33258=CARTESIAN_POINT('Ctrl Pts',(-1.88820926433409,-1.,-0.76600483706209));
#33259=CARTESIAN_POINT('Ctrl Pts',(-1.88820926433409,1.,-0.76600483706209));
#33260=CARTESIAN_POINT('Ctrl Pts',(-1.89436577771389,-1.,-0.765913193856979));
#33261=CARTESIAN_POINT('Ctrl Pts',(-1.89436577771389,1.,-0.765913193856979));
#33262=CARTESIAN_POINT('Ctrl Pts',(-1.90052930393599,-1.,-0.765772772593395));
#33263=CARTESIAN_POINT('Ctrl Pts',(-1.90052930393599,1.,-0.765772772593395));
#33264=CARTESIAN_POINT('Ctrl Pts',(-1.90669961402362,-1.,-0.765584196937936));
#33265=CARTESIAN_POINT('Ctrl Pts',(-1.90669961402362,1.,-0.765584196937936));
#33266=CARTESIAN_POINT('Ctrl Pts',(-1.91287765805174,-1.,-0.765348465884739));
#33267=CARTESIAN_POINT('Ctrl Pts',(-1.91287765805174,1.,-0.765348465884739));
#33268=CARTESIAN_POINT('Ctrl Pts',(-1.91906491634197,-1.,-0.765066729667095));
#33269=CARTESIAN_POINT('Ctrl Pts',(-1.91906491634197,1.,-0.765066729667095));
#33270=CARTESIAN_POINT('Ctrl Pts',(-1.92526263537041,-1.,-0.764740025488189));
#33271=CARTESIAN_POINT('Ctrl Pts',(-1.92526263537041,1.,-0.764740025488189));
#33272=CARTESIAN_POINT('Ctrl Pts',(-1.93147105496367,-1.,-0.764369010673889));
#33273=CARTESIAN_POINT('Ctrl Pts',(-1.93147105496367,1.,-0.764369010673889));
#33274=CARTESIAN_POINT('Ctrl Pts',(-1.93768964875867,-1.,-0.763954049121393));
#33275=CARTESIAN_POINT('Ctrl Pts',(-1.93768964875867,1.,-0.763954049121393));
#33276=CARTESIAN_POINT('Ctrl Pts',(-1.94391746617626,-1.,-0.76349533353858));
#33277=CARTESIAN_POINT('Ctrl Pts',(-1.94391746617626,1.,-0.76349533353858));
#33278=CARTESIAN_POINT('Ctrl Pts',(-1.95015342590025,-1.,-0.762992990878774));
#33279=CARTESIAN_POINT('Ctrl Pts',(-1.95015342590025,1.,-0.762992990878774));
#33280=CARTESIAN_POINT('Ctrl Pts',(-1.95639665309893,-1.,-0.762447203806263));
#33281=CARTESIAN_POINT('Ctrl Pts',(-1.95639665309893,1.,-0.762447203806263));
#33282=CARTESIAN_POINT('Ctrl Pts',(-1.96264672744229,-1.,-0.761858300014575));
#33283=CARTESIAN_POINT('Ctrl Pts',(-1.96264672744229,1.,-0.761858300014575));
#33284=CARTESIAN_POINT('Ctrl Pts',(-1.96890351582545,-1.,-0.761226690483986));
#33285=CARTESIAN_POINT('Ctrl Pts',(-1.96890351582545,1.,-0.761226690483986));
#33286=CARTESIAN_POINT('Ctrl Pts',(-1.97516705321521,-1.,-0.760552825409855));
#33287=CARTESIAN_POINT('Ctrl Pts',(-1.97516705321521,1.,-0.760552825409855));
#33288=CARTESIAN_POINT('Ctrl Pts',(-1.98143741418156,-1.,-0.759837147452135));
#33289=CARTESIAN_POINT('Ctrl Pts',(-1.98143741418156,1.,-0.759837147452135));
#33290=CARTESIAN_POINT('Ctrl Pts',(-1.98771456680806,-1.,-0.759080037802242));
#33291=CARTESIAN_POINT('Ctrl Pts',(-1.98771456680806,1.,-0.759080037802242));
#33292=CARTESIAN_POINT('Ctrl Pts',(-1.9939983109871,-1.,-0.758281796766377));
#33293=CARTESIAN_POINT('Ctrl Pts',(-1.9939983109871,1.,-0.758281796766377));
#33294=CARTESIAN_POINT('Ctrl Pts',(-2.00028834739072,-1.,-0.757442676862341));
#33295=CARTESIAN_POINT('Ctrl Pts',(-2.00028834739072,1.,-0.757442676862341));
#33296=CARTESIAN_POINT('Ctrl Pts',(-2.00658431587682,-1.,-0.756562904646496));
#33297=CARTESIAN_POINT('Ctrl Pts',(-2.00658431587682,1.,-0.756562904646496));
#33298=CARTESIAN_POINT('Ctrl Pts',(-2.01288584328149,-1.,-0.7556427049581));
#33299=CARTESIAN_POINT('Ctrl Pts',(-2.01288584328149,1.,-0.7556427049581));
#33300=CARTESIAN_POINT('Ctrl Pts',(-2.01919259406003,-1.,-0.75468233072352));
#33301=CARTESIAN_POINT('Ctrl Pts',(-2.01919259406003,1.,-0.75468233072352));
#33302=CARTESIAN_POINT('Ctrl Pts',(-2.02550428623587,-1.,-0.753682061113765));
#33303=CARTESIAN_POINT('Ctrl Pts',(-2.02550428623587,1.,-0.753682061113765));
#33304=CARTESIAN_POINT('Ctrl Pts',(-2.03182068456467,-1.,-0.752642180488104));
#33305=CARTESIAN_POINT('Ctrl Pts',(-2.03182068456467,1.,-0.752642180488104));
#33306=CARTESIAN_POINT('Ctrl Pts',(-2.03814160092173,-1.,-0.751562963361383));
#33307=CARTESIAN_POINT('Ctrl Pts',(-2.03814160092173,1.,-0.751562963361383));
#33308=CARTESIAN_POINT('Ctrl Pts',(-2.04446689147754,-1.,-0.750444657874758));
#33309=CARTESIAN_POINT('Ctrl Pts',(-2.04446689147754,1.,-0.750444657874758));
#33310=CARTESIAN_POINT('Ctrl Pts',(-2.05079645591606,-1.,-0.749287468663053));
#33311=CARTESIAN_POINT('Ctrl Pts',(-2.05079645591606,1.,-0.749287468663053));
#33312=CARTESIAN_POINT('Ctrl Pts',(-2.05713023030263,-1.,-0.748091554181101));
#33313=CARTESIAN_POINT('Ctrl Pts',(-2.05713023030263,1.,-0.748091554181101));
#33314=CARTESIAN_POINT('Ctrl Pts',(-2.06220058927162,-1.,-0.747103932785504));
#33315=CARTESIAN_POINT('Ctrl Pts',(-2.06220058927162,1.,-0.747103932785504));
#33316=CARTESIAN_POINT('Ctrl Pts',(-2.06600523016401,-1.,-0.746345871542695));
#33317=CARTESIAN_POINT('Ctrl Pts',(-2.06600523016401,1.,-0.746345871542695));
#33318=CARTESIAN_POINT('Ctrl Pts',(-2.06854248895575,-1.,-0.74583279137781));
#33319=CARTESIAN_POINT('Ctrl Pts',(-2.06854248895575,1.,-0.74583279137781));
#33320=CARTESIAN_POINT('Ctrl Pts',(-2.0698113262342,-1.,-0.745574324794401));
#33321=CARTESIAN_POINT('Ctrl Pts',(-2.0698113262342,1.,-0.745574324794401));
#33322=CARTESIAN_POINT('',(-1.60662857109684,1.,-0.693717979106306));
#33323=CARTESIAN_POINT('Ctrl Pts',(-1.60662857109684,1.,-0.693717979106306));
#33324=CARTESIAN_POINT('Ctrl Pts',(-1.61106790958151,1.,-0.695712097881194));
#33325=CARTESIAN_POINT('Ctrl Pts',(-1.61974673472612,1.,-0.699605146405088));
#33326=CARTESIAN_POINT('Ctrl Pts',(-1.63216541664676,1.,-0.705159151988319));
#33327=CARTESIAN_POINT('Ctrl Pts',(-1.64752408832016,1.,-0.711993139355394));
#33328=CARTESIAN_POINT('Ctrl Pts',(-1.6647288055568,1.,-0.719585433804282));
#33329=CARTESIAN_POINT('Ctrl Pts',(-1.67996158455503,1.,-0.726235967997433));
#33330=CARTESIAN_POINT('Ctrl Pts',(-1.69326921975743,1.,-0.731963238697195));
#33331=CARTESIAN_POINT('Ctrl Pts',(-1.70473309006121,1.,-0.736799665724771));
#33332=CARTESIAN_POINT('Ctrl Pts',(-1.71447789751927,1.,-0.740795162032087));
#33333=CARTESIAN_POINT('Ctrl Pts',(-1.7226822991693,1.,-0.744021445433764));
#33334=CARTESIAN_POINT('Ctrl Pts',(-1.72958533647399,1.,-0.746574710096436));
#33335=CARTESIAN_POINT('Ctrl Pts',(-1.73550351679848,1.,-0.748582462954854));
#33336=CARTESIAN_POINT('Ctrl Pts',(-1.74080458266705,1.,-0.75019343597954));
#33337=CARTESIAN_POINT('Ctrl Pts',(-1.74585086852298,1.,-0.751555614163629));
#33338=CARTESIAN_POINT('Ctrl Pts',(-1.75095139468809,1.,-0.752797683531377));
#33339=CARTESIAN_POINT('Ctrl Pts',(-1.75631083600175,1.,-0.75400925402848));
#33340=CARTESIAN_POINT('Ctrl Pts',(-1.7619781724032,1.,-0.755220979975262));
#33341=CARTESIAN_POINT('Ctrl Pts',(-1.76789396003141,1.,-0.756421896028403));
#33342=CARTESIAN_POINT('Ctrl Pts',(-1.77394167108342,1.,-0.757578264077238));
#33343=CARTESIAN_POINT('Ctrl Pts',(-1.77999411220912,1.,-0.75865062667738));
#33344=CARTESIAN_POINT('Ctrl Pts',(-1.78596964884526,1.,-0.759614401109868));
#33345=CARTESIAN_POINT('Ctrl Pts',(-1.79185815610802,1.,-0.760469555880425));
#33346=CARTESIAN_POINT('Ctrl Pts',(-1.79768986997735,1.,-0.761229695230359));
#33347=CARTESIAN_POINT('Ctrl Pts',(-1.80351583877334,1.,-0.761915336443515));
#33348=CARTESIAN_POINT('Ctrl Pts',(-1.80938551463989,1.,-0.762546129464036));
#33349=CARTESIAN_POINT('Ctrl Pts',(-1.81532118405566,1.,-0.763132003836783));
#33350=CARTESIAN_POINT('Ctrl Pts',(-1.82131873145297,1.,-0.763673465462854));
#33351=CARTESIAN_POINT('Ctrl Pts',(-1.8273599120008,1.,-0.764165902606055));
#33352=CARTESIAN_POINT('Ctrl Pts',(-1.8334207722714,1.,-0.764602549687845));
#33353=CARTESIAN_POINT('Ctrl Pts',(-1.83948181064823,1.,-0.764978057881687));
#33354=CARTESIAN_POINT('Ctrl Pts',(-1.8455369887591,1.,-0.765291664861971));
#33355=CARTESIAN_POINT('Ctrl Pts',(-1.85158945130054,1.,-0.765545710619023));
#33356=CARTESIAN_POINT('Ctrl Pts',(-1.85764741390391,1.,-0.765744212909305));
#33357=CARTESIAN_POINT('Ctrl Pts',(-1.86372027063314,1.,-0.765891519092557));
#33358=CARTESIAN_POINT('Ctrl Pts',(-1.86981398314345,1.,-0.765990708546111));
#33359=CARTESIAN_POINT('Ctrl Pts',(-1.87592888967886,1.,-0.766042837036759));
#33360=CARTESIAN_POINT('Ctrl Pts',(-1.88206215302561,1.,-0.766047794851868));
#33361=CARTESIAN_POINT('Ctrl Pts',(-1.88820926433409,1.,-0.76600483706209));
#33362=CARTESIAN_POINT('Ctrl Pts',(-1.89436577771389,1.,-0.765913193856979));
#33363=CARTESIAN_POINT('Ctrl Pts',(-1.90052930393599,1.,-0.765772772593395));
#33364=CARTESIAN_POINT('Ctrl Pts',(-1.90669961402362,1.,-0.765584196937936));
#33365=CARTESIAN_POINT('Ctrl Pts',(-1.91287765805174,1.,-0.765348465884739));
#33366=CARTESIAN_POINT('Ctrl Pts',(-1.91906491634197,1.,-0.765066729667095));
#33367=CARTESIAN_POINT('Ctrl Pts',(-1.92526263537041,1.,-0.764740025488189));
#33368=CARTESIAN_POINT('Ctrl Pts',(-1.93147105496367,1.,-0.764369010673889));
#33369=CARTESIAN_POINT('Ctrl Pts',(-1.93768964875867,1.,-0.763954049121393));
#33370=CARTESIAN_POINT('Ctrl Pts',(-1.94391746617626,1.,-0.76349533353858));
#33371=CARTESIAN_POINT('Ctrl Pts',(-1.95015342590025,1.,-0.762992990878774));
#33372=CARTESIAN_POINT('Ctrl Pts',(-1.95639665309893,1.,-0.762447203806263));
#33373=CARTESIAN_POINT('Ctrl Pts',(-1.96264672744229,1.,-0.761858300014575));
#33374=CARTESIAN_POINT('Ctrl Pts',(-1.96890351582545,1.,-0.761226690483986));
#33375=CARTESIAN_POINT('Ctrl Pts',(-1.97516705321521,1.,-0.760552825409855));
#33376=CARTESIAN_POINT('Ctrl Pts',(-1.98143741418156,1.,-0.759837147452135));
#33377=CARTESIAN_POINT('Ctrl Pts',(-1.98771456680806,1.,-0.759080037802242));
#33378=CARTESIAN_POINT('Ctrl Pts',(-1.9939983109871,1.,-0.758281796766377));
#33379=CARTESIAN_POINT('Ctrl Pts',(-2.00028834739072,1.,-0.757442676862341));
#33380=CARTESIAN_POINT('Ctrl Pts',(-2.00658431587682,1.,-0.756562904646496));
#33381=CARTESIAN_POINT('Ctrl Pts',(-2.01288584328149,1.,-0.7556427049581));
#33382=CARTESIAN_POINT('Ctrl Pts',(-2.01919259406003,1.,-0.75468233072352));
#33383=CARTESIAN_POINT('Ctrl Pts',(-2.02550428623587,1.,-0.753682061113765));
#33384=CARTESIAN_POINT('Ctrl Pts',(-2.03182068456467,1.,-0.752642180488104));
#33385=CARTESIAN_POINT('Ctrl Pts',(-2.03814160092173,1.,-0.751562963361383));
#33386=CARTESIAN_POINT('Ctrl Pts',(-2.04446689147754,1.,-0.750444657874758));
#33387=CARTESIAN_POINT('Ctrl Pts',(-2.05079645591606,1.,-0.749287468663053));
#33388=CARTESIAN_POINT('Ctrl Pts',(-2.05713023030263,1.,-0.748091554181101));
#33389=CARTESIAN_POINT('Ctrl Pts',(-2.06220058927162,1.,-0.747103932785504));
#33390=CARTESIAN_POINT('Ctrl Pts',(-2.06600523016401,1.,-0.746345871542695));
#33391=CARTESIAN_POINT('Ctrl Pts',(-2.06854248895575,1.,-0.74583279137781));
#33392=CARTESIAN_POINT('Ctrl Pts',(-2.0698113262342,1.,-0.745574324794401));
#33393=CARTESIAN_POINT('',(-1.60662857109684,0.,-0.693717979106306));
#33394=CARTESIAN_POINT('Origin',(0.,0.,0.));
#33395=CARTESIAN_POINT('',(-1.5055822144029,1.,-0.892032620296855));
#33396=CARTESIAN_POINT('Origin',(0.,1.,0.));
#33397=CARTESIAN_POINT('',(-1.5055822144029,0.,-0.892032620296855));
#33398=CARTESIAN_POINT('Ctrl Pts',(-1.81978687191668,-1.,-1.23627494547115));
#33399=CARTESIAN_POINT('Ctrl Pts',(-1.81978687191668,1.,-1.23627494547115));
#33400=CARTESIAN_POINT('Ctrl Pts',(-1.81925017193666,-1.,-1.23509651170476));
#33401=CARTESIAN_POINT('Ctrl Pts',(-1.81925017193666,1.,-1.23509651170476));
#33402=CARTESIAN_POINT('Ctrl Pts',(-1.81817389921279,-1.,-1.2327422452705));
#33403=CARTESIAN_POINT('Ctrl Pts',(-1.81817389921279,1.,-1.2327422452705));
#33404=CARTESIAN_POINT('Ctrl Pts',(-1.8165508718364,-1.,-1.2292186489137));
#33405=CARTESIAN_POINT('Ctrl Pts',(-1.8165508718364,1.,-1.2292186489137));
#33406=CARTESIAN_POINT('Ctrl Pts',(-1.81436959210434,-1.,-1.2245361330495));
#33407=CARTESIAN_POINT('Ctrl Pts',(-1.81436959210434,1.,-1.2245361330495));
#33408=CARTESIAN_POINT('Ctrl Pts',(-1.81161420806656,-1.,-1.21870906103557));
#33409=CARTESIAN_POINT('Ctrl Pts',(-1.81161420806656,1.,-1.21870906103557));
#33410=CARTESIAN_POINT('Ctrl Pts',(-1.80882996917129,-1.,-1.21290815708314));
#33411=CARTESIAN_POINT('Ctrl Pts',(-1.80882996917129,1.,-1.21290815708314));
#33412=CARTESIAN_POINT('Ctrl Pts',(-1.80601678480707,-1.,-1.20713356605475));
#33413=CARTESIAN_POINT('Ctrl Pts',(-1.80601678480707,1.,-1.20713356605475));
#33414=CARTESIAN_POINT('Ctrl Pts',(-1.80317454838603,-1.,-1.20138548938974));
#33415=CARTESIAN_POINT('Ctrl Pts',(-1.80317454838603,1.,-1.20138548938974));
#33416=CARTESIAN_POINT('Ctrl Pts',(-1.80030314369879,-1.,-1.19566418930242));
#33417=CARTESIAN_POINT('Ctrl Pts',(-1.80030314369879,1.,-1.19566418930242));
#33418=CARTESIAN_POINT('Ctrl Pts',(-1.79740245923478,-1.,-1.18996997934445));
#33419=CARTESIAN_POINT('Ctrl Pts',(-1.79740245923478,1.,-1.18996997934445));
#33420=CARTESIAN_POINT('Ctrl Pts',(-1.79447240321515,-1.,-1.18430321697432));
#33421=CARTESIAN_POINT('Ctrl Pts',(-1.79447240321515,1.,-1.18430321697432));
#33422=CARTESIAN_POINT('Ctrl Pts',(-1.79151291552689,-1.,-1.17866429440809));
#33423=CARTESIAN_POINT('Ctrl Pts',(-1.79151291552689,1.,-1.17866429440809));
#33424=CARTESIAN_POINT('Ctrl Pts',(-1.78852398877616,-1.,-1.17305363177328));
#33425=CARTESIAN_POINT('Ctrl Pts',(-1.78852398877616,1.,-1.17305363177328));
#33426=CARTESIAN_POINT('Ctrl Pts',(-1.78550566040443,-1.,-1.16747166312303));
#33427=CARTESIAN_POINT('Ctrl Pts',(-1.78550566040443,1.,-1.16747166312303));
#33428=CARTESIAN_POINT('Ctrl Pts',(-1.78245795881009,-1.,-1.16191881298499));
#33429=CARTESIAN_POINT('Ctrl Pts',(-1.78245795881009,1.,-1.16191881298499));
#33430=CARTESIAN_POINT('Ctrl Pts',(-1.77938085564275,-1.,-1.15639547194698));
#33431=CARTESIAN_POINT('Ctrl Pts',(-1.77938085564275,1.,-1.15639547194698));
#33432=CARTESIAN_POINT('Ctrl Pts',(-1.7762742255701,-1.,-1.15090197841515));
#33433=CARTESIAN_POINT('Ctrl Pts',(-1.7762742255701,1.,-1.15090197841515));
#33434=CARTESIAN_POINT('Ctrl Pts',(-1.77313777896194,-1.,-1.1454385822692));
#33435=CARTESIAN_POINT('Ctrl Pts',(-1.77313777896194,1.,-1.1454385822692));
#33436=CARTESIAN_POINT('Ctrl Pts',(-1.76997111386769,-1.,-1.14000548336975));
#33437=CARTESIAN_POINT('Ctrl Pts',(-1.76997111386769,1.,-1.14000548336975));
#33438=CARTESIAN_POINT('Ctrl Pts',(-1.76677384551862,-1.,-1.1346029180462));
#33439=CARTESIAN_POINT('Ctrl Pts',(-1.76677384551862,1.,-1.1346029180462));
#33440=CARTESIAN_POINT('Ctrl Pts',(-1.7635457196617,-1.,-1.12923123555075));
#33441=CARTESIAN_POINT('Ctrl Pts',(-1.7635457196617,1.,-1.12923123555075));
#33442=CARTESIAN_POINT('Ctrl Pts',(-1.76028671825096,-1.,-1.12389096855086));
#33443=CARTESIAN_POINT('Ctrl Pts',(-1.76028671825096,1.,-1.12389096855086));
#33444=CARTESIAN_POINT('Ctrl Pts',(-1.75699720772105,-1.,-1.11858293216763));
#33445=CARTESIAN_POINT('Ctrl Pts',(-1.75699720772105,1.,-1.11858293216763));
#33446=CARTESIAN_POINT('Ctrl Pts',(-1.7536777209463,-1.,-1.11330807582551));
#33447=CARTESIAN_POINT('Ctrl Pts',(-1.7536777209463,1.,-1.11330807582551));
#33448=CARTESIAN_POINT('Ctrl Pts',(-1.7503286607592,-1.,-1.10806728183007));
#33449=CARTESIAN_POINT('Ctrl Pts',(-1.7503286607592,1.,-1.10806728183007));
#33450=CARTESIAN_POINT('Ctrl Pts',(-1.74695004214923,-1.,-1.10286118991143));
#33451=CARTESIAN_POINT('Ctrl Pts',(-1.74695004214923,1.,-1.10286118991143));
#33452=CARTESIAN_POINT('Ctrl Pts',(-1.74354119236208,-1.,-1.09768999241225));
#33453=CARTESIAN_POINT('Ctrl Pts',(-1.74354119236208,1.,-1.09768999241225));
#33454=CARTESIAN_POINT('Ctrl Pts',(-1.74010053962247,-1.,-1.09255329056493));
#33455=CARTESIAN_POINT('Ctrl Pts',(-1.74010053962247,1.,-1.09255329056493));
#33456=CARTESIAN_POINT('Ctrl Pts',(-1.73662628326091,-1.,-1.08745056285427));
#33457=CARTESIAN_POINT('Ctrl Pts',(-1.73662628326091,1.,-1.08745056285427));
#33458=CARTESIAN_POINT('Ctrl Pts',(-1.73311705663407,-1.,-1.08238162784749));
#33459=CARTESIAN_POINT('Ctrl Pts',(-1.73311705663407,1.,-1.08238162784749));
#33460=CARTESIAN_POINT('Ctrl Pts',(-1.72957248977424,-1.,-1.0773470373727));
#33461=CARTESIAN_POINT('Ctrl Pts',(-1.72957248977424,1.,-1.0773470373727));
#33462=CARTESIAN_POINT('Ctrl Pts',(-1.72599406198488,-1.,-1.07234866990252));
#33463=CARTESIAN_POINT('Ctrl Pts',(-1.72599406198488,1.,-1.07234866990252));
#33464=CARTESIAN_POINT('Ctrl Pts',(-1.72238500928453,-1.,-1.06738966975462));
#33465=CARTESIAN_POINT('Ctrl Pts',(-1.72238500928453,1.,-1.06738966975462));
#33466=CARTESIAN_POINT('Ctrl Pts',(-1.71874858456904,-1.,-1.06247324680647));
#33467=CARTESIAN_POINT('Ctrl Pts',(-1.71874858456904,1.,-1.06247324680647));
#33468=CARTESIAN_POINT('Ctrl Pts',(-1.7150865442702,-1.,-1.05760163192479));
#33469=CARTESIAN_POINT('Ctrl Pts',(-1.7150865442702,1.,-1.05760163192479));
#33470=CARTESIAN_POINT('Ctrl Pts',(-1.71139783543989,-1.,-1.05277517202855));
#33471=CARTESIAN_POINT('Ctrl Pts',(-1.71139783543989,1.,-1.05277517202855));
#33472=CARTESIAN_POINT('Ctrl Pts',(-1.70767646263649,-1.,-1.04799085404995));
#33473=CARTESIAN_POINT('Ctrl Pts',(-1.70767646263649,1.,-1.04799085404995));
#33474=CARTESIAN_POINT('Ctrl Pts',(-1.70391338707982,-1.,-1.04324363334554));
#33475=CARTESIAN_POINT('Ctrl Pts',(-1.70391338707982,1.,-1.04324363334554));
#33476=CARTESIAN_POINT('Ctrl Pts',(-1.70010052930962,-1.,-1.03852922490789));
#33477=CARTESIAN_POINT('Ctrl Pts',(-1.70010052930962,1.,-1.03852922490789));
#33478=CARTESIAN_POINT('Ctrl Pts',(-1.69623414782771,-1.,-1.03384646003588));
#33479=CARTESIAN_POINT('Ctrl Pts',(-1.69623414782771,1.,-1.03384646003588));
#33480=CARTESIAN_POINT('Ctrl Pts',(-1.69231840863458,-1.,-1.02919977579147));
#33481=CARTESIAN_POINT('Ctrl Pts',(-1.69231840863458,1.,-1.02919977579147));
#33482=CARTESIAN_POINT('Ctrl Pts',(-1.68836910178447,-1.,-1.02460180535255));
#33483=CARTESIAN_POINT('Ctrl Pts',(-1.68836910178447,1.,-1.02460180535255));
#33484=CARTESIAN_POINT('Ctrl Pts',(-1.68440578021706,-1.,-1.02006795074201));
#33485=CARTESIAN_POINT('Ctrl Pts',(-1.68440578021706,1.,-1.02006795074201));
#33486=CARTESIAN_POINT('Ctrl Pts',(-1.68044289894798,-1.,-1.01561026162773));
#33487=CARTESIAN_POINT('Ctrl Pts',(-1.68044289894798,1.,-1.01561026162773));
#33488=CARTESIAN_POINT('Ctrl Pts',(-1.67648246776464,-1.,-1.01123236493511));
#33489=CARTESIAN_POINT('Ctrl Pts',(-1.67648246776464,1.,-1.01123236493511));
#33490=CARTESIAN_POINT('Ctrl Pts',(-1.67250335383293,-1.,-1.00692206696414));
#33491=CARTESIAN_POINT('Ctrl Pts',(-1.67250335383293,1.,-1.00692206696414));
#33492=CARTESIAN_POINT('Ctrl Pts',(-1.66846059277303,-1.,-1.00265091003727));
#33493=CARTESIAN_POINT('Ctrl Pts',(-1.66846059277303,1.,-1.00265091003727));
#33494=CARTESIAN_POINT('Ctrl Pts',(-1.66430758030376,-1.,-0.998389654952758));
#33495=CARTESIAN_POINT('Ctrl Pts',(-1.66430758030376,1.,-0.998389654952758));
#33496=CARTESIAN_POINT('Ctrl Pts',(-1.66001553809947,-1.,-0.994121836661306));
#33497=CARTESIAN_POINT('Ctrl Pts',(-1.66001553809947,1.,-0.994121836661306));
#33498=CARTESIAN_POINT('Ctrl Pts',(-1.65559044289699,-1.,-0.989855627854165));
#33499=CARTESIAN_POINT('Ctrl Pts',(-1.65559044289699,1.,-0.989855627854165));
#33500=CARTESIAN_POINT('Ctrl Pts',(-1.65110016612638,-1.,-0.985642622920821));
#33501=CARTESIAN_POINT('Ctrl Pts',(-1.65110016612638,1.,-0.985642622920821));
#33502=CARTESIAN_POINT('Ctrl Pts',(-1.64665139190656,-1.,-0.981562530939489));
#33503=CARTESIAN_POINT('Ctrl Pts',(-1.64665139190656,1.,-0.981562530939489));
#33504=CARTESIAN_POINT('Ctrl Pts',(-1.64233990826687,-1.,-0.977689794119416));
#33505=CARTESIAN_POINT('Ctrl Pts',(-1.64233990826687,1.,-0.977689794119416));
#33506=CARTESIAN_POINT('Ctrl Pts',(-1.63820952658144,-1.,-0.974066058287418));
#33507=CARTESIAN_POINT('Ctrl Pts',(-1.63820952658144,1.,-0.974066058287418));
#33508=CARTESIAN_POINT('Ctrl Pts',(-1.63420665729798,-1.,-0.970669715997509));
#33509=CARTESIAN_POINT('Ctrl Pts',(-1.63420665729798,1.,-0.970669715997509));
#33510=CARTESIAN_POINT('Ctrl Pts',(-1.63013849959461,-1.,-0.967387853230345));
#33511=CARTESIAN_POINT('Ctrl Pts',(-1.63013849959461,1.,-0.967387853230345));
#33512=CARTESIAN_POINT('Ctrl Pts',(-1.62571930670187,-1.,-0.964046107040536));
#33513=CARTESIAN_POINT('Ctrl Pts',(-1.62571930670187,1.,-0.964046107040536));
#33514=CARTESIAN_POINT('Ctrl Pts',(-1.62061638140221,-1.,-0.960438326101729));
#33515=CARTESIAN_POINT('Ctrl Pts',(-1.62061638140221,1.,-0.960438326101729));
#33516=CARTESIAN_POINT('Ctrl Pts',(-1.61449324337085,-1.,-0.956354422920671));
#33517=CARTESIAN_POINT('Ctrl Pts',(-1.61449324337085,1.,-0.956354422920671));
#33518=CARTESIAN_POINT('Ctrl Pts',(-1.60706069896936,-1.,-0.951613284356035));
#33519=CARTESIAN_POINT('Ctrl Pts',(-1.60706069896936,1.,-0.951613284356035));
#33520=CARTESIAN_POINT('Ctrl Pts',(-1.59810042043673,-1.,-0.946078063315257));
#33521=CARTESIAN_POINT('Ctrl Pts',(-1.59810042043673,1.,-0.946078063315257));
#33522=CARTESIAN_POINT('Ctrl Pts',(-1.58744937487176,-1.,-0.939646377893399));
#33523=CARTESIAN_POINT('Ctrl Pts',(-1.58744937487176,1.,-0.939646377893399));
#33524=CARTESIAN_POINT('Ctrl Pts',(-1.57499388382243,-1.,-0.932246680108685));
#33525=CARTESIAN_POINT('Ctrl Pts',(-1.57499388382243,1.,-0.932246680108685));
#33526=CARTESIAN_POINT('Ctrl Pts',(-1.56065988578893,-1.,-0.923832188944341));
#33527=CARTESIAN_POINT('Ctrl Pts',(-1.56065988578893,1.,-0.923832188944341));
#33528=CARTESIAN_POINT('Ctrl Pts',(-1.54440491149498,-1.,-0.914375919026456));
#33529=CARTESIAN_POINT('Ctrl Pts',(-1.54440491149498,1.,-0.914375919026456));
#33530=CARTESIAN_POINT('Ctrl Pts',(-1.52984849887993,-1.,-0.905967409625651));
#33531=CARTESIAN_POINT('Ctrl Pts',(-1.52984849887993,1.,-0.905967409625651));
#33532=CARTESIAN_POINT('Ctrl Pts',(-1.51805569590094,-1.,-0.899185047483511));
#33533=CARTESIAN_POINT('Ctrl Pts',(-1.51805569590094,1.,-0.899185047483511));
#33534=CARTESIAN_POINT('Ctrl Pts',(-1.50980486806688,-1.,-0.894452006964543));
#33535=CARTESIAN_POINT('Ctrl Pts',(-1.50980486806688,1.,-0.894452006964543));
#33536=CARTESIAN_POINT('Ctrl Pts',(-1.5055822144029,-1.,-0.892032620296855));
#33537=CARTESIAN_POINT('Ctrl Pts',(-1.5055822144029,1.,-0.892032620296855));
#33538=CARTESIAN_POINT('',(-1.81978687191668,1.,-1.23627494547115));
#33539=CARTESIAN_POINT('Ctrl Pts',(-1.81978687191668,1.,-1.23627494547115));
#33540=CARTESIAN_POINT('Ctrl Pts',(-1.81925017193666,1.,-1.23509651170476));
#33541=CARTESIAN_POINT('Ctrl Pts',(-1.81817389921279,1.,-1.2327422452705));
#33542=CARTESIAN_POINT('Ctrl Pts',(-1.8165508718364,1.,-1.2292186489137));
#33543=CARTESIAN_POINT('Ctrl Pts',(-1.81436959210434,1.,-1.2245361330495));
#33544=CARTESIAN_POINT('Ctrl Pts',(-1.81161420806656,1.,-1.21870906103557));
#33545=CARTESIAN_POINT('Ctrl Pts',(-1.80882996917129,1.,-1.21290815708314));
#33546=CARTESIAN_POINT('Ctrl Pts',(-1.80601678480707,1.,-1.20713356605475));
#33547=CARTESIAN_POINT('Ctrl Pts',(-1.80317454838603,1.,-1.20138548938974));
#33548=CARTESIAN_POINT('Ctrl Pts',(-1.80030314369879,1.,-1.19566418930242));
#33549=CARTESIAN_POINT('Ctrl Pts',(-1.79740245923478,1.,-1.18996997934445));
#33550=CARTESIAN_POINT('Ctrl Pts',(-1.79447240321515,1.,-1.18430321697432));
#33551=CARTESIAN_POINT('Ctrl Pts',(-1.79151291552689,1.,-1.17866429440809));
#33552=CARTESIAN_POINT('Ctrl Pts',(-1.78852398877616,1.,-1.17305363177328));
#33553=CARTESIAN_POINT('Ctrl Pts',(-1.78550566040443,1.,-1.16747166312303));
#33554=CARTESIAN_POINT('Ctrl Pts',(-1.78245795881009,1.,-1.16191881298499));
#33555=CARTESIAN_POINT('Ctrl Pts',(-1.77938085564275,1.,-1.15639547194698));
#33556=CARTESIAN_POINT('Ctrl Pts',(-1.7762742255701,1.,-1.15090197841515));
#33557=CARTESIAN_POINT('Ctrl Pts',(-1.77313777896194,1.,-1.1454385822692));
#33558=CARTESIAN_POINT('Ctrl Pts',(-1.76997111386769,1.,-1.14000548336975));
#33559=CARTESIAN_POINT('Ctrl Pts',(-1.76677384551862,1.,-1.1346029180462));
#33560=CARTESIAN_POINT('Ctrl Pts',(-1.7635457196617,1.,-1.12923123555075));
#33561=CARTESIAN_POINT('Ctrl Pts',(-1.76028671825096,1.,-1.12389096855086));
#33562=CARTESIAN_POINT('Ctrl Pts',(-1.75699720772105,1.,-1.11858293216763));
#33563=CARTESIAN_POINT('Ctrl Pts',(-1.7536777209463,1.,-1.11330807582551));
#33564=CARTESIAN_POINT('Ctrl Pts',(-1.7503286607592,1.,-1.10806728183007));
#33565=CARTESIAN_POINT('Ctrl Pts',(-1.74695004214923,1.,-1.10286118991143));
#33566=CARTESIAN_POINT('Ctrl Pts',(-1.74354119236208,1.,-1.09768999241225));
#33567=CARTESIAN_POINT('Ctrl Pts',(-1.74010053962247,1.,-1.09255329056493));
#33568=CARTESIAN_POINT('Ctrl Pts',(-1.73662628326091,1.,-1.08745056285427));
#33569=CARTESIAN_POINT('Ctrl Pts',(-1.73311705663407,1.,-1.08238162784749));
#33570=CARTESIAN_POINT('Ctrl Pts',(-1.72957248977424,1.,-1.0773470373727));
#33571=CARTESIAN_POINT('Ctrl Pts',(-1.72599406198488,1.,-1.07234866990252));
#33572=CARTESIAN_POINT('Ctrl Pts',(-1.72238500928453,1.,-1.06738966975462));
#33573=CARTESIAN_POINT('Ctrl Pts',(-1.71874858456904,1.,-1.06247324680647));
#33574=CARTESIAN_POINT('Ctrl Pts',(-1.7150865442702,1.,-1.05760163192479));
#33575=CARTESIAN_POINT('Ctrl Pts',(-1.71139783543989,1.,-1.05277517202855));
#33576=CARTESIAN_POINT('Ctrl Pts',(-1.70767646263649,1.,-1.04799085404995));
#33577=CARTESIAN_POINT('Ctrl Pts',(-1.70391338707982,1.,-1.04324363334554));
#33578=CARTESIAN_POINT('Ctrl Pts',(-1.70010052930962,1.,-1.03852922490789));
#33579=CARTESIAN_POINT('Ctrl Pts',(-1.69623414782771,1.,-1.03384646003588));
#33580=CARTESIAN_POINT('Ctrl Pts',(-1.69231840863458,1.,-1.02919977579147));
#33581=CARTESIAN_POINT('Ctrl Pts',(-1.68836910178447,1.,-1.02460180535255));
#33582=CARTESIAN_POINT('Ctrl Pts',(-1.68440578021706,1.,-1.02006795074201));
#33583=CARTESIAN_POINT('Ctrl Pts',(-1.68044289894798,1.,-1.01561026162773));
#33584=CARTESIAN_POINT('Ctrl Pts',(-1.67648246776464,1.,-1.01123236493511));
#33585=CARTESIAN_POINT('Ctrl Pts',(-1.67250335383293,1.,-1.00692206696414));
#33586=CARTESIAN_POINT('Ctrl Pts',(-1.66846059277303,1.,-1.00265091003727));
#33587=CARTESIAN_POINT('Ctrl Pts',(-1.66430758030376,1.,-0.998389654952758));
#33588=CARTESIAN_POINT('Ctrl Pts',(-1.66001553809947,1.,-0.994121836661306));
#33589=CARTESIAN_POINT('Ctrl Pts',(-1.65559044289699,1.,-0.989855627854165));
#33590=CARTESIAN_POINT('Ctrl Pts',(-1.65110016612638,1.,-0.985642622920821));
#33591=CARTESIAN_POINT('Ctrl Pts',(-1.64665139190656,1.,-0.981562530939489));
#33592=CARTESIAN_POINT('Ctrl Pts',(-1.64233990826687,1.,-0.977689794119416));
#33593=CARTESIAN_POINT('Ctrl Pts',(-1.63820952658144,1.,-0.974066058287418));
#33594=CARTESIAN_POINT('Ctrl Pts',(-1.63420665729798,1.,-0.970669715997509));
#33595=CARTESIAN_POINT('Ctrl Pts',(-1.63013849959461,1.,-0.967387853230345));
#33596=CARTESIAN_POINT('Ctrl Pts',(-1.62571930670187,1.,-0.964046107040536));
#33597=CARTESIAN_POINT('Ctrl Pts',(-1.62061638140221,1.,-0.960438326101729));
#33598=CARTESIAN_POINT('Ctrl Pts',(-1.61449324337085,1.,-0.956354422920671));
#33599=CARTESIAN_POINT('Ctrl Pts',(-1.60706069896936,1.,-0.951613284356035));
#33600=CARTESIAN_POINT('Ctrl Pts',(-1.59810042043673,1.,-0.946078063315257));
#33601=CARTESIAN_POINT('Ctrl Pts',(-1.58744937487176,1.,-0.939646377893399));
#33602=CARTESIAN_POINT('Ctrl Pts',(-1.57499388382243,1.,-0.932246680108685));
#33603=CARTESIAN_POINT('Ctrl Pts',(-1.56065988578893,1.,-0.923832188944341));
#33604=CARTESIAN_POINT('Ctrl Pts',(-1.54440491149498,1.,-0.914375919026456));
#33605=CARTESIAN_POINT('Ctrl Pts',(-1.52984849887993,1.,-0.905967409625651));
#33606=CARTESIAN_POINT('Ctrl Pts',(-1.51805569590094,1.,-0.899185047483511));
#33607=CARTESIAN_POINT('Ctrl Pts',(-1.50980486806688,1.,-0.894452006964543));
#33608=CARTESIAN_POINT('Ctrl Pts',(-1.5055822144029,1.,-0.892032620296855));
#33609=CARTESIAN_POINT('',(-1.81978687191668,0.,-1.23627494547115));
#33610=CARTESIAN_POINT('Origin',(-1.73811241238545,0.,-1.34869019493419));
#33611=CARTESIAN_POINT('',(-1.73811241238545,1.,-1.34869019493419));
#33612=CARTESIAN_POINT('',(-1.81978687191668,1.,-1.23627494547115));
#33613=CARTESIAN_POINT('',(-1.73811241238545,0.,-1.34869019493419));
#33614=CARTESIAN_POINT('Ctrl Pts',(-1.31362392696032,-1.,-1.15624053661742));
#33615=CARTESIAN_POINT('Ctrl Pts',(-1.31362392696032,1.,-1.15624053661742));
#33616=CARTESIAN_POINT('Ctrl Pts',(-1.31722977216397,-1.,-1.15950888730809));
#33617=CARTESIAN_POINT('Ctrl Pts',(-1.31722977216397,1.,-1.15950888730809));
#33618=CARTESIAN_POINT('Ctrl Pts',(-1.32428080721772,-1.,-1.16589330093588));
#33619=CARTESIAN_POINT('Ctrl Pts',(-1.32428080721772,1.,-1.16589330093588));
#33620=CARTESIAN_POINT('Ctrl Pts',(-1.33437539347008,-1.,-1.17501305789857));
#33621=CARTESIAN_POINT('Ctrl Pts',(-1.33437539347008,1.,-1.17501305789857));
#33622=CARTESIAN_POINT('Ctrl Pts',(-1.34687054001093,-1.,-1.18625865667441));
#33623=CARTESIAN_POINT('Ctrl Pts',(-1.34687054001093,1.,-1.18625865667441));
#33624=CARTESIAN_POINT('Ctrl Pts',(-1.36088705043885,-1.,-1.1987959077932));
#33625=CARTESIAN_POINT('Ctrl Pts',(-1.36088705043885,1.,-1.1987959077932));
#33626=CARTESIAN_POINT('Ctrl Pts',(-1.37331915607905,-1.,-1.20982812925645));
#33627=CARTESIAN_POINT('Ctrl Pts',(-1.37331915607905,1.,-1.20982812925645));
#33628=CARTESIAN_POINT('Ctrl Pts',(-1.38420564527715,-1.,-1.21938737280852));
#33629=CARTESIAN_POINT('Ctrl Pts',(-1.38420564527715,1.,-1.21938737280852));
#33630=CARTESIAN_POINT('Ctrl Pts',(-1.39361389568796,-1.,-1.22752961899387));
#33631=CARTESIAN_POINT('Ctrl Pts',(-1.39361389568796,1.,-1.22752961899387));
#33632=CARTESIAN_POINT('Ctrl Pts',(-1.40164708206106,-1.,-1.23434087290423));
#33633=CARTESIAN_POINT('Ctrl Pts',(-1.40164708206106,1.,-1.23434087290423));
#33634=CARTESIAN_POINT('Ctrl Pts',(-1.40845295531283,-1.,-1.23994455029534));
#33635=CARTESIAN_POINT('Ctrl Pts',(-1.40845295531283,1.,-1.23994455029534));
#33636=CARTESIAN_POINT('Ctrl Pts',(-1.41422913175179,-1.,-1.24450600513056));
#33637=CARTESIAN_POINT('Ctrl Pts',(-1.41422913175179,1.,-1.24450600513056));
#33638=CARTESIAN_POINT('Ctrl Pts',(-1.41923722596025,-1.,-1.24824430986571));
#33639=CARTESIAN_POINT('Ctrl Pts',(-1.41923722596025,1.,-1.24824430986571));
#33640=CARTESIAN_POINT('Ctrl Pts',(-1.42378102115575,-1.,-1.2514145557001));
#33641=CARTESIAN_POINT('Ctrl Pts',(-1.42378102115575,1.,-1.2514145557001));
#33642=CARTESIAN_POINT('Ctrl Pts',(-1.42815938799387,-1.,-1.25426945222639));
#33643=CARTESIAN_POINT('Ctrl Pts',(-1.42815938799387,1.,-1.25426945222639));
#33644=CARTESIAN_POINT('Ctrl Pts',(-1.43262645609691,-1.,-1.25702687965755));
#33645=CARTESIAN_POINT('Ctrl Pts',(-1.43262645609691,1.,-1.25702687965755));
#33646=CARTESIAN_POINT('Ctrl Pts',(-1.43734919180848,-1.,-1.25983531012005));
#33647=CARTESIAN_POINT('Ctrl Pts',(-1.43734919180848,1.,-1.25983531012005));
#33648=CARTESIAN_POINT('Ctrl Pts',(-1.44236470511303,-1.,-1.26273903323859));
#33649=CARTESIAN_POINT('Ctrl Pts',(-1.44236470511303,1.,-1.26273903323859));
#33650=CARTESIAN_POINT('Ctrl Pts',(-1.44761985001662,-1.,-1.26570925118868));
#33651=CARTESIAN_POINT('Ctrl Pts',(-1.44761985001662,1.,-1.26570925118868));
#33652=CARTESIAN_POINT('Ctrl Pts',(-1.45301422764247,-1.,-1.2686778680489));
#33653=CARTESIAN_POINT('Ctrl Pts',(-1.45301422764247,1.,-1.2686778680489));
#33654=CARTESIAN_POINT('Ctrl Pts',(-1.45843906294697,-1.,-1.27156805265289));
#33655=CARTESIAN_POINT('Ctrl Pts',(-1.45843906294697,1.,-1.27156805265289));
#33656=CARTESIAN_POINT('Ctrl Pts',(-1.46382431332476,-1.,-1.27433119897822));
#33657=CARTESIAN_POINT('Ctrl Pts',(-1.46382431332476,1.,-1.27433119897822));
#33658=CARTESIAN_POINT('Ctrl Pts',(-1.46916035917133,-1.,-1.27696414831089));
#33659=CARTESIAN_POINT('Ctrl Pts',(-1.46916035917133,1.,-1.27696414831089));
#33660=CARTESIAN_POINT('Ctrl Pts',(-1.4744717526707,-1.,-1.2794891824849));
#33661=CARTESIAN_POINT('Ctrl Pts',(-1.4744717526707,1.,-1.2794891824849));
#33662=CARTESIAN_POINT('Ctrl Pts',(-1.47980070347095,-1.,-1.28194158939517));
#33663=CARTESIAN_POINT('Ctrl Pts',(-1.47980070347095,1.,-1.28194158939517));
#33664=CARTESIAN_POINT('Ctrl Pts',(-1.4851881711891,-1.,-1.28435533880201));
#33665=CARTESIAN_POINT('Ctrl Pts',(-1.4851881711891,1.,-1.28435533880201));
#33666=CARTESIAN_POINT('Ctrl Pts',(-1.4906522831278,-1.,-1.2867467611644));
#33667=CARTESIAN_POINT('Ctrl Pts',(-1.4906522831278,1.,-1.2867467611644));
#33668=CARTESIAN_POINT('Ctrl Pts',(-1.49618896881754,-1.,-1.28911506584254));
#33669=CARTESIAN_POINT('Ctrl Pts',(-1.49618896881754,1.,-1.28911506584254));
#33670=CARTESIAN_POINT('Ctrl Pts',(-1.50178230149776,-1.,-1.29145022885181));
#33671=CARTESIAN_POINT('Ctrl Pts',(-1.50178230149776,1.,-1.29145022885181));
#33672=CARTESIAN_POINT('Ctrl Pts',(-1.50741159078365,-1.,-1.29373841372842));
#33673=CARTESIAN_POINT('Ctrl Pts',(-1.50741159078365,1.,-1.29373841372842));
#33674=CARTESIAN_POINT('Ctrl Pts',(-1.51305994241402,-1.,-1.29596850710509));
#33675=CARTESIAN_POINT('Ctrl Pts',(-1.51305994241402,1.,-1.29596850710509));
#33676=CARTESIAN_POINT('Ctrl Pts',(-1.51872184912724,-1.,-1.29813791800747));
#33677=CARTESIAN_POINT('Ctrl Pts',(-1.51872184912724,1.,-1.29813791800747));
#33678=CARTESIAN_POINT('Ctrl Pts',(-1.52439957861062,-1.,-1.30024984366328));
#33679=CARTESIAN_POINT('Ctrl Pts',(-1.52439957861062,1.,-1.30024984366328));
#33680=CARTESIAN_POINT('Ctrl Pts',(-1.53009970283891,-1.,-1.30231064395568));
#33681=CARTESIAN_POINT('Ctrl Pts',(-1.53009970283891,1.,-1.30231064395568));
#33682=CARTESIAN_POINT('Ctrl Pts',(-1.53582981268977,-1.,-1.30432735639489));
#33683=CARTESIAN_POINT('Ctrl Pts',(-1.53582981268977,1.,-1.30432735639489));
#33684=CARTESIAN_POINT('Ctrl Pts',(-1.54159462645432,-1.,-1.30630475189556));
#33685=CARTESIAN_POINT('Ctrl Pts',(-1.54159462645432,1.,-1.30630475189556));
#33686=CARTESIAN_POINT('Ctrl Pts',(-1.54739413957185,-1.,-1.30824393907473));
#33687=CARTESIAN_POINT('Ctrl Pts',(-1.54739413957185,1.,-1.30824393907473));
#33688=CARTESIAN_POINT('Ctrl Pts',(-1.55322568759481,-1.,-1.31014393684222));
#33689=CARTESIAN_POINT('Ctrl Pts',(-1.55322568759481,1.,-1.31014393684222));
#33690=CARTESIAN_POINT('Ctrl Pts',(-1.55908521254821,-1.,-1.31200264341696));
#33691=CARTESIAN_POINT('Ctrl Pts',(-1.55908521254821,1.,-1.31200264341696));
#33692=CARTESIAN_POINT('Ctrl Pts',(-1.56496872402353,-1.,-1.31381795281002));
#33693=CARTESIAN_POINT('Ctrl Pts',(-1.56496872402353,1.,-1.31381795281002));
#33694=CARTESIAN_POINT('Ctrl Pts',(-1.57087397835723,-1.,-1.31558903860016));
#33695=CARTESIAN_POINT('Ctrl Pts',(-1.57087397835723,1.,-1.31558903860016));
#33696=CARTESIAN_POINT('Ctrl Pts',(-1.5768005650559,-1.,-1.31731642317187));
#33697=CARTESIAN_POINT('Ctrl Pts',(-1.5768005650559,1.,-1.31731642317187));
#33698=CARTESIAN_POINT('Ctrl Pts',(-1.58274907898834,-1.,-1.31900135021432));
#33699=CARTESIAN_POINT('Ctrl Pts',(-1.58274907898834,1.,-1.31900135021432));
#33700=CARTESIAN_POINT('Ctrl Pts',(-1.58872057258245,-1.,-1.32064537110892));
#33701=CARTESIAN_POINT('Ctrl Pts',(-1.58872057258245,1.,-1.32064537110892));
#33702=CARTESIAN_POINT('Ctrl Pts',(-1.59471591079403,-1.,-1.32224985747682));
#33703=CARTESIAN_POINT('Ctrl Pts',(-1.59471591079403,1.,-1.32224985747682));
#33704=CARTESIAN_POINT('Ctrl Pts',(-1.60073511858687,-1.,-1.32381550858256));
#33705=CARTESIAN_POINT('Ctrl Pts',(-1.60073511858687,1.,-1.32381550858256));
#33706=CARTESIAN_POINT('Ctrl Pts',(-1.60677758290954,-1.,-1.32534250785782));
#33707=CARTESIAN_POINT('Ctrl Pts',(-1.60677758290954,1.,-1.32534250785782));
#33708=CARTESIAN_POINT('Ctrl Pts',(-1.6128423401575,-1.,-1.32683074483356));
#33709=CARTESIAN_POINT('Ctrl Pts',(-1.6128423401575,1.,-1.32683074483356));
#33710=CARTESIAN_POINT('Ctrl Pts',(-1.61892832270724,-1.,-1.32828000610449));
#33711=CARTESIAN_POINT('Ctrl Pts',(-1.61892832270724,1.,-1.32828000610449));
#33712=CARTESIAN_POINT('Ctrl Pts',(-1.62503464209797,-1.,-1.3296901950568));
#33713=CARTESIAN_POINT('Ctrl Pts',(-1.62503464209797,1.,-1.3296901950568));
#33714=CARTESIAN_POINT('Ctrl Pts',(-1.63116079730923,-1.,-1.33106149345645));
#33715=CARTESIAN_POINT('Ctrl Pts',(-1.63116079730923,1.,-1.33106149345645));
#33716=CARTESIAN_POINT('Ctrl Pts',(-1.63730653475089,-1.,-1.33239425103724));
#33717=CARTESIAN_POINT('Ctrl Pts',(-1.63730653475089,1.,-1.33239425103724));
#33718=CARTESIAN_POINT('Ctrl Pts',(-1.6434717485603,-1.,-1.33368890676572));
#33719=CARTESIAN_POINT('Ctrl Pts',(-1.6434717485603,1.,-1.33368890676572));
#33720=CARTESIAN_POINT('Ctrl Pts',(-1.6496563728683,-1.,-1.33494590467993));
#33721=CARTESIAN_POINT('Ctrl Pts',(-1.6496563728683,1.,-1.33494590467993));
#33722=CARTESIAN_POINT('Ctrl Pts',(-1.65586025952593,-1.,-1.33616559745172));
#33723=CARTESIAN_POINT('Ctrl Pts',(-1.65586025952593,1.,-1.33616559745172));
#33724=CARTESIAN_POINT('Ctrl Pts',(-1.66208312541983,-1.,-1.33734820885262));
#33725=CARTESIAN_POINT('Ctrl Pts',(-1.66208312541983,1.,-1.33734820885262));
#33726=CARTESIAN_POINT('Ctrl Pts',(-1.66832460783989,-1.,-1.33849388654388));
#33727=CARTESIAN_POINT('Ctrl Pts',(-1.66832460783989,1.,-1.33849388654388));
#33728=CARTESIAN_POINT('Ctrl Pts',(-1.67458429426086,-1.,-1.3396027347034));
#33729=CARTESIAN_POINT('Ctrl Pts',(-1.67458429426086,1.,-1.3396027347034));
#33730=CARTESIAN_POINT('Ctrl Pts',(-1.68086176030362,-1.,-1.34067485185203));
#33731=CARTESIAN_POINT('Ctrl Pts',(-1.68086176030362,1.,-1.34067485185203));
#33732=CARTESIAN_POINT('Ctrl Pts',(-1.68715660868764,-1.,-1.341710374848));
#33733=CARTESIAN_POINT('Ctrl Pts',(-1.68715660868764,1.,-1.341710374848));
#33734=CARTESIAN_POINT('Ctrl Pts',(-1.6934684849687,-1.,-1.34270948206319));
#33735=CARTESIAN_POINT('Ctrl Pts',(-1.6934684849687,1.,-1.34270948206319));
#33736=CARTESIAN_POINT('Ctrl Pts',(-1.69979707754427,-1.,-1.34367237124483));
#33737=CARTESIAN_POINT('Ctrl Pts',(-1.69979707754427,1.,-1.34367237124483));
#33738=CARTESIAN_POINT('Ctrl Pts',(-1.70614212266738,-1.,-1.34459924533831));
#33739=CARTESIAN_POINT('Ctrl Pts',(-1.70614212266738,1.,-1.34459924533831));
#33740=CARTESIAN_POINT('Ctrl Pts',(-1.71250340686822,-1.,-1.34549029589416));
#33741=CARTESIAN_POINT('Ctrl Pts',(-1.71250340686822,1.,-1.34549029589416));
#33742=CARTESIAN_POINT('Ctrl Pts',(-1.7188807715049,-1.,-1.34634568653227));
#33743=CARTESIAN_POINT('Ctrl Pts',(-1.7188807715049,1.,-1.34634568653227));
#33744=CARTESIAN_POINT('Ctrl Pts',(-1.72527410680674,-1.,-1.34716554819527));
#33745=CARTESIAN_POINT('Ctrl Pts',(-1.72527410680674,1.,-1.34716554819527));
#33746=CARTESIAN_POINT('Ctrl Pts',(-1.7304014965394,-1.,-1.34779309152035));
#33747=CARTESIAN_POINT('Ctrl Pts',(-1.7304014965394,1.,-1.34779309152035));
#33748=CARTESIAN_POINT('Ctrl Pts',(-1.73425417885907,-1.,-1.34824783112887));
#33749=CARTESIAN_POINT('Ctrl Pts',(-1.73425417885907,1.,-1.34824783112887));
#33750=CARTESIAN_POINT('Ctrl Pts',(-1.73682580585691,-1.,-1.34854391898045));
#33751=CARTESIAN_POINT('Ctrl Pts',(-1.73682580585691,1.,-1.34854391898045));
#33752=CARTESIAN_POINT('Ctrl Pts',(-1.73811241238545,-1.,-1.34869019493419));
#33753=CARTESIAN_POINT('Ctrl Pts',(-1.73811241238545,1.,-1.34869019493419));
#33754=CARTESIAN_POINT('',(-1.31362392696032,1.,-1.15624053661742));
#33755=CARTESIAN_POINT('Ctrl Pts',(-1.31362392696032,1.,-1.15624053661742));
#33756=CARTESIAN_POINT('Ctrl Pts',(-1.31722977216397,1.,-1.15950888730809));
#33757=CARTESIAN_POINT('Ctrl Pts',(-1.32428080721772,1.,-1.16589330093588));
#33758=CARTESIAN_POINT('Ctrl Pts',(-1.33437539347008,1.,-1.17501305789857));
#33759=CARTESIAN_POINT('Ctrl Pts',(-1.34687054001093,1.,-1.18625865667441));
#33760=CARTESIAN_POINT('Ctrl Pts',(-1.36088705043885,1.,-1.1987959077932));
#33761=CARTESIAN_POINT('Ctrl Pts',(-1.37331915607905,1.,-1.20982812925645));
#33762=CARTESIAN_POINT('Ctrl Pts',(-1.38420564527715,1.,-1.21938737280852));
#33763=CARTESIAN_POINT('Ctrl Pts',(-1.39361389568796,1.,-1.22752961899387));
#33764=CARTESIAN_POINT('Ctrl Pts',(-1.40164708206106,1.,-1.23434087290423));
#33765=CARTESIAN_POINT('Ctrl Pts',(-1.40845295531283,1.,-1.23994455029534));
#33766=CARTESIAN_POINT('Ctrl Pts',(-1.41422913175179,1.,-1.24450600513056));
#33767=CARTESIAN_POINT('Ctrl Pts',(-1.41923722596025,1.,-1.24824430986571));
#33768=CARTESIAN_POINT('Ctrl Pts',(-1.42378102115575,1.,-1.2514145557001));
#33769=CARTESIAN_POINT('Ctrl Pts',(-1.42815938799387,1.,-1.25426945222639));
#33770=CARTESIAN_POINT('Ctrl Pts',(-1.43262645609691,1.,-1.25702687965755));
#33771=CARTESIAN_POINT('Ctrl Pts',(-1.43734919180848,1.,-1.25983531012005));
#33772=CARTESIAN_POINT('Ctrl Pts',(-1.44236470511303,1.,-1.26273903323859));
#33773=CARTESIAN_POINT('Ctrl Pts',(-1.44761985001662,1.,-1.26570925118868));
#33774=CARTESIAN_POINT('Ctrl Pts',(-1.45301422764247,1.,-1.2686778680489));
#33775=CARTESIAN_POINT('Ctrl Pts',(-1.45843906294697,1.,-1.27156805265289));
#33776=CARTESIAN_POINT('Ctrl Pts',(-1.46382431332476,1.,-1.27433119897822));
#33777=CARTESIAN_POINT('Ctrl Pts',(-1.46916035917133,1.,-1.27696414831089));
#33778=CARTESIAN_POINT('Ctrl Pts',(-1.4744717526707,1.,-1.2794891824849));
#33779=CARTESIAN_POINT('Ctrl Pts',(-1.47980070347095,1.,-1.28194158939517));
#33780=CARTESIAN_POINT('Ctrl Pts',(-1.4851881711891,1.,-1.28435533880201));
#33781=CARTESIAN_POINT('Ctrl Pts',(-1.4906522831278,1.,-1.2867467611644));
#33782=CARTESIAN_POINT('Ctrl Pts',(-1.49618896881754,1.,-1.28911506584254));
#33783=CARTESIAN_POINT('Ctrl Pts',(-1.50178230149776,1.,-1.29145022885181));
#33784=CARTESIAN_POINT('Ctrl Pts',(-1.50741159078365,1.,-1.29373841372842));
#33785=CARTESIAN_POINT('Ctrl Pts',(-1.51305994241402,1.,-1.29596850710509));
#33786=CARTESIAN_POINT('Ctrl Pts',(-1.51872184912724,1.,-1.29813791800747));
#33787=CARTESIAN_POINT('Ctrl Pts',(-1.52439957861062,1.,-1.30024984366328));
#33788=CARTESIAN_POINT('Ctrl Pts',(-1.53009970283891,1.,-1.30231064395568));
#33789=CARTESIAN_POINT('Ctrl Pts',(-1.53582981268977,1.,-1.30432735639489));
#33790=CARTESIAN_POINT('Ctrl Pts',(-1.54159462645432,1.,-1.30630475189556));
#33791=CARTESIAN_POINT('Ctrl Pts',(-1.54739413957185,1.,-1.30824393907473));
#33792=CARTESIAN_POINT('Ctrl Pts',(-1.55322568759481,1.,-1.31014393684222));
#33793=CARTESIAN_POINT('Ctrl Pts',(-1.55908521254821,1.,-1.31200264341696));
#33794=CARTESIAN_POINT('Ctrl Pts',(-1.56496872402353,1.,-1.31381795281002));
#33795=CARTESIAN_POINT('Ctrl Pts',(-1.57087397835723,1.,-1.31558903860016));
#33796=CARTESIAN_POINT('Ctrl Pts',(-1.5768005650559,1.,-1.31731642317187));
#33797=CARTESIAN_POINT('Ctrl Pts',(-1.58274907898834,1.,-1.31900135021432));
#33798=CARTESIAN_POINT('Ctrl Pts',(-1.58872057258245,1.,-1.32064537110892));
#33799=CARTESIAN_POINT('Ctrl Pts',(-1.59471591079403,1.,-1.32224985747682));
#33800=CARTESIAN_POINT('Ctrl Pts',(-1.60073511858687,1.,-1.32381550858256));
#33801=CARTESIAN_POINT('Ctrl Pts',(-1.60677758290954,1.,-1.32534250785782));
#33802=CARTESIAN_POINT('Ctrl Pts',(-1.6128423401575,1.,-1.32683074483356));
#33803=CARTESIAN_POINT('Ctrl Pts',(-1.61892832270724,1.,-1.32828000610449));
#33804=CARTESIAN_POINT('Ctrl Pts',(-1.62503464209797,1.,-1.3296901950568));
#33805=CARTESIAN_POINT('Ctrl Pts',(-1.63116079730923,1.,-1.33106149345645));
#33806=CARTESIAN_POINT('Ctrl Pts',(-1.63730653475089,1.,-1.33239425103724));
#33807=CARTESIAN_POINT('Ctrl Pts',(-1.6434717485603,1.,-1.33368890676572));
#33808=CARTESIAN_POINT('Ctrl Pts',(-1.6496563728683,1.,-1.33494590467993));
#33809=CARTESIAN_POINT('Ctrl Pts',(-1.65586025952593,1.,-1.33616559745172));
#33810=CARTESIAN_POINT('Ctrl Pts',(-1.66208312541983,1.,-1.33734820885262));
#33811=CARTESIAN_POINT('Ctrl Pts',(-1.66832460783989,1.,-1.33849388654388));
#33812=CARTESIAN_POINT('Ctrl Pts',(-1.67458429426086,1.,-1.3396027347034));
#33813=CARTESIAN_POINT('Ctrl Pts',(-1.68086176030362,1.,-1.34067485185203));
#33814=CARTESIAN_POINT('Ctrl Pts',(-1.68715660868764,1.,-1.341710374848));
#33815=CARTESIAN_POINT('Ctrl Pts',(-1.6934684849687,1.,-1.34270948206319));
#33816=CARTESIAN_POINT('Ctrl Pts',(-1.69979707754427,1.,-1.34367237124483));
#33817=CARTESIAN_POINT('Ctrl Pts',(-1.70614212266738,1.,-1.34459924533831));
#33818=CARTESIAN_POINT('Ctrl Pts',(-1.71250340686822,1.,-1.34549029589416));
#33819=CARTESIAN_POINT('Ctrl Pts',(-1.7188807715049,1.,-1.34634568653227));
#33820=CARTESIAN_POINT('Ctrl Pts',(-1.72527410680674,1.,-1.34716554819527));
#33821=CARTESIAN_POINT('Ctrl Pts',(-1.7304014965394,1.,-1.34779309152035));
#33822=CARTESIAN_POINT('Ctrl Pts',(-1.73425417885907,1.,-1.34824783112887));
#33823=CARTESIAN_POINT('Ctrl Pts',(-1.73682580585691,1.,-1.34854391898045));
#33824=CARTESIAN_POINT('Ctrl Pts',(-1.73811241238545,1.,-1.34869019493419));
#33825=CARTESIAN_POINT('',(-1.31362392696032,0.,-1.15624053661742));
#33826=CARTESIAN_POINT('Origin',(0.,0.,0.));
#33827=CARTESIAN_POINT('',(-1.15624053661742,1.,-1.31362392696033));
#33828=CARTESIAN_POINT('Origin',(0.,1.,0.));
#33829=CARTESIAN_POINT('',(-1.15624053661742,0.,-1.31362392696033));
#33830=CARTESIAN_POINT('Ctrl Pts',(-1.34869019493419,-1.,-1.73811241238545));
#33831=CARTESIAN_POINT('Ctrl Pts',(-1.34869019493419,1.,-1.73811241238545));
#33832=CARTESIAN_POINT('Ctrl Pts',(-1.34854391898145,-1.,-1.73682580585819));
#33833=CARTESIAN_POINT('Ctrl Pts',(-1.34854391898145,1.,-1.73682580585819));
#33834=CARTESIAN_POINT('Ctrl Pts',(-1.34824783113158,-1.,-1.73425417886255));
#33835=CARTESIAN_POINT('Ctrl Pts',(-1.34824783113158,1.,-1.73425417886255));
#33836=CARTESIAN_POINT('Ctrl Pts',(-1.3477930915247,-1.,-1.73040149654497));
#33837=CARTESIAN_POINT('Ctrl Pts',(-1.3477930915247,1.,-1.73040149654497));
#33838=CARTESIAN_POINT('Ctrl Pts',(-1.34716554820013,-1.,-1.72527410681298));
#33839=CARTESIAN_POINT('Ctrl Pts',(-1.34716554820013,1.,-1.72527410681298));
#33840=CARTESIAN_POINT('Ctrl Pts',(-1.34634568653586,-1.,-1.7188807715095));
#33841=CARTESIAN_POINT('Ctrl Pts',(-1.34634568653586,1.,-1.7188807715095));
#33842=CARTESIAN_POINT('Ctrl Pts',(-1.34549029589563,-1.,-1.71250340687011));
#33843=CARTESIAN_POINT('Ctrl Pts',(-1.34549029589563,1.,-1.71250340687011));
#33844=CARTESIAN_POINT('Ctrl Pts',(-1.34459924533783,-1.,-1.70614212266676));
#33845=CARTESIAN_POINT('Ctrl Pts',(-1.34459924533783,1.,-1.70614212266676));
#33846=CARTESIAN_POINT('Ctrl Pts',(-1.34367237124322,-1.,-1.69979707754221));
#33847=CARTESIAN_POINT('Ctrl Pts',(-1.34367237124322,1.,-1.69979707754221));
#33848=CARTESIAN_POINT('Ctrl Pts',(-1.34270948206139,-1.,-1.6934684849664));
#33849=CARTESIAN_POINT('Ctrl Pts',(-1.34270948206139,1.,-1.6934684849664));
#33850=CARTESIAN_POINT('Ctrl Pts',(-1.34171037484673,-1.,-1.68715660868602));
#33851=CARTESIAN_POINT('Ctrl Pts',(-1.34171037484673,1.,-1.68715660868602));
#33852=CARTESIAN_POINT('Ctrl Pts',(-1.3406748518516,-1.,-1.68086176030308));
#33853=CARTESIAN_POINT('Ctrl Pts',(-1.3406748518516,1.,-1.68086176030308));
#33854=CARTESIAN_POINT('Ctrl Pts',(-1.33960273470372,-1.,-1.67458429426126));
#33855=CARTESIAN_POINT('Ctrl Pts',(-1.33960273470372,1.,-1.67458429426126));
#33856=CARTESIAN_POINT('Ctrl Pts',(-1.33849388654458,-1.,-1.66832460784078));
#33857=CARTESIAN_POINT('Ctrl Pts',(-1.33849388654458,1.,-1.66832460784078));
#33858=CARTESIAN_POINT('Ctrl Pts',(-1.33734820885331,-1.,-1.66208312542073));
#33859=CARTESIAN_POINT('Ctrl Pts',(-1.33734820885331,1.,-1.66208312542073));
#33860=CARTESIAN_POINT('Ctrl Pts',(-1.33616559745217,-1.,-1.65586025952651));
#33861=CARTESIAN_POINT('Ctrl Pts',(-1.33616559745217,1.,-1.65586025952651));
#33862=CARTESIAN_POINT('Ctrl Pts',(-1.33494590468003,-1.,-1.64965637286843));
#33863=CARTESIAN_POINT('Ctrl Pts',(-1.33494590468003,1.,-1.64965637286843));
#33864=CARTESIAN_POINT('Ctrl Pts',(-1.33368890676554,-1.,-1.64347174856007));
#33865=CARTESIAN_POINT('Ctrl Pts',(-1.33368890676554,1.,-1.64347174856007));
#33866=CARTESIAN_POINT('Ctrl Pts',(-1.33239425103694,-1.,-1.6373065347505));
#33867=CARTESIAN_POINT('Ctrl Pts',(-1.33239425103694,1.,-1.6373065347505));
#33868=CARTESIAN_POINT('Ctrl Pts',(-1.33106149345618,-1.,-1.63116079730887));
#33869=CARTESIAN_POINT('Ctrl Pts',(-1.33106149345618,1.,-1.63116079730887));
#33870=CARTESIAN_POINT('Ctrl Pts',(-1.32969019505665,-1.,-1.62503464209777));
#33871=CARTESIAN_POINT('Ctrl Pts',(-1.32969019505665,1.,-1.62503464209777));
#33872=CARTESIAN_POINT('Ctrl Pts',(-1.32828000610448,-1.,-1.61892832270723));
#33873=CARTESIAN_POINT('Ctrl Pts',(-1.32828000610448,1.,-1.61892832270723));
#33874=CARTESIAN_POINT('Ctrl Pts',(-1.32683074483365,-1.,-1.61284234015762));
#33875=CARTESIAN_POINT('Ctrl Pts',(-1.32683074483365,1.,-1.61284234015762));
#33876=CARTESIAN_POINT('Ctrl Pts',(-1.32534250785794,-1.,-1.6067775829097));
#33877=CARTESIAN_POINT('Ctrl Pts',(-1.32534250785794,1.,-1.6067775829097));
#33878=CARTESIAN_POINT('Ctrl Pts',(-1.32381550858266,-1.,-1.600735118587));
#33879=CARTESIAN_POINT('Ctrl Pts',(-1.32381550858266,1.,-1.600735118587));
#33880=CARTESIAN_POINT('Ctrl Pts',(-1.32224985747686,-1.,-1.59471591079408));
#33881=CARTESIAN_POINT('Ctrl Pts',(-1.32224985747686,1.,-1.59471591079408));
#33882=CARTESIAN_POINT('Ctrl Pts',(-1.32064537110891,-1.,-1.58872057258244));
#33883=CARTESIAN_POINT('Ctrl Pts',(-1.32064537110891,1.,-1.58872057258244));
#33884=CARTESIAN_POINT('Ctrl Pts',(-1.31900135021428,-1.,-1.58274907898829));
#33885=CARTESIAN_POINT('Ctrl Pts',(-1.31900135021428,1.,-1.58274907898829));
#33886=CARTESIAN_POINT('Ctrl Pts',(-1.31731642317183,-1.,-1.57680056505585));
#33887=CARTESIAN_POINT('Ctrl Pts',(-1.31731642317183,1.,-1.57680056505585));
#33888=CARTESIAN_POINT('Ctrl Pts',(-1.31558903860015,-1.,-1.57087397835721));
#33889=CARTESIAN_POINT('Ctrl Pts',(-1.31558903860015,1.,-1.57087397835721));
#33890=CARTESIAN_POINT('Ctrl Pts',(-1.31381795281002,-1.,-1.56496872402352));
#33891=CARTESIAN_POINT('Ctrl Pts',(-1.31381795281002,1.,-1.56496872402352));
#33892=CARTESIAN_POINT('Ctrl Pts',(-1.31200264341696,-1.,-1.55908521254822));
#33893=CARTESIAN_POINT('Ctrl Pts',(-1.31200264341696,1.,-1.55908521254822));
#33894=CARTESIAN_POINT('Ctrl Pts',(-1.31014393684221,-1.,-1.55322568759481));
#33895=CARTESIAN_POINT('Ctrl Pts',(-1.31014393684221,1.,-1.55322568759481));
#33896=CARTESIAN_POINT('Ctrl Pts',(-1.30824393907471,-1.,-1.54739413957183));
#33897=CARTESIAN_POINT('Ctrl Pts',(-1.30824393907471,1.,-1.54739413957183));
#33898=CARTESIAN_POINT('Ctrl Pts',(-1.30630475189553,-1.,-1.54159462645428));
#33899=CARTESIAN_POINT('Ctrl Pts',(-1.30630475189553,1.,-1.54159462645428));
#33900=CARTESIAN_POINT('Ctrl Pts',(-1.30432735639487,-1.,-1.53582981268976));
#33901=CARTESIAN_POINT('Ctrl Pts',(-1.30432735639487,1.,-1.53582981268976));
#33902=CARTESIAN_POINT('Ctrl Pts',(-1.3023106439557,-1.,-1.53009970283893));
#33903=CARTESIAN_POINT('Ctrl Pts',(-1.3023106439557,1.,-1.53009970283893));
#33904=CARTESIAN_POINT('Ctrl Pts',(-1.30024984366334,-1.,-1.5243995786107));
#33905=CARTESIAN_POINT('Ctrl Pts',(-1.30024984366334,1.,-1.5243995786107));
#33906=CARTESIAN_POINT('Ctrl Pts',(-1.29813791800757,-1.,-1.51872184912735));
#33907=CARTESIAN_POINT('Ctrl Pts',(-1.29813791800757,1.,-1.51872184912735));
#33908=CARTESIAN_POINT('Ctrl Pts',(-1.29596850710518,-1.,-1.51305994241412));
#33909=CARTESIAN_POINT('Ctrl Pts',(-1.29596850710518,1.,-1.51305994241412));
#33910=CARTESIAN_POINT('Ctrl Pts',(-1.29373841372843,-1.,-1.50741159078367));
#33911=CARTESIAN_POINT('Ctrl Pts',(-1.29373841372843,1.,-1.50741159078367));
#33912=CARTESIAN_POINT('Ctrl Pts',(-1.29145022885171,-1.,-1.50178230149764));
#33913=CARTESIAN_POINT('Ctrl Pts',(-1.29145022885171,1.,-1.50178230149764));
#33914=CARTESIAN_POINT('Ctrl Pts',(-1.28911506584232,-1.,-1.49618896881729));
#33915=CARTESIAN_POINT('Ctrl Pts',(-1.28911506584232,1.,-1.49618896881729));
#33916=CARTESIAN_POINT('Ctrl Pts',(-1.28674676116415,-1.,-1.4906522831275));
#33917=CARTESIAN_POINT('Ctrl Pts',(-1.28674676116415,1.,-1.4906522831275));
#33918=CARTESIAN_POINT('Ctrl Pts',(-1.28435533880184,-1.,-1.48518817118891));
#33919=CARTESIAN_POINT('Ctrl Pts',(-1.28435533880184,1.,-1.48518817118891));
#33920=CARTESIAN_POINT('Ctrl Pts',(-1.28194158939522,-1.,-1.47980070347102));
#33921=CARTESIAN_POINT('Ctrl Pts',(-1.28194158939522,1.,-1.47980070347102));
#33922=CARTESIAN_POINT('Ctrl Pts',(-1.27948918248524,-1.,-1.4744717526711));
#33923=CARTESIAN_POINT('Ctrl Pts',(-1.27948918248524,1.,-1.4744717526711));
#33924=CARTESIAN_POINT('Ctrl Pts',(-1.27696414831144,-1.,-1.46916035917197));
#33925=CARTESIAN_POINT('Ctrl Pts',(-1.27696414831144,1.,-1.46916035917197));
#33926=CARTESIAN_POINT('Ctrl Pts',(-1.27433119897877,-1.,-1.4638243133254));
#33927=CARTESIAN_POINT('Ctrl Pts',(-1.27433119897877,1.,-1.4638243133254));
#33928=CARTESIAN_POINT('Ctrl Pts',(-1.27156805265312,-1.,-1.45843906294725));
#33929=CARTESIAN_POINT('Ctrl Pts',(-1.27156805265312,1.,-1.45843906294725));
#33930=CARTESIAN_POINT('Ctrl Pts',(-1.26867786804854,-1.,-1.45301422764205));
#33931=CARTESIAN_POINT('Ctrl Pts',(-1.26867786804854,1.,-1.45301422764205));
#33932=CARTESIAN_POINT('Ctrl Pts',(-1.26570925118767,-1.,-1.44761985001544));
#33933=CARTESIAN_POINT('Ctrl Pts',(-1.26570925118767,1.,-1.44761985001544));
#33934=CARTESIAN_POINT('Ctrl Pts',(-1.26273903323723,-1.,-1.44236470511145));
#33935=CARTESIAN_POINT('Ctrl Pts',(-1.26273903323723,1.,-1.44236470511145));
#33936=CARTESIAN_POINT('Ctrl Pts',(-1.25983531011894,-1.,-1.43734919180719));
#33937=CARTESIAN_POINT('Ctrl Pts',(-1.25983531011894,1.,-1.43734919180719));
#33938=CARTESIAN_POINT('Ctrl Pts',(-1.25702687965744,-1.,-1.43262645609679));
#33939=CARTESIAN_POINT('Ctrl Pts',(-1.25702687965744,1.,-1.43262645609679));
#33940=CARTESIAN_POINT('Ctrl Pts',(-1.25426945222783,-1.,-1.42815938799555));
#33941=CARTESIAN_POINT('Ctrl Pts',(-1.25426945222783,1.,-1.42815938799555));
#33942=CARTESIAN_POINT('Ctrl Pts',(-1.25141455570299,-1.,-1.42378102115911));
#33943=CARTESIAN_POINT('Ctrl Pts',(-1.25141455570299,1.,-1.42378102115911));
#33944=CARTESIAN_POINT('Ctrl Pts',(-1.24824430986911,-1.,-1.41923722596421));
#33945=CARTESIAN_POINT('Ctrl Pts',(-1.24824430986911,1.,-1.41923722596421));
#33946=CARTESIAN_POINT('Ctrl Pts',(-1.24450600513278,-1.,-1.41422913175437));
#33947=CARTESIAN_POINT('Ctrl Pts',(-1.24450600513278,1.,-1.41422913175437));
#33948=CARTESIAN_POINT('Ctrl Pts',(-1.23994455029421,-1.,-1.40845295531151));
#33949=CARTESIAN_POINT('Ctrl Pts',(-1.23994455029421,1.,-1.40845295531151));
#33950=CARTESIAN_POINT('Ctrl Pts',(-1.23434087289768,-1.,-1.40164708205345));
#33951=CARTESIAN_POINT('Ctrl Pts',(-1.23434087289768,1.,-1.40164708205345));
#33952=CARTESIAN_POINT('Ctrl Pts',(-1.22752961898063,-1.,-1.39361389567257));
#33953=CARTESIAN_POINT('Ctrl Pts',(-1.22752961898063,1.,-1.39361389567257));
#33954=CARTESIAN_POINT('Ctrl Pts',(-1.21938737278853,-1.,-1.38420564525391));
#33955=CARTESIAN_POINT('Ctrl Pts',(-1.21938737278853,1.,-1.38420564525391));
#33956=CARTESIAN_POINT('Ctrl Pts',(-1.20982812923113,-1.,-1.37331915604962));
#33957=CARTESIAN_POINT('Ctrl Pts',(-1.20982812923113,1.,-1.37331915604962));
#33958=CARTESIAN_POINT('Ctrl Pts',(-1.1987959077656,-1.,-1.36088705040677));
#33959=CARTESIAN_POINT('Ctrl Pts',(-1.1987959077656,1.,-1.36088705040677));
#33960=CARTESIAN_POINT('Ctrl Pts',(-1.18625865664915,-1.,-1.34687053998157));
#33961=CARTESIAN_POINT('Ctrl Pts',(-1.18625865664915,1.,-1.34687053998157));
#33962=CARTESIAN_POINT('Ctrl Pts',(-1.17501305787994,-1.,-1.33437539344842));
#33963=CARTESIAN_POINT('Ctrl Pts',(-1.17501305787994,1.,-1.33437539344842));
#33964=CARTESIAN_POINT('Ctrl Pts',(-1.16589330092532,-1.,-1.32428080720544));
#33965=CARTESIAN_POINT('Ctrl Pts',(-1.16589330092532,1.,-1.32428080720544));
#33966=CARTESIAN_POINT('Ctrl Pts',(-1.15950888730433,-1.,-1.3172297721596));
#33967=CARTESIAN_POINT('Ctrl Pts',(-1.15950888730433,1.,-1.3172297721596));
#33968=CARTESIAN_POINT('Ctrl Pts',(-1.15624053661742,-1.,-1.31362392696033));
#33969=CARTESIAN_POINT('Ctrl Pts',(-1.15624053661742,1.,-1.31362392696033));
#33970=CARTESIAN_POINT('',(-1.34869019493419,1.,-1.73811241238545));
#33971=CARTESIAN_POINT('Ctrl Pts',(-1.34869019493419,1.,-1.73811241238545));
#33972=CARTESIAN_POINT('Ctrl Pts',(-1.34854391898145,1.,-1.73682580585819));
#33973=CARTESIAN_POINT('Ctrl Pts',(-1.34824783113158,1.,-1.73425417886255));
#33974=CARTESIAN_POINT('Ctrl Pts',(-1.3477930915247,1.,-1.73040149654497));
#33975=CARTESIAN_POINT('Ctrl Pts',(-1.34716554820013,1.,-1.72527410681298));
#33976=CARTESIAN_POINT('Ctrl Pts',(-1.34634568653586,1.,-1.7188807715095));
#33977=CARTESIAN_POINT('Ctrl Pts',(-1.34549029589563,1.,-1.71250340687011));
#33978=CARTESIAN_POINT('Ctrl Pts',(-1.34459924533783,1.,-1.70614212266676));
#33979=CARTESIAN_POINT('Ctrl Pts',(-1.34367237124322,1.,-1.69979707754221));
#33980=CARTESIAN_POINT('Ctrl Pts',(-1.34270948206139,1.,-1.6934684849664));
#33981=CARTESIAN_POINT('Ctrl Pts',(-1.34171037484673,1.,-1.68715660868602));
#33982=CARTESIAN_POINT('Ctrl Pts',(-1.3406748518516,1.,-1.68086176030308));
#33983=CARTESIAN_POINT('Ctrl Pts',(-1.33960273470372,1.,-1.67458429426126));
#33984=CARTESIAN_POINT('Ctrl Pts',(-1.33849388654458,1.,-1.66832460784078));
#33985=CARTESIAN_POINT('Ctrl Pts',(-1.33734820885331,1.,-1.66208312542073));
#33986=CARTESIAN_POINT('Ctrl Pts',(-1.33616559745217,1.,-1.65586025952651));
#33987=CARTESIAN_POINT('Ctrl Pts',(-1.33494590468003,1.,-1.64965637286843));
#33988=CARTESIAN_POINT('Ctrl Pts',(-1.33368890676554,1.,-1.64347174856007));
#33989=CARTESIAN_POINT('Ctrl Pts',(-1.33239425103694,1.,-1.6373065347505));
#33990=CARTESIAN_POINT('Ctrl Pts',(-1.33106149345618,1.,-1.63116079730887));
#33991=CARTESIAN_POINT('Ctrl Pts',(-1.32969019505665,1.,-1.62503464209777));
#33992=CARTESIAN_POINT('Ctrl Pts',(-1.32828000610448,1.,-1.61892832270723));
#33993=CARTESIAN_POINT('Ctrl Pts',(-1.32683074483365,1.,-1.61284234015762));
#33994=CARTESIAN_POINT('Ctrl Pts',(-1.32534250785794,1.,-1.6067775829097));
#33995=CARTESIAN_POINT('Ctrl Pts',(-1.32381550858266,1.,-1.600735118587));
#33996=CARTESIAN_POINT('Ctrl Pts',(-1.32224985747686,1.,-1.59471591079408));
#33997=CARTESIAN_POINT('Ctrl Pts',(-1.32064537110891,1.,-1.58872057258244));
#33998=CARTESIAN_POINT('Ctrl Pts',(-1.31900135021428,1.,-1.58274907898829));
#33999=CARTESIAN_POINT('Ctrl Pts',(-1.31731642317183,1.,-1.57680056505585));
#34000=CARTESIAN_POINT('Ctrl Pts',(-1.31558903860015,1.,-1.57087397835721));
#34001=CARTESIAN_POINT('Ctrl Pts',(-1.31381795281002,1.,-1.56496872402352));
#34002=CARTESIAN_POINT('Ctrl Pts',(-1.31200264341696,1.,-1.55908521254822));
#34003=CARTESIAN_POINT('Ctrl Pts',(-1.31014393684221,1.,-1.55322568759481));
#34004=CARTESIAN_POINT('Ctrl Pts',(-1.30824393907471,1.,-1.54739413957183));
#34005=CARTESIAN_POINT('Ctrl Pts',(-1.30630475189553,1.,-1.54159462645428));
#34006=CARTESIAN_POINT('Ctrl Pts',(-1.30432735639487,1.,-1.53582981268976));
#34007=CARTESIAN_POINT('Ctrl Pts',(-1.3023106439557,1.,-1.53009970283893));
#34008=CARTESIAN_POINT('Ctrl Pts',(-1.30024984366334,1.,-1.5243995786107));
#34009=CARTESIAN_POINT('Ctrl Pts',(-1.29813791800757,1.,-1.51872184912735));
#34010=CARTESIAN_POINT('Ctrl Pts',(-1.29596850710518,1.,-1.51305994241412));
#34011=CARTESIAN_POINT('Ctrl Pts',(-1.29373841372843,1.,-1.50741159078367));
#34012=CARTESIAN_POINT('Ctrl Pts',(-1.29145022885171,1.,-1.50178230149764));
#34013=CARTESIAN_POINT('Ctrl Pts',(-1.28911506584232,1.,-1.49618896881729));
#34014=CARTESIAN_POINT('Ctrl Pts',(-1.28674676116415,1.,-1.4906522831275));
#34015=CARTESIAN_POINT('Ctrl Pts',(-1.28435533880184,1.,-1.48518817118891));
#34016=CARTESIAN_POINT('Ctrl Pts',(-1.28194158939522,1.,-1.47980070347102));
#34017=CARTESIAN_POINT('Ctrl Pts',(-1.27948918248524,1.,-1.4744717526711));
#34018=CARTESIAN_POINT('Ctrl Pts',(-1.27696414831144,1.,-1.46916035917197));
#34019=CARTESIAN_POINT('Ctrl Pts',(-1.27433119897877,1.,-1.4638243133254));
#34020=CARTESIAN_POINT('Ctrl Pts',(-1.27156805265312,1.,-1.45843906294725));
#34021=CARTESIAN_POINT('Ctrl Pts',(-1.26867786804854,1.,-1.45301422764205));
#34022=CARTESIAN_POINT('Ctrl Pts',(-1.26570925118767,1.,-1.44761985001544));
#34023=CARTESIAN_POINT('Ctrl Pts',(-1.26273903323723,1.,-1.44236470511145));
#34024=CARTESIAN_POINT('Ctrl Pts',(-1.25983531011894,1.,-1.43734919180719));
#34025=CARTESIAN_POINT('Ctrl Pts',(-1.25702687965744,1.,-1.43262645609679));
#34026=CARTESIAN_POINT('Ctrl Pts',(-1.25426945222783,1.,-1.42815938799555));
#34027=CARTESIAN_POINT('Ctrl Pts',(-1.25141455570299,1.,-1.42378102115911));
#34028=CARTESIAN_POINT('Ctrl Pts',(-1.24824430986911,1.,-1.41923722596421));
#34029=CARTESIAN_POINT('Ctrl Pts',(-1.24450600513278,1.,-1.41422913175437));
#34030=CARTESIAN_POINT('Ctrl Pts',(-1.23994455029421,1.,-1.40845295531151));
#34031=CARTESIAN_POINT('Ctrl Pts',(-1.23434087289768,1.,-1.40164708205345));
#34032=CARTESIAN_POINT('Ctrl Pts',(-1.22752961898063,1.,-1.39361389567257));
#34033=CARTESIAN_POINT('Ctrl Pts',(-1.21938737278853,1.,-1.38420564525391));
#34034=CARTESIAN_POINT('Ctrl Pts',(-1.20982812923113,1.,-1.37331915604962));
#34035=CARTESIAN_POINT('Ctrl Pts',(-1.1987959077656,1.,-1.36088705040677));
#34036=CARTESIAN_POINT('Ctrl Pts',(-1.18625865664915,1.,-1.34687053998157));
#34037=CARTESIAN_POINT('Ctrl Pts',(-1.17501305787994,1.,-1.33437539344842));
#34038=CARTESIAN_POINT('Ctrl Pts',(-1.16589330092532,1.,-1.32428080720544));
#34039=CARTESIAN_POINT('Ctrl Pts',(-1.15950888730433,1.,-1.3172297721596));
#34040=CARTESIAN_POINT('Ctrl Pts',(-1.15624053661742,1.,-1.31362392696033));
#34041=CARTESIAN_POINT('',(-1.34869019493419,0.,-1.73811241238545));
#34042=CARTESIAN_POINT('Origin',(-1.23627494547115,0.,-1.81978687191668));
#34043=CARTESIAN_POINT('',(-1.23627494547115,1.,-1.81978687191668));
#34044=CARTESIAN_POINT('',(-1.34869019493419,1.,-1.73811241238545));
#34045=CARTESIAN_POINT('',(-1.23627494547115,0.,-1.81978687191668));
#34046=CARTESIAN_POINT('Ctrl Pts',(-0.892032620296855,-1.,-1.5055822144029));
#34047=CARTESIAN_POINT('Ctrl Pts',(-0.892032620296855,1.,-1.5055822144029));
#34048=CARTESIAN_POINT('Ctrl Pts',(-0.894452006967538,-1.,-1.50980486807181));
#34049=CARTESIAN_POINT('Ctrl Pts',(-0.894452006967538,1.,-1.50980486807181));
#34050=CARTESIAN_POINT('Ctrl Pts',(-0.89918504749193,-1.,-1.51805569591479));
#34051=CARTESIAN_POINT('Ctrl Pts',(-0.89918504749193,1.,-1.51805569591479));
#34052=CARTESIAN_POINT('Ctrl Pts',(-0.905967409640499,-1.,-1.52984849890434));
#34053=CARTESIAN_POINT('Ctrl Pts',(-0.905967409640499,1.,-1.52984849890434));
#34054=CARTESIAN_POINT('Ctrl Pts',(-0.91437591904658,-1.,-1.54440491152808));
#34055=CARTESIAN_POINT('Ctrl Pts',(-0.91437591904658,1.,-1.54440491152808));
#34056=CARTESIAN_POINT('Ctrl Pts',(-0.923832188966322,-1.,-1.56065988582509));
#34057=CARTESIAN_POINT('Ctrl Pts',(-0.923832188966322,1.,-1.56065988582509));
#34058=CARTESIAN_POINT('Ctrl Pts',(-0.932246680128849,-1.,-1.57499388385561));
#34059=CARTESIAN_POINT('Ctrl Pts',(-0.932246680128849,1.,-1.57499388385561));
#34060=CARTESIAN_POINT('Ctrl Pts',(-0.939646377909319,-1.,-1.58744937489796));
#34061=CARTESIAN_POINT('Ctrl Pts',(-0.939646377909319,1.,-1.58744937489796));
#34062=CARTESIAN_POINT('Ctrl Pts',(-0.946078063325796,-1.,-1.59810042045408));
#34063=CARTESIAN_POINT('Ctrl Pts',(-0.946078063325796,1.,-1.59810042045408));
#34064=CARTESIAN_POINT('Ctrl Pts',(-0.951613284361248,-1.,-1.60706069897794));
#34065=CARTESIAN_POINT('Ctrl Pts',(-0.951613284361248,1.,-1.60706069897794));
#34066=CARTESIAN_POINT('Ctrl Pts',(-0.956354422921573,-1.,-1.61449324337233));
#34067=CARTESIAN_POINT('Ctrl Pts',(-0.956354422921573,1.,-1.61449324337233));
#34068=CARTESIAN_POINT('Ctrl Pts',(-0.960438326099958,-1.,-1.62061638139929));
#34069=CARTESIAN_POINT('Ctrl Pts',(-0.960438326099958,1.,-1.62061638139929));
#34070=CARTESIAN_POINT('Ctrl Pts',(-0.964046107037821,-1.,-1.6257193066974));
#34071=CARTESIAN_POINT('Ctrl Pts',(-0.964046107037821,1.,-1.6257193066974));
#34072=CARTESIAN_POINT('Ctrl Pts',(-0.967387853228041,-1.,-1.63013849959083));
#34073=CARTESIAN_POINT('Ctrl Pts',(-0.967387853228041,1.,-1.63013849959083));
#34074=CARTESIAN_POINT('Ctrl Pts',(-0.970669715996356,-1.,-1.63420665729609));
#34075=CARTESIAN_POINT('Ctrl Pts',(-0.970669715996356,1.,-1.63420665729609));
#34076=CARTESIAN_POINT('Ctrl Pts',(-0.974066058287501,-1.,-1.63820952658157));
#34077=CARTESIAN_POINT('Ctrl Pts',(-0.974066058287501,1.,-1.63820952658157));
#34078=CARTESIAN_POINT('Ctrl Pts',(-0.977689794120297,-1.,-1.64233990826831));
#34079=CARTESIAN_POINT('Ctrl Pts',(-0.977689794120297,1.,-1.64233990826831));
#34080=CARTESIAN_POINT('Ctrl Pts',(-0.981562530940574,-1.,-1.64665139190834));
#34081=CARTESIAN_POINT('Ctrl Pts',(-0.981562530940574,1.,-1.64665139190834));
#34082=CARTESIAN_POINT('Ctrl Pts',(-0.985642622921626,-1.,-1.6511001661277));
#34083=CARTESIAN_POINT('Ctrl Pts',(-0.985642622921626,1.,-1.6511001661277));
#34084=CARTESIAN_POINT('Ctrl Pts',(-0.98985562785445,-1.,-1.65559044289746));
#34085=CARTESIAN_POINT('Ctrl Pts',(-0.98985562785445,1.,-1.65559044289746));
#34086=CARTESIAN_POINT('Ctrl Pts',(-0.994121836661116,-1.,-1.66001553809916));
#34087=CARTESIAN_POINT('Ctrl Pts',(-0.994121836661116,1.,-1.66001553809916));
#34088=CARTESIAN_POINT('Ctrl Pts',(-0.998389654952317,-1.,-1.66430758030304));
#34089=CARTESIAN_POINT('Ctrl Pts',(-0.998389654952317,1.,-1.66430758030304));
#34090=CARTESIAN_POINT('Ctrl Pts',(-1.00265091003682,-1.,-1.66846059277231));
#34091=CARTESIAN_POINT('Ctrl Pts',(-1.00265091003682,1.,-1.66846059277231));
#34092=CARTESIAN_POINT('Ctrl Pts',(-1.00692206696387,-1.,-1.67250335383248));
#34093=CARTESIAN_POINT('Ctrl Pts',(-1.00692206696387,1.,-1.67250335383248));
#34094=CARTESIAN_POINT('Ctrl Pts',(-1.01123236493507,-1.,-1.67648246776457));
#34095=CARTESIAN_POINT('Ctrl Pts',(-1.01123236493507,1.,-1.67648246776457));
#34096=CARTESIAN_POINT('Ctrl Pts',(-1.01561026162787,-1.,-1.6804428989482));
#34097=CARTESIAN_POINT('Ctrl Pts',(-1.01561026162787,1.,-1.6804428989482));
#34098=CARTESIAN_POINT('Ctrl Pts',(-1.02006795074222,-1.,-1.68440578021739));
#34099=CARTESIAN_POINT('Ctrl Pts',(-1.02006795074222,1.,-1.68440578021739));
#34100=CARTESIAN_POINT('Ctrl Pts',(-1.02460180535272,-1.,-1.68836910178475));
#34101=CARTESIAN_POINT('Ctrl Pts',(-1.02460180535272,1.,-1.68836910178475));
#34102=CARTESIAN_POINT('Ctrl Pts',(-1.02919977579155,-1.,-1.69231840863471));
#34103=CARTESIAN_POINT('Ctrl Pts',(-1.02919977579155,1.,-1.69231840863471));
#34104=CARTESIAN_POINT('Ctrl Pts',(-1.03384646003587,-1.,-1.69623414782769));
#34105=CARTESIAN_POINT('Ctrl Pts',(-1.03384646003587,1.,-1.69623414782769));
#34106=CARTESIAN_POINT('Ctrl Pts',(-1.03852922490782,-1.,-1.70010052930951));
#34107=CARTESIAN_POINT('Ctrl Pts',(-1.03852922490782,1.,-1.70010052930951));
#34108=CARTESIAN_POINT('Ctrl Pts',(-1.04324363334546,-1.,-1.70391338707969));
#34109=CARTESIAN_POINT('Ctrl Pts',(-1.04324363334546,1.,-1.70391338707969));
#34110=CARTESIAN_POINT('Ctrl Pts',(-1.0479908540499,-1.,-1.70767646263641));
#34111=CARTESIAN_POINT('Ctrl Pts',(-1.0479908540499,1.,-1.70767646263641));
#34112=CARTESIAN_POINT('Ctrl Pts',(-1.05277517202854,-1.,-1.71139783543986));
#34113=CARTESIAN_POINT('Ctrl Pts',(-1.05277517202854,1.,-1.71139783543986));
#34114=CARTESIAN_POINT('Ctrl Pts',(-1.05760163192481,-1.,-1.71508654427022));
#34115=CARTESIAN_POINT('Ctrl Pts',(-1.05760163192481,1.,-1.71508654427022));
#34116=CARTESIAN_POINT('Ctrl Pts',(-1.0624732468065,-1.,-1.71874858456908));
#34117=CARTESIAN_POINT('Ctrl Pts',(-1.0624732468065,1.,-1.71874858456908));
#34118=CARTESIAN_POINT('Ctrl Pts',(-1.06738966975463,-1.,-1.72238500928456));
#34119=CARTESIAN_POINT('Ctrl Pts',(-1.06738966975463,1.,-1.72238500928456));
#34120=CARTESIAN_POINT('Ctrl Pts',(-1.07234866990252,-1.,-1.72599406198489));
#34121=CARTESIAN_POINT('Ctrl Pts',(-1.07234866990252,1.,-1.72599406198489));
#34122=CARTESIAN_POINT('Ctrl Pts',(-1.0773470373727,-1.,-1.72957248977424));
#34123=CARTESIAN_POINT('Ctrl Pts',(-1.0773470373727,1.,-1.72957248977424));
#34124=CARTESIAN_POINT('Ctrl Pts',(-1.08238162784749,-1.,-1.73311705663407));
#34125=CARTESIAN_POINT('Ctrl Pts',(-1.08238162784749,1.,-1.73311705663407));
#34126=CARTESIAN_POINT('Ctrl Pts',(-1.08745056285429,-1.,-1.73662628326093));
#34127=CARTESIAN_POINT('Ctrl Pts',(-1.08745056285429,1.,-1.73662628326093));
#34128=CARTESIAN_POINT('Ctrl Pts',(-1.09255329056496,-1.,-1.74010053962252));
#34129=CARTESIAN_POINT('Ctrl Pts',(-1.09255329056496,1.,-1.74010053962252));
#34130=CARTESIAN_POINT('Ctrl Pts',(-1.09768999241229,-1.,-1.74354119236212));
#34131=CARTESIAN_POINT('Ctrl Pts',(-1.09768999241229,1.,-1.74354119236212));
#34132=CARTESIAN_POINT('Ctrl Pts',(-1.10286118991144,-1.,-1.74695004214924));
#34133=CARTESIAN_POINT('Ctrl Pts',(-1.10286118991144,1.,-1.74695004214924));
#34134=CARTESIAN_POINT('Ctrl Pts',(-1.10806728183003,-1.,-1.75032866075914));
#34135=CARTESIAN_POINT('Ctrl Pts',(-1.10806728183003,1.,-1.75032866075914));
#34136=CARTESIAN_POINT('Ctrl Pts',(-1.11330807582542,-1.,-1.75367772094617));
#34137=CARTESIAN_POINT('Ctrl Pts',(-1.11330807582542,1.,-1.75367772094617));
#34138=CARTESIAN_POINT('Ctrl Pts',(-1.11858293216752,-1.,-1.75699720772089));
#34139=CARTESIAN_POINT('Ctrl Pts',(-1.11858293216752,1.,-1.75699720772089));
#34140=CARTESIAN_POINT('Ctrl Pts',(-1.12389096855078,-1.,-1.76028671825084));
#34141=CARTESIAN_POINT('Ctrl Pts',(-1.12389096855078,1.,-1.76028671825084));
#34142=CARTESIAN_POINT('Ctrl Pts',(-1.12923123555076,-1.,-1.76354571966171));
#34143=CARTESIAN_POINT('Ctrl Pts',(-1.12923123555076,1.,-1.76354571966171));
#34144=CARTESIAN_POINT('Ctrl Pts',(-1.13460291804635,-1.,-1.76677384551883));
#34145=CARTESIAN_POINT('Ctrl Pts',(-1.13460291804635,1.,-1.76677384551883));
#34146=CARTESIAN_POINT('Ctrl Pts',(-1.14000548337,-1.,-1.76997111386806));
#34147=CARTESIAN_POINT('Ctrl Pts',(-1.14000548337,1.,-1.76997111386806));
#34148=CARTESIAN_POINT('Ctrl Pts',(-1.14543858226948,-1.,-1.77313777896234));
#34149=CARTESIAN_POINT('Ctrl Pts',(-1.14543858226948,1.,-1.77313777896234));
#34150=CARTESIAN_POINT('Ctrl Pts',(-1.15090197841531,-1.,-1.77627422557034));
#34151=CARTESIAN_POINT('Ctrl Pts',(-1.15090197841531,1.,-1.77627422557034));
#34152=CARTESIAN_POINT('Ctrl Pts',(-1.15639547194689,-1.,-1.77938085564261));
#34153=CARTESIAN_POINT('Ctrl Pts',(-1.15639547194689,1.,-1.77938085564261));
#34154=CARTESIAN_POINT('Ctrl Pts',(-1.16191881298458,-1.,-1.78245795880949));
#34155=CARTESIAN_POINT('Ctrl Pts',(-1.16191881298458,1.,-1.78245795880949));
#34156=CARTESIAN_POINT('Ctrl Pts',(-1.16747166312239,-1.,-1.78550566040349));
#34157=CARTESIAN_POINT('Ctrl Pts',(-1.16747166312239,1.,-1.78550566040349));
#34158=CARTESIAN_POINT('Ctrl Pts',(-1.17305363177265,-1.,-1.78852398877523));
#34159=CARTESIAN_POINT('Ctrl Pts',(-1.17305363177265,1.,-1.78852398877523));
#34160=CARTESIAN_POINT('Ctrl Pts',(-1.17866429440781,-1.,-1.79151291552646));
#34161=CARTESIAN_POINT('Ctrl Pts',(-1.17866429440781,1.,-1.79151291552646));
#34162=CARTESIAN_POINT('Ctrl Pts',(-1.18430321697471,-1.,-1.79447240321572));
#34163=CARTESIAN_POINT('Ctrl Pts',(-1.18430321697471,1.,-1.79447240321572));
#34164=CARTESIAN_POINT('Ctrl Pts',(-1.1899699793456,-1.,-1.79740245923649));
#34165=CARTESIAN_POINT('Ctrl Pts',(-1.1899699793456,1.,-1.79740245923649));
#34166=CARTESIAN_POINT('Ctrl Pts',(-1.19566418930405,-1.,-1.80030314370121));
#34167=CARTESIAN_POINT('Ctrl Pts',(-1.19566418930405,1.,-1.80030314370121));
#34168=CARTESIAN_POINT('Ctrl Pts',(-1.2013854893912,-1.,-1.8031745483882));
#34169=CARTESIAN_POINT('Ctrl Pts',(-1.2013854893912,1.,-1.8031745483882));
#34170=CARTESIAN_POINT('Ctrl Pts',(-1.20713356605519,-1.,-1.80601678480772));
#34171=CARTESIAN_POINT('Ctrl Pts',(-1.20713356605519,1.,-1.80601678480772));
#34172=CARTESIAN_POINT('Ctrl Pts',(-1.2129081570818,-1.,-1.80882996916931));
#34173=CARTESIAN_POINT('Ctrl Pts',(-1.2129081570818,1.,-1.80882996916931));
#34174=CARTESIAN_POINT('Ctrl Pts',(-1.2187090610323,-1.,-1.81161420806172));
#34175=CARTESIAN_POINT('Ctrl Pts',(-1.2187090610323,1.,-1.81161420806172));
#34176=CARTESIAN_POINT('Ctrl Pts',(-1.22453613304507,-1.,-1.81436959209778));
#34177=CARTESIAN_POINT('Ctrl Pts',(-1.22453613304507,1.,-1.81436959209778));
#34178=CARTESIAN_POINT('Ctrl Pts',(-1.22921864890975,-1.,-1.81655087183054));
#34179=CARTESIAN_POINT('Ctrl Pts',(-1.22921864890975,1.,-1.81655087183054));
#34180=CARTESIAN_POINT('Ctrl Pts',(-1.23274224526804,-1.,-1.81817389920914));
#34181=CARTESIAN_POINT('Ctrl Pts',(-1.23274224526804,1.,-1.81817389920914));
#34182=CARTESIAN_POINT('Ctrl Pts',(-1.23509651170384,-1.,-1.81925017193531));
#34183=CARTESIAN_POINT('Ctrl Pts',(-1.23509651170384,1.,-1.81925017193531));
#34184=CARTESIAN_POINT('Ctrl Pts',(-1.23627494547115,-1.,-1.81978687191668));
#34185=CARTESIAN_POINT('Ctrl Pts',(-1.23627494547115,1.,-1.81978687191668));
#34186=CARTESIAN_POINT('',(-0.892032620296855,1.,-1.5055822144029));
#34187=CARTESIAN_POINT('Ctrl Pts',(-0.892032620296855,1.,-1.5055822144029));
#34188=CARTESIAN_POINT('Ctrl Pts',(-0.894452006967538,1.,-1.50980486807181));
#34189=CARTESIAN_POINT('Ctrl Pts',(-0.89918504749193,1.,-1.51805569591479));
#34190=CARTESIAN_POINT('Ctrl Pts',(-0.905967409640499,1.,-1.52984849890434));
#34191=CARTESIAN_POINT('Ctrl Pts',(-0.91437591904658,1.,-1.54440491152808));
#34192=CARTESIAN_POINT('Ctrl Pts',(-0.923832188966322,1.,-1.56065988582509));
#34193=CARTESIAN_POINT('Ctrl Pts',(-0.932246680128849,1.,-1.57499388385561));
#34194=CARTESIAN_POINT('Ctrl Pts',(-0.939646377909319,1.,-1.58744937489796));
#34195=CARTESIAN_POINT('Ctrl Pts',(-0.946078063325796,1.,-1.59810042045408));
#34196=CARTESIAN_POINT('Ctrl Pts',(-0.951613284361248,1.,-1.60706069897794));
#34197=CARTESIAN_POINT('Ctrl Pts',(-0.956354422921573,1.,-1.61449324337233));
#34198=CARTESIAN_POINT('Ctrl Pts',(-0.960438326099958,1.,-1.62061638139929));
#34199=CARTESIAN_POINT('Ctrl Pts',(-0.964046107037821,1.,-1.6257193066974));
#34200=CARTESIAN_POINT('Ctrl Pts',(-0.967387853228041,1.,-1.63013849959083));
#34201=CARTESIAN_POINT('Ctrl Pts',(-0.970669715996356,1.,-1.63420665729609));
#34202=CARTESIAN_POINT('Ctrl Pts',(-0.974066058287501,1.,-1.63820952658157));
#34203=CARTESIAN_POINT('Ctrl Pts',(-0.977689794120297,1.,-1.64233990826831));
#34204=CARTESIAN_POINT('Ctrl Pts',(-0.981562530940574,1.,-1.64665139190834));
#34205=CARTESIAN_POINT('Ctrl Pts',(-0.985642622921626,1.,-1.6511001661277));
#34206=CARTESIAN_POINT('Ctrl Pts',(-0.98985562785445,1.,-1.65559044289746));
#34207=CARTESIAN_POINT('Ctrl Pts',(-0.994121836661116,1.,-1.66001553809916));
#34208=CARTESIAN_POINT('Ctrl Pts',(-0.998389654952317,1.,-1.66430758030304));
#34209=CARTESIAN_POINT('Ctrl Pts',(-1.00265091003682,1.,-1.66846059277231));
#34210=CARTESIAN_POINT('Ctrl Pts',(-1.00692206696387,1.,-1.67250335383248));
#34211=CARTESIAN_POINT('Ctrl Pts',(-1.01123236493507,1.,-1.67648246776457));
#34212=CARTESIAN_POINT('Ctrl Pts',(-1.01561026162787,1.,-1.6804428989482));
#34213=CARTESIAN_POINT('Ctrl Pts',(-1.02006795074222,1.,-1.68440578021739));
#34214=CARTESIAN_POINT('Ctrl Pts',(-1.02460180535272,1.,-1.68836910178475));
#34215=CARTESIAN_POINT('Ctrl Pts',(-1.02919977579155,1.,-1.69231840863471));
#34216=CARTESIAN_POINT('Ctrl Pts',(-1.03384646003587,1.,-1.69623414782769));
#34217=CARTESIAN_POINT('Ctrl Pts',(-1.03852922490782,1.,-1.70010052930951));
#34218=CARTESIAN_POINT('Ctrl Pts',(-1.04324363334546,1.,-1.70391338707969));
#34219=CARTESIAN_POINT('Ctrl Pts',(-1.0479908540499,1.,-1.70767646263641));
#34220=CARTESIAN_POINT('Ctrl Pts',(-1.05277517202854,1.,-1.71139783543986));
#34221=CARTESIAN_POINT('Ctrl Pts',(-1.05760163192481,1.,-1.71508654427022));
#34222=CARTESIAN_POINT('Ctrl Pts',(-1.0624732468065,1.,-1.71874858456908));
#34223=CARTESIAN_POINT('Ctrl Pts',(-1.06738966975463,1.,-1.72238500928456));
#34224=CARTESIAN_POINT('Ctrl Pts',(-1.07234866990252,1.,-1.72599406198489));
#34225=CARTESIAN_POINT('Ctrl Pts',(-1.0773470373727,1.,-1.72957248977424));
#34226=CARTESIAN_POINT('Ctrl Pts',(-1.08238162784749,1.,-1.73311705663407));
#34227=CARTESIAN_POINT('Ctrl Pts',(-1.08745056285429,1.,-1.73662628326093));
#34228=CARTESIAN_POINT('Ctrl Pts',(-1.09255329056496,1.,-1.74010053962252));
#34229=CARTESIAN_POINT('Ctrl Pts',(-1.09768999241229,1.,-1.74354119236212));
#34230=CARTESIAN_POINT('Ctrl Pts',(-1.10286118991144,1.,-1.74695004214924));
#34231=CARTESIAN_POINT('Ctrl Pts',(-1.10806728183003,1.,-1.75032866075914));
#34232=CARTESIAN_POINT('Ctrl Pts',(-1.11330807582542,1.,-1.75367772094617));
#34233=CARTESIAN_POINT('Ctrl Pts',(-1.11858293216752,1.,-1.75699720772089));
#34234=CARTESIAN_POINT('Ctrl Pts',(-1.12389096855078,1.,-1.76028671825084));
#34235=CARTESIAN_POINT('Ctrl Pts',(-1.12923123555076,1.,-1.76354571966171));
#34236=CARTESIAN_POINT('Ctrl Pts',(-1.13460291804635,1.,-1.76677384551883));
#34237=CARTESIAN_POINT('Ctrl Pts',(-1.14000548337,1.,-1.76997111386806));
#34238=CARTESIAN_POINT('Ctrl Pts',(-1.14543858226948,1.,-1.77313777896234));
#34239=CARTESIAN_POINT('Ctrl Pts',(-1.15090197841531,1.,-1.77627422557034));
#34240=CARTESIAN_POINT('Ctrl Pts',(-1.15639547194689,1.,-1.77938085564261));
#34241=CARTESIAN_POINT('Ctrl Pts',(-1.16191881298458,1.,-1.78245795880949));
#34242=CARTESIAN_POINT('Ctrl Pts',(-1.16747166312239,1.,-1.78550566040349));
#34243=CARTESIAN_POINT('Ctrl Pts',(-1.17305363177265,1.,-1.78852398877523));
#34244=CARTESIAN_POINT('Ctrl Pts',(-1.17866429440781,1.,-1.79151291552646));
#34245=CARTESIAN_POINT('Ctrl Pts',(-1.18430321697471,1.,-1.79447240321572));
#34246=CARTESIAN_POINT('Ctrl Pts',(-1.1899699793456,1.,-1.79740245923649));
#34247=CARTESIAN_POINT('Ctrl Pts',(-1.19566418930405,1.,-1.80030314370121));
#34248=CARTESIAN_POINT('Ctrl Pts',(-1.2013854893912,1.,-1.8031745483882));
#34249=CARTESIAN_POINT('Ctrl Pts',(-1.20713356605519,1.,-1.80601678480772));
#34250=CARTESIAN_POINT('Ctrl Pts',(-1.2129081570818,1.,-1.80882996916931));
#34251=CARTESIAN_POINT('Ctrl Pts',(-1.2187090610323,1.,-1.81161420806172));
#34252=CARTESIAN_POINT('Ctrl Pts',(-1.22453613304507,1.,-1.81436959209778));
#34253=CARTESIAN_POINT('Ctrl Pts',(-1.22921864890975,1.,-1.81655087183054));
#34254=CARTESIAN_POINT('Ctrl Pts',(-1.23274224526804,1.,-1.81817389920914));
#34255=CARTESIAN_POINT('Ctrl Pts',(-1.23509651170384,1.,-1.81925017193531));
#34256=CARTESIAN_POINT('Ctrl Pts',(-1.23627494547115,1.,-1.81978687191668));
#34257=CARTESIAN_POINT('',(-0.892032620296856,0.,-1.5055822144029));
#34258=CARTESIAN_POINT('Origin',(0.,0.,0.));
#34259=CARTESIAN_POINT('',(-0.693717979106305,1.,-1.60662857109684));
#34260=CARTESIAN_POINT('Origin',(0.,1.,0.));
#34261=CARTESIAN_POINT('',(-0.693717979106306,0.,-1.60662857109684));
#34262=CARTESIAN_POINT('Ctrl Pts',(-0.745574324794401,-1.,-2.0698113262342));
#34263=CARTESIAN_POINT('Ctrl Pts',(-0.745574324794401,1.,-2.0698113262342));
#34264=CARTESIAN_POINT('Ctrl Pts',(-0.745832791378367,-1.,-2.06854248895728));
#34265=CARTESIAN_POINT('Ctrl Pts',(-0.745832791378367,1.,-2.06854248895728));
#34266=CARTESIAN_POINT('Ctrl Pts',(-0.7463458715442,-1.,-2.06600523016815));
#34267=CARTESIAN_POINT('Ctrl Pts',(-0.7463458715442,1.,-2.06600523016815));
#34268=CARTESIAN_POINT('Ctrl Pts',(-0.747103932787919,-1.,-2.06220058927826));
#34269=CARTESIAN_POINT('Ctrl Pts',(-0.747103932787919,1.,-2.06220058927826));
#34270=CARTESIAN_POINT('Ctrl Pts',(-0.748091554183802,-1.,-2.05713023031006));
#34271=CARTESIAN_POINT('Ctrl Pts',(-0.748091554183802,1.,-2.05713023031006));
#34272=CARTESIAN_POINT('Ctrl Pts',(-0.749287468665046,-1.,-2.05079645592154));
#34273=CARTESIAN_POINT('Ctrl Pts',(-0.749287468665046,1.,-2.05079645592154));
#34274=CARTESIAN_POINT('Ctrl Pts',(-0.750444657875576,-1.,-2.04446689147979));
#34275=CARTESIAN_POINT('Ctrl Pts',(-0.750444657875576,1.,-2.04446689147979));
#34276=CARTESIAN_POINT('Ctrl Pts',(-0.751562963361115,-1.,-2.03814160092099));
#34277=CARTESIAN_POINT('Ctrl Pts',(-0.751562963361115,1.,-2.03814160092099));
#34278=CARTESIAN_POINT('Ctrl Pts',(-0.752642180487211,-1.,-2.03182068456221));
#34279=CARTESIAN_POINT('Ctrl Pts',(-0.752642180487211,1.,-2.03182068456221));
#34280=CARTESIAN_POINT('Ctrl Pts',(-0.753682061112768,-1.,-2.02550428623313));
#34281=CARTESIAN_POINT('Ctrl Pts',(-0.753682061112768,1.,-2.02550428623313));
#34282=CARTESIAN_POINT('Ctrl Pts',(-0.754682330722816,-1.,-2.01919259405809));
#34283=CARTESIAN_POINT('Ctrl Pts',(-0.754682330722816,1.,-2.01919259405809));
#34284=CARTESIAN_POINT('Ctrl Pts',(-0.755642704957865,-1.,-2.01288584328084));
#34285=CARTESIAN_POINT('Ctrl Pts',(-0.755642704957865,1.,-2.01288584328084));
#34286=CARTESIAN_POINT('Ctrl Pts',(-0.75656290464667,-1.,-2.0065843158773));
#34287=CARTESIAN_POINT('Ctrl Pts',(-0.75656290464667,1.,-2.0065843158773));
#34288=CARTESIAN_POINT('Ctrl Pts',(-0.757442676862724,-1.,-2.00028834739178));
#34289=CARTESIAN_POINT('Ctrl Pts',(-0.757442676862724,1.,-2.00028834739178));
#34290=CARTESIAN_POINT('Ctrl Pts',(-0.758281796766761,-1.,-1.99399831098817));
#34291=CARTESIAN_POINT('Ctrl Pts',(-0.758281796766761,1.,-1.99399831098817));
#34292=CARTESIAN_POINT('Ctrl Pts',(-0.759080037802488,-1.,-1.98771456680874));
#34293=CARTESIAN_POINT('Ctrl Pts',(-0.759080037802488,1.,-1.98771456680874));
#34294=CARTESIAN_POINT('Ctrl Pts',(-0.75983714745219,-1.,-1.98143741418172));
#34295=CARTESIAN_POINT('Ctrl Pts',(-0.75983714745219,1.,-1.98143741418172));
#34296=CARTESIAN_POINT('Ctrl Pts',(-0.760552825409757,-1.,-1.97516705321494));
#34297=CARTESIAN_POINT('Ctrl Pts',(-0.760552825409757,1.,-1.97516705321494));
#34298=CARTESIAN_POINT('Ctrl Pts',(-0.76122669048382,-1.,-1.96890351582499));
#34299=CARTESIAN_POINT('Ctrl Pts',(-0.76122669048382,1.,-1.96890351582499));
#34300=CARTESIAN_POINT('Ctrl Pts',(-0.761858300014423,-1.,-1.96264672744186));
#34301=CARTESIAN_POINT('Ctrl Pts',(-0.761858300014423,1.,-1.96264672744186));
#34302=CARTESIAN_POINT('Ctrl Pts',(-0.762447203806179,-1.,-1.95639665309869));
#34303=CARTESIAN_POINT('Ctrl Pts',(-0.762447203806179,1.,-1.95639665309869));
#34304=CARTESIAN_POINT('Ctrl Pts',(-0.762992990878769,-1.,-1.95015342590024));
#34305=CARTESIAN_POINT('Ctrl Pts',(-0.762992990878769,1.,-1.95015342590024));
#34306=CARTESIAN_POINT('Ctrl Pts',(-0.763495333538629,-1.,-1.9439174661764));
#34307=CARTESIAN_POINT('Ctrl Pts',(-0.763495333538629,1.,-1.9439174661764));
#34308=CARTESIAN_POINT('Ctrl Pts',(-0.763954049121458,-1.,-1.93768964875886));
#34309=CARTESIAN_POINT('Ctrl Pts',(-0.763954049121458,1.,-1.93768964875886));
#34310=CARTESIAN_POINT('Ctrl Pts',(-0.764369010673941,-1.,-1.93147105496382));
#34311=CARTESIAN_POINT('Ctrl Pts',(-0.764369010673941,1.,-1.93147105496382));
#34312=CARTESIAN_POINT('Ctrl Pts',(-0.764740025488211,-1.,-1.92526263537048));
#34313=CARTESIAN_POINT('Ctrl Pts',(-0.764740025488211,1.,-1.92526263537048));
#34314=CARTESIAN_POINT('Ctrl Pts',(-0.765066729667088,-1.,-1.91906491634196));
#34315=CARTESIAN_POINT('Ctrl Pts',(-0.765066729667088,1.,-1.91906491634196));
#34316=CARTESIAN_POINT('Ctrl Pts',(-0.765348465884722,-1.,-1.91287765805169));
#34317=CARTESIAN_POINT('Ctrl Pts',(-0.765348465884722,1.,-1.91287765805169));
#34318=CARTESIAN_POINT('Ctrl Pts',(-0.765584196937919,-1.,-1.90669961402356));
#34319=CARTESIAN_POINT('Ctrl Pts',(-0.765584196937919,1.,-1.90669961402356));
#34320=CARTESIAN_POINT('Ctrl Pts',(-0.765772772593386,-1.,-1.90052930393596));
#34321=CARTESIAN_POINT('Ctrl Pts',(-0.765772772593386,1.,-1.90052930393596));
#34322=CARTESIAN_POINT('Ctrl Pts',(-0.765913193856978,-1.,-1.89436577771388));
#34323=CARTESIAN_POINT('Ctrl Pts',(-0.765913193856978,1.,-1.89436577771388));
#34324=CARTESIAN_POINT('Ctrl Pts',(-0.766004837062091,-1.,-1.88820926433409));
#34325=CARTESIAN_POINT('Ctrl Pts',(-0.766004837062091,1.,-1.88820926433409));
#34326=CARTESIAN_POINT('Ctrl Pts',(-0.766047794851865,-1.,-1.88206215302561));
#34327=CARTESIAN_POINT('Ctrl Pts',(-0.766047794851865,1.,-1.88206215302561));
#34328=CARTESIAN_POINT('Ctrl Pts',(-0.766042837036744,-1.,-1.87592888967883));
#34329=CARTESIAN_POINT('Ctrl Pts',(-0.766042837036744,1.,-1.87592888967883));
#34330=CARTESIAN_POINT('Ctrl Pts',(-0.765990708546091,-1.,-1.86981398314341));
#34331=CARTESIAN_POINT('Ctrl Pts',(-0.765990708546091,1.,-1.86981398314341));
#34332=CARTESIAN_POINT('Ctrl Pts',(-0.765891519092547,-1.,-1.86372027063312));
#34333=CARTESIAN_POINT('Ctrl Pts',(-0.765891519092547,1.,-1.86372027063312));
#34334=CARTESIAN_POINT('Ctrl Pts',(-0.765744212909318,-1.,-1.85764741390394));
#34335=CARTESIAN_POINT('Ctrl Pts',(-0.765744212909318,1.,-1.85764741390394));
#34336=CARTESIAN_POINT('Ctrl Pts',(-0.765545710619062,-1.,-1.85158945130063));
#34337=CARTESIAN_POINT('Ctrl Pts',(-0.765545710619062,1.,-1.85158945130063));
#34338=CARTESIAN_POINT('Ctrl Pts',(-0.765291664862029,-1.,-1.84553698875924));
#34339=CARTESIAN_POINT('Ctrl Pts',(-0.765291664862029,1.,-1.84553698875924));
#34340=CARTESIAN_POINT('Ctrl Pts',(-0.764978057881737,-1.,-1.83948181064835));
#34341=CARTESIAN_POINT('Ctrl Pts',(-0.764978057881737,1.,-1.83948181064835));
#34342=CARTESIAN_POINT('Ctrl Pts',(-0.764602549687853,-1.,-1.83342077227142));
#34343=CARTESIAN_POINT('Ctrl Pts',(-0.764602549687853,1.,-1.83342077227142));
#34344=CARTESIAN_POINT('Ctrl Pts',(-0.764165902605995,-1.,-1.82735991200065));
#34345=CARTESIAN_POINT('Ctrl Pts',(-0.764165902605995,1.,-1.82735991200065));
#34346=CARTESIAN_POINT('Ctrl Pts',(-0.763673465462726,-1.,-1.82131873145266));
#34347=CARTESIAN_POINT('Ctrl Pts',(-0.763673465462726,1.,-1.82131873145266));
#34348=CARTESIAN_POINT('Ctrl Pts',(-0.763132003836634,-1.,-1.8153211840553));
#34349=CARTESIAN_POINT('Ctrl Pts',(-0.763132003836634,1.,-1.8153211840553));
#34350=CARTESIAN_POINT('Ctrl Pts',(-0.762546129463938,-1.,-1.80938551463965));
#34351=CARTESIAN_POINT('Ctrl Pts',(-0.762546129463938,1.,-1.80938551463965));
#34352=CARTESIAN_POINT('Ctrl Pts',(-0.761915336443547,-1.,-1.80351583877342));
#34353=CARTESIAN_POINT('Ctrl Pts',(-0.761915336443547,1.,-1.80351583877342));
#34354=CARTESIAN_POINT('Ctrl Pts',(-0.761229695230558,-1.,-1.79768986997783));
#34355=CARTESIAN_POINT('Ctrl Pts',(-0.761229695230558,1.,-1.79768986997783));
#34356=CARTESIAN_POINT('Ctrl Pts',(-0.760469555880749,-1.,-1.7918581561088));
#34357=CARTESIAN_POINT('Ctrl Pts',(-0.760469555880749,1.,-1.7918581561088));
#34358=CARTESIAN_POINT('Ctrl Pts',(-0.759614401110189,-1.,-1.78596964884604));
#34359=CARTESIAN_POINT('Ctrl Pts',(-0.759614401110189,1.,-1.78596964884604));
#34360=CARTESIAN_POINT('Ctrl Pts',(-0.758650626677518,-1.,-1.77999411220945));
#34361=CARTESIAN_POINT('Ctrl Pts',(-0.758650626677518,1.,-1.77999411220945));
#34362=CARTESIAN_POINT('Ctrl Pts',(-0.757578264077029,-1.,-1.77394167108292));
#34363=CARTESIAN_POINT('Ctrl Pts',(-0.757578264077029,1.,-1.77394167108292));
#34364=CARTESIAN_POINT('Ctrl Pts',(-0.75642189602781,-1.,-1.76789396002998));
#34365=CARTESIAN_POINT('Ctrl Pts',(-0.75642189602781,1.,-1.76789396002998));
#34366=CARTESIAN_POINT('Ctrl Pts',(-0.755220979974461,-1.,-1.76197817240128));
#34367=CARTESIAN_POINT('Ctrl Pts',(-0.755220979974461,1.,-1.76197817240128));
#34368=CARTESIAN_POINT('Ctrl Pts',(-0.754009254027829,-1.,-1.75631083600019));
#34369=CARTESIAN_POINT('Ctrl Pts',(-0.754009254027829,1.,-1.75631083600019));
#34370=CARTESIAN_POINT('Ctrl Pts',(-0.752797683531314,-1.,-1.75095139468794));
#34371=CARTESIAN_POINT('Ctrl Pts',(-0.752797683531314,1.,-1.75095139468794));
#34372=CARTESIAN_POINT('Ctrl Pts',(-0.751555614164482,-1.,-1.74585086852502));
#34373=CARTESIAN_POINT('Ctrl Pts',(-0.751555614164482,1.,-1.74585086852502));
#34374=CARTESIAN_POINT('Ctrl Pts',(-0.750193435981249,-1.,-1.74080458267114));
#34375=CARTESIAN_POINT('Ctrl Pts',(-0.750193435981249,1.,-1.74080458267114));
#34376=CARTESIAN_POINT('Ctrl Pts',(-0.74858246295687,-1.,-1.7355035168033));
#34377=CARTESIAN_POINT('Ctrl Pts',(-0.74858246295687,1.,-1.7355035168033));
#34378=CARTESIAN_POINT('Ctrl Pts',(-0.746574710097752,-1.,-1.72958533647714));
#34379=CARTESIAN_POINT('Ctrl Pts',(-0.746574710097752,1.,-1.72958533647714));
#34380=CARTESIAN_POINT('Ctrl Pts',(-0.744021445433093,-1.,-1.72268229916769));
#34381=CARTESIAN_POINT('Ctrl Pts',(-0.744021445433093,1.,-1.72268229916769));
#34382=CARTESIAN_POINT('Ctrl Pts',(-0.74079516202821,-1.,-1.71447789751001));
#34383=CARTESIAN_POINT('Ctrl Pts',(-0.74079516202821,1.,-1.71447789751001));
#34384=CARTESIAN_POINT('Ctrl Pts',(-0.736799665716932,-1.,-1.70473309004249));
#34385=CARTESIAN_POINT('Ctrl Pts',(-0.736799665716932,1.,-1.70473309004249));
#34386=CARTESIAN_POINT('Ctrl Pts',(-0.731963238685357,-1.,-1.69326921972915));
#34387=CARTESIAN_POINT('Ctrl Pts',(-0.731963238685357,1.,-1.69326921972915));
#34388=CARTESIAN_POINT('Ctrl Pts',(-0.726235967982445,-1.,-1.67996158451922));
#34389=CARTESIAN_POINT('Ctrl Pts',(-0.726235967982445,1.,-1.67996158451922));
#34390=CARTESIAN_POINT('Ctrl Pts',(-0.71958543378795,-1.,-1.66472880551777));
#34391=CARTESIAN_POINT('Ctrl Pts',(-0.71958543378795,1.,-1.66472880551777));
#34392=CARTESIAN_POINT('Ctrl Pts',(-0.711993139340447,-1.,-1.64752408828442));
#34393=CARTESIAN_POINT('Ctrl Pts',(-0.711993139340447,1.,-1.64752408828442));
#34394=CARTESIAN_POINT('Ctrl Pts',(-0.705159151977294,-1.,-1.6321654166204));
#34395=CARTESIAN_POINT('Ctrl Pts',(-0.705159151977294,1.,-1.6321654166204));
#34396=CARTESIAN_POINT('Ctrl Pts',(-0.699605146398837,-1.,-1.61974673471117));
#34397=CARTESIAN_POINT('Ctrl Pts',(-0.699605146398837,1.,-1.61974673471117));
#34398=CARTESIAN_POINT('Ctrl Pts',(-0.69571209787897,-1.,-1.61106790957619));
#34399=CARTESIAN_POINT('Ctrl Pts',(-0.69571209787897,1.,-1.61106790957619));
#34400=CARTESIAN_POINT('Ctrl Pts',(-0.693717979106305,-1.,-1.60662857109684));
#34401=CARTESIAN_POINT('Ctrl Pts',(-0.693717979106305,1.,-1.60662857109684));
#34402=CARTESIAN_POINT('',(-0.745574324794401,1.,-2.0698113262342));
#34403=CARTESIAN_POINT('Ctrl Pts',(-0.745574324794401,1.,-2.0698113262342));
#34404=CARTESIAN_POINT('Ctrl Pts',(-0.745832791378367,1.,-2.06854248895728));
#34405=CARTESIAN_POINT('Ctrl Pts',(-0.7463458715442,1.,-2.06600523016815));
#34406=CARTESIAN_POINT('Ctrl Pts',(-0.747103932787919,1.,-2.06220058927826));
#34407=CARTESIAN_POINT('Ctrl Pts',(-0.748091554183802,1.,-2.05713023031006));
#34408=CARTESIAN_POINT('Ctrl Pts',(-0.749287468665046,1.,-2.05079645592154));
#34409=CARTESIAN_POINT('Ctrl Pts',(-0.750444657875576,1.,-2.04446689147979));
#34410=CARTESIAN_POINT('Ctrl Pts',(-0.751562963361115,1.,-2.03814160092099));
#34411=CARTESIAN_POINT('Ctrl Pts',(-0.752642180487211,1.,-2.03182068456221));
#34412=CARTESIAN_POINT('Ctrl Pts',(-0.753682061112768,1.,-2.02550428623313));
#34413=CARTESIAN_POINT('Ctrl Pts',(-0.754682330722816,1.,-2.01919259405809));
#34414=CARTESIAN_POINT('Ctrl Pts',(-0.755642704957865,1.,-2.01288584328084));
#34415=CARTESIAN_POINT('Ctrl Pts',(-0.75656290464667,1.,-2.0065843158773));
#34416=CARTESIAN_POINT('Ctrl Pts',(-0.757442676862724,1.,-2.00028834739178));
#34417=CARTESIAN_POINT('Ctrl Pts',(-0.758281796766761,1.,-1.99399831098817));
#34418=CARTESIAN_POINT('Ctrl Pts',(-0.759080037802488,1.,-1.98771456680874));
#34419=CARTESIAN_POINT('Ctrl Pts',(-0.75983714745219,1.,-1.98143741418172));
#34420=CARTESIAN_POINT('Ctrl Pts',(-0.760552825409757,1.,-1.97516705321494));
#34421=CARTESIAN_POINT('Ctrl Pts',(-0.76122669048382,1.,-1.96890351582499));
#34422=CARTESIAN_POINT('Ctrl Pts',(-0.761858300014423,1.,-1.96264672744186));
#34423=CARTESIAN_POINT('Ctrl Pts',(-0.762447203806179,1.,-1.95639665309869));
#34424=CARTESIAN_POINT('Ctrl Pts',(-0.762992990878769,1.,-1.95015342590024));
#34425=CARTESIAN_POINT('Ctrl Pts',(-0.763495333538629,1.,-1.9439174661764));
#34426=CARTESIAN_POINT('Ctrl Pts',(-0.763954049121458,1.,-1.93768964875886));
#34427=CARTESIAN_POINT('Ctrl Pts',(-0.764369010673941,1.,-1.93147105496382));
#34428=CARTESIAN_POINT('Ctrl Pts',(-0.764740025488211,1.,-1.92526263537048));
#34429=CARTESIAN_POINT('Ctrl Pts',(-0.765066729667088,1.,-1.91906491634196));
#34430=CARTESIAN_POINT('Ctrl Pts',(-0.765348465884722,1.,-1.91287765805169));
#34431=CARTESIAN_POINT('Ctrl Pts',(-0.765584196937919,1.,-1.90669961402356));
#34432=CARTESIAN_POINT('Ctrl Pts',(-0.765772772593386,1.,-1.90052930393596));
#34433=CARTESIAN_POINT('Ctrl Pts',(-0.765913193856978,1.,-1.89436577771388));
#34434=CARTESIAN_POINT('Ctrl Pts',(-0.766004837062091,1.,-1.88820926433409));
#34435=CARTESIAN_POINT('Ctrl Pts',(-0.766047794851865,1.,-1.88206215302561));
#34436=CARTESIAN_POINT('Ctrl Pts',(-0.766042837036744,1.,-1.87592888967883));
#34437=CARTESIAN_POINT('Ctrl Pts',(-0.765990708546091,1.,-1.86981398314341));
#34438=CARTESIAN_POINT('Ctrl Pts',(-0.765891519092547,1.,-1.86372027063312));
#34439=CARTESIAN_POINT('Ctrl Pts',(-0.765744212909318,1.,-1.85764741390394));
#34440=CARTESIAN_POINT('Ctrl Pts',(-0.765545710619062,1.,-1.85158945130063));
#34441=CARTESIAN_POINT('Ctrl Pts',(-0.765291664862029,1.,-1.84553698875924));
#34442=CARTESIAN_POINT('Ctrl Pts',(-0.764978057881737,1.,-1.83948181064835));
#34443=CARTESIAN_POINT('Ctrl Pts',(-0.764602549687853,1.,-1.83342077227142));
#34444=CARTESIAN_POINT('Ctrl Pts',(-0.764165902605995,1.,-1.82735991200065));
#34445=CARTESIAN_POINT('Ctrl Pts',(-0.763673465462726,1.,-1.82131873145266));
#34446=CARTESIAN_POINT('Ctrl Pts',(-0.763132003836634,1.,-1.8153211840553));
#34447=CARTESIAN_POINT('Ctrl Pts',(-0.762546129463938,1.,-1.80938551463965));
#34448=CARTESIAN_POINT('Ctrl Pts',(-0.761915336443547,1.,-1.80351583877342));
#34449=CARTESIAN_POINT('Ctrl Pts',(-0.761229695230558,1.,-1.79768986997783));
#34450=CARTESIAN_POINT('Ctrl Pts',(-0.760469555880749,1.,-1.7918581561088));
#34451=CARTESIAN_POINT('Ctrl Pts',(-0.759614401110189,1.,-1.78596964884604));
#34452=CARTESIAN_POINT('Ctrl Pts',(-0.758650626677518,1.,-1.77999411220945));
#34453=CARTESIAN_POINT('Ctrl Pts',(-0.757578264077029,1.,-1.77394167108292));
#34454=CARTESIAN_POINT('Ctrl Pts',(-0.75642189602781,1.,-1.76789396002998));
#34455=CARTESIAN_POINT('Ctrl Pts',(-0.755220979974461,1.,-1.76197817240128));
#34456=CARTESIAN_POINT('Ctrl Pts',(-0.754009254027829,1.,-1.75631083600019));
#34457=CARTESIAN_POINT('Ctrl Pts',(-0.752797683531314,1.,-1.75095139468794));
#34458=CARTESIAN_POINT('Ctrl Pts',(-0.751555614164482,1.,-1.74585086852502));
#34459=CARTESIAN_POINT('Ctrl Pts',(-0.750193435981249,1.,-1.74080458267114));
#34460=CARTESIAN_POINT('Ctrl Pts',(-0.74858246295687,1.,-1.7355035168033));
#34461=CARTESIAN_POINT('Ctrl Pts',(-0.746574710097752,1.,-1.72958533647714));
#34462=CARTESIAN_POINT('Ctrl Pts',(-0.744021445433093,1.,-1.72268229916769));
#34463=CARTESIAN_POINT('Ctrl Pts',(-0.74079516202821,1.,-1.71447789751001));
#34464=CARTESIAN_POINT('Ctrl Pts',(-0.736799665716932,1.,-1.70473309004249));
#34465=CARTESIAN_POINT('Ctrl Pts',(-0.731963238685357,1.,-1.69326921972915));
#34466=CARTESIAN_POINT('Ctrl Pts',(-0.726235967982445,1.,-1.67996158451922));
#34467=CARTESIAN_POINT('Ctrl Pts',(-0.71958543378795,1.,-1.66472880551777));
#34468=CARTESIAN_POINT('Ctrl Pts',(-0.711993139340447,1.,-1.64752408828442));
#34469=CARTESIAN_POINT('Ctrl Pts',(-0.705159151977294,1.,-1.6321654166204));
#34470=CARTESIAN_POINT('Ctrl Pts',(-0.699605146398837,1.,-1.61974673471117));
#34471=CARTESIAN_POINT('Ctrl Pts',(-0.69571209787897,1.,-1.61106790957619));
#34472=CARTESIAN_POINT('Ctrl Pts',(-0.693717979106305,1.,-1.60662857109684));
#34473=CARTESIAN_POINT('',(-0.745574324794401,0.,-2.0698113262342));
#34474=CARTESIAN_POINT('Origin',(-0.61342227326009,0.,-2.11275013067528));
#34475=CARTESIAN_POINT('',(-0.61342227326009,1.,-2.11275013067528));
#34476=CARTESIAN_POINT('',(-0.745574324794401,1.,-2.0698113262342));
#34477=CARTESIAN_POINT('',(-0.61342227326009,0.,-2.11275013067528));
#34478=CARTESIAN_POINT('Ctrl Pts',(-0.383122945602004,-1.,-1.7075470150345));
#34479=CARTESIAN_POINT('Ctrl Pts',(-0.383122945602004,1.,-1.7075470150345));
#34480=CARTESIAN_POINT('Ctrl Pts',(-0.384119047315542,-1.,-1.71231062891958));
#34481=CARTESIAN_POINT('Ctrl Pts',(-0.384119047315542,1.,-1.71231062891958));
#34482=CARTESIAN_POINT('Ctrl Pts',(-0.38607079032701,-1.,-1.72162022246158));
#34483=CARTESIAN_POINT('Ctrl Pts',(-0.38607079032701,1.,-1.72162022246158));
#34484=CARTESIAN_POINT('Ctrl Pts',(-0.388877023509191,-1.,-1.7349317097561));
#34485=CARTESIAN_POINT('Ctrl Pts',(-0.388877023509191,1.,-1.7349317097561));
#34486=CARTESIAN_POINT('Ctrl Pts',(-0.392375812294307,-1.,-1.75137405313962));
#34487=CARTESIAN_POINT('Ctrl Pts',(-0.392375812294307,1.,-1.75137405313962));
#34488=CARTESIAN_POINT('Ctrl Pts',(-0.39634619612042,-1.,-1.7697556004756));
#34489=CARTESIAN_POINT('Ctrl Pts',(-0.39634619612042,1.,-1.7697556004756));
#34490=CARTESIAN_POINT('Ctrl Pts',(-0.39991940378308,-1.,-1.78598826347533));
#34491=CARTESIAN_POINT('Ctrl Pts',(-0.39991940378308,1.,-1.78598826347533));
#34492=CARTESIAN_POINT('Ctrl Pts',(-0.403107976170441,-1.,-1.80012077176221));
#34493=CARTESIAN_POINT('Ctrl Pts',(-0.403107976170441,1.,-1.80012077176221));
#34494=CARTESIAN_POINT('Ctrl Pts',(-0.405933518411838,-1.,-1.81223801813988));
#34495=CARTESIAN_POINT('Ctrl Pts',(-0.405933518411838,1.,-1.81223801813988));
#34496=CARTESIAN_POINT('Ctrl Pts',(-0.408428948108533,-1.,-1.8224702267854));
#34497=CARTESIAN_POINT('Ctrl Pts',(-0.408428948108533,1.,-1.8224702267854));
#34498=CARTESIAN_POINT('Ctrl Pts',(-0.410641256301675,-1.,-1.83100408895216));
#34499=CARTESIAN_POINT('Ctrl Pts',(-0.410641256301675,1.,-1.83100408895216));
#34500=CARTESIAN_POINT('Ctrl Pts',(-0.412633125322162,-1.,-1.83808953475839));
#34501=CARTESIAN_POINT('Ctrl Pts',(-0.412633125322162,1.,-1.83808953475839));
#34502=CARTESIAN_POINT('Ctrl Pts',(-0.41448743825434,-1.,-1.8440575707371));
#34503=CARTESIAN_POINT('Ctrl Pts',(-0.41448743825434,1.,-1.8440575707371));
#34504=CARTESIAN_POINT('Ctrl Pts',(-0.416300022038864,-1.,-1.84929312929882));
#34505=CARTESIAN_POINT('Ctrl Pts',(-0.416300022038864,1.,-1.84929312929882));
#34506=CARTESIAN_POINT('Ctrl Pts',(-0.418164129143534,-1.,-1.85417632856234));
#34507=CARTESIAN_POINT('Ctrl Pts',(-0.418164129143534,1.,-1.85417632856234));
#34508=CARTESIAN_POINT('Ctrl Pts',(-0.420157287975619,-1.,-1.85903281096686));
#34509=CARTESIAN_POINT('Ctrl Pts',(-0.420157287975619,1.,-1.85903281096686));
#34510=CARTESIAN_POINT('Ctrl Pts',(-0.422327307418275,-1.,-1.86408083334028));
#34511=CARTESIAN_POINT('Ctrl Pts',(-0.422327307418275,1.,-1.86408083334028));
#34512=CARTESIAN_POINT('Ctrl Pts',(-0.424678177291359,-1.,-1.86937803944323));
#34513=CARTESIAN_POINT('Ctrl Pts',(-0.424678177291359,1.,-1.86937803944323));
#34514=CARTESIAN_POINT('Ctrl Pts',(-0.427183828519102,-1.,-1.87486989291484));
#34515=CARTESIAN_POINT('Ctrl Pts',(-0.427183828519102,1.,-1.87486989291484));
#34516=CARTESIAN_POINT('Ctrl Pts',(-0.429803062482344,-1.,-1.88044229001832));
#34517=CARTESIAN_POINT('Ctrl Pts',(-0.429803062482344,1.,-1.88044229001832));
#34518=CARTESIAN_POINT('Ctrl Pts',(-0.432493038548748,-1.,-1.88596913666793));
#34519=CARTESIAN_POINT('Ctrl Pts',(-0.432493038548748,1.,-1.88596913666793));
#34520=CARTESIAN_POINT('Ctrl Pts',(-0.435225660963383,-1.,-1.89136993975504));
#34521=CARTESIAN_POINT('Ctrl Pts',(-0.435225660963383,1.,-1.89136993975504));
#34522=CARTESIAN_POINT('Ctrl Pts',(-0.437995003948244,-1.,-1.89663648956466));
#34523=CARTESIAN_POINT('Ctrl Pts',(-0.437995003948244,1.,-1.89663648956466));
#34524=CARTESIAN_POINT('Ctrl Pts',(-0.440807833704038,-1.,-1.90180124389086));
#34525=CARTESIAN_POINT('Ctrl Pts',(-0.440807833704038,1.,-1.90180124389086));
#34526=CARTESIAN_POINT('Ctrl Pts',(-0.443677556849151,-1.,-1.90691756144898));
#34527=CARTESIAN_POINT('Ctrl Pts',(-0.443677556849151,1.,-1.90691756144898));
#34528=CARTESIAN_POINT('Ctrl Pts',(-0.446617343485711,-1.,-1.9120369998112));
#34529=CARTESIAN_POINT('Ctrl Pts',(-0.446617343485711,1.,-1.9120369998112));
#34530=CARTESIAN_POINT('Ctrl Pts',(-0.449632260106662,-1.,-1.91718342555755));
#34531=CARTESIAN_POINT('Ctrl Pts',(-0.449632260106662,1.,-1.91718342555755));
#34532=CARTESIAN_POINT('Ctrl Pts',(-0.452719478359432,-1.,-1.92235380648502));
#34533=CARTESIAN_POINT('Ctrl Pts',(-0.452719478359432,1.,-1.92235380648502));
#34534=CARTESIAN_POINT('Ctrl Pts',(-0.455872005174371,-1.,-1.92753067150476));
#34535=CARTESIAN_POINT('Ctrl Pts',(-0.455872005174371,1.,-1.92753067150476));
#34536=CARTESIAN_POINT('Ctrl Pts',(-0.459081234547926,-1.,-1.93269066517934));
#34537=CARTESIAN_POINT('Ctrl Pts',(-0.459081234547926,1.,-1.93269066517934));
#34538=CARTESIAN_POINT('Ctrl Pts',(-0.462340031009056,-1.,-1.93781486640821));
#34539=CARTESIAN_POINT('Ctrl Pts',(-0.462340031009056,1.,-1.93781486640821));
#34540=CARTESIAN_POINT('Ctrl Pts',(-0.46564546202603,-1.,-1.9428979419619));
#34541=CARTESIAN_POINT('Ctrl Pts',(-0.46564546202603,1.,-1.9428979419619));
#34542=CARTESIAN_POINT('Ctrl Pts',(-0.468997482913135,-1.,-1.94794381136514));
#34543=CARTESIAN_POINT('Ctrl Pts',(-0.468997482913135,1.,-1.94794381136514));
#34544=CARTESIAN_POINT('Ctrl Pts',(-0.472397672264072,-1.,-1.95296148278133));
#34545=CARTESIAN_POINT('Ctrl Pts',(-0.472397672264072,1.,-1.95296148278133));
#34546=CARTESIAN_POINT('Ctrl Pts',(-0.475848034683176,-1.,-1.95796111148177));
#34547=CARTESIAN_POINT('Ctrl Pts',(-0.475848034683176,1.,-1.95796111148177));
#34548=CARTESIAN_POINT('Ctrl Pts',(-0.479349583074855,-1.,-1.96294933055943));
#34549=CARTESIAN_POINT('Ctrl Pts',(-0.479349583074855,1.,-1.96294933055943));
#34550=CARTESIAN_POINT('Ctrl Pts',(-0.482901662120691,-1.,-1.96792703422362));
#34551=CARTESIAN_POINT('Ctrl Pts',(-0.482901662120691,1.,-1.96792703422362));
#34552=CARTESIAN_POINT('Ctrl Pts',(-0.486502692907659,-1.,-1.97289186263272));
#34553=CARTESIAN_POINT('Ctrl Pts',(-0.486502692907659,1.,-1.97289186263272));
#34554=CARTESIAN_POINT('Ctrl Pts',(-0.490150627860952,-1.,-1.97783973019229));
#34555=CARTESIAN_POINT('Ctrl Pts',(-0.490150627860952,1.,-1.97783973019229));
#34556=CARTESIAN_POINT('Ctrl Pts',(-0.493843476541495,-1.,-1.98276658761821));
#34557=CARTESIAN_POINT('Ctrl Pts',(-0.493843476541495,1.,-1.98276658761821));
#34558=CARTESIAN_POINT('Ctrl Pts',(-0.497579909545574,-1.,-1.98767044752932));
#34559=CARTESIAN_POINT('Ctrl Pts',(-0.497579909545574,1.,-1.98767044752932));
#34560=CARTESIAN_POINT('Ctrl Pts',(-0.501359287727146,-1.,-1.99255149126155));
#34561=CARTESIAN_POINT('Ctrl Pts',(-0.501359287727146,1.,-1.99255149126155));
#34562=CARTESIAN_POINT('Ctrl Pts',(-0.505181361323026,-1.,-1.99741107463572));
#34563=CARTESIAN_POINT('Ctrl Pts',(-0.505181361323026,1.,-1.99741107463572));
#34564=CARTESIAN_POINT('Ctrl Pts',(-0.509046069886157,-1.,-2.00225107134734));
#34565=CARTESIAN_POINT('Ctrl Pts',(-0.509046069886157,1.,-2.00225107134734));
#34566=CARTESIAN_POINT('Ctrl Pts',(-0.512953306961792,-1.,-2.00707309946949));
#34567=CARTESIAN_POINT('Ctrl Pts',(-0.512953306961792,1.,-2.00707309946949));
#34568=CARTESIAN_POINT('Ctrl Pts',(-0.516902681728687,-1.,-2.01187773939242));
#34569=CARTESIAN_POINT('Ctrl Pts',(-0.516902681728687,1.,-2.01187773939242));
#34570=CARTESIAN_POINT('Ctrl Pts',(-0.52089359039937,-1.,-2.01666477917286));
#34571=CARTESIAN_POINT('Ctrl Pts',(-0.52089359039937,1.,-2.01666477917286));
#34572=CARTESIAN_POINT('Ctrl Pts',(-0.524925318333476,-1.,-2.02143356304698));
#34573=CARTESIAN_POINT('Ctrl Pts',(-0.524925318333476,1.,-2.02143356304698));
#34574=CARTESIAN_POINT('Ctrl Pts',(-0.528997127241914,-1.,-2.0261832908329));
#34575=CARTESIAN_POINT('Ctrl Pts',(-0.528997127241914,1.,-2.0261832908329));
#34576=CARTESIAN_POINT('Ctrl Pts',(-0.533108355132977,-1.,-2.03091336214426));
#34577=CARTESIAN_POINT('Ctrl Pts',(-0.533108355132977,1.,-2.03091336214426));
#34578=CARTESIAN_POINT('Ctrl Pts',(-0.537258489833262,-1.,-2.03562362954037));
#34579=CARTESIAN_POINT('Ctrl Pts',(-0.537258489833262,1.,-2.03562362954037));
#34580=CARTESIAN_POINT('Ctrl Pts',(-0.541447120615659,-1.,-2.04031422690527));
#34581=CARTESIAN_POINT('Ctrl Pts',(-0.541447120615659,1.,-2.04031422690527));
#34582=CARTESIAN_POINT('Ctrl Pts',(-0.54567390381743,-1.,-2.04498544714588));
#34583=CARTESIAN_POINT('Ctrl Pts',(-0.54567390381743,1.,-2.04498544714588));
#34584=CARTESIAN_POINT('Ctrl Pts',(-0.549938525150295,-1.,-2.04963761077958));
#34585=CARTESIAN_POINT('Ctrl Pts',(-0.549938525150295,1.,-2.04963761077958));
#34586=CARTESIAN_POINT('Ctrl Pts',(-0.554240657463906,-1.,-2.05427091604413));
#34587=CARTESIAN_POINT('Ctrl Pts',(-0.554240657463906,1.,-2.05427091604413));
#34588=CARTESIAN_POINT('Ctrl Pts',(-0.558579940185151,-1.,-2.05888537756462));
#34589=CARTESIAN_POINT('Ctrl Pts',(-0.558579940185151,1.,-2.05888537756462));
#34590=CARTESIAN_POINT('Ctrl Pts',(-0.562955993082261,-1.,-2.06348090160589));
#34591=CARTESIAN_POINT('Ctrl Pts',(-0.562955993082261,1.,-2.06348090160589));
#34592=CARTESIAN_POINT('Ctrl Pts',(-0.567368421181087,-1.,-2.06805732997334));
#34593=CARTESIAN_POINT('Ctrl Pts',(-0.567368421181087,1.,-2.06805732997334));
#34594=CARTESIAN_POINT('Ctrl Pts',(-0.571816823242603,-1.,-2.07261449292824));
#34595=CARTESIAN_POINT('Ctrl Pts',(-0.571816823242603,1.,-2.07261449292824));
#34596=CARTESIAN_POINT('Ctrl Pts',(-0.576300797416844,-1.,-2.07715226767559));
#34597=CARTESIAN_POINT('Ctrl Pts',(-0.576300797416844,1.,-2.07715226767559));
#34598=CARTESIAN_POINT('Ctrl Pts',(-0.580819952108063,-1.,-2.08167059018418));
#34599=CARTESIAN_POINT('Ctrl Pts',(-0.580819952108063,1.,-2.08167059018418));
#34600=CARTESIAN_POINT('Ctrl Pts',(-0.585373918991617,-1.,-2.08616943727951));
#34601=CARTESIAN_POINT('Ctrl Pts',(-0.585373918991617,1.,-2.08616943727951));
#34602=CARTESIAN_POINT('Ctrl Pts',(-0.589962365403406,-1.,-2.09064881812129));
#34603=CARTESIAN_POINT('Ctrl Pts',(-0.589962365403406,1.,-2.09064881812129));
#34604=CARTESIAN_POINT('Ctrl Pts',(-0.594585006052162,-1.,-2.0951087622027));
#34605=CARTESIAN_POINT('Ctrl Pts',(-0.594585006052162,1.,-2.0951087622027));
#34606=CARTESIAN_POINT('Ctrl Pts',(-0.599241616420533,-1.,-2.0995493086477));
#34607=CARTESIAN_POINT('Ctrl Pts',(-0.599241616420533,1.,-2.0995493086477));
#34608=CARTESIAN_POINT('Ctrl Pts',(-0.60393203073603,-1.,-2.10397049886949));
#34609=CARTESIAN_POINT('Ctrl Pts',(-0.60393203073603,1.,-2.10397049886949));
#34610=CARTESIAN_POINT('Ctrl Pts',(-0.607711315454876,-1.,-2.1074919961518));
#34611=CARTESIAN_POINT('Ctrl Pts',(-0.607711315454876,1.,-2.1074919961518));
#34612=CARTESIAN_POINT('Ctrl Pts',(-0.610560911689899,-1.,-2.11012443807238));
#34613=CARTESIAN_POINT('Ctrl Pts',(-0.610560911689899,1.,-2.11012443807238));
#34614=CARTESIAN_POINT('Ctrl Pts',(-0.6124673655618,-1.,-2.11187554259986));
#34615=CARTESIAN_POINT('Ctrl Pts',(-0.6124673655618,1.,-2.11187554259986));
#34616=CARTESIAN_POINT('Ctrl Pts',(-0.61342227326009,-1.,-2.11275013067528));
#34617=CARTESIAN_POINT('Ctrl Pts',(-0.61342227326009,1.,-2.11275013067528));
#34618=CARTESIAN_POINT('',(-0.383122945602004,1.,-1.7075470150345));
#34619=CARTESIAN_POINT('Ctrl Pts',(-0.383122945602004,1.,-1.7075470150345));
#34620=CARTESIAN_POINT('Ctrl Pts',(-0.384119047315542,1.,-1.71231062891958));
#34621=CARTESIAN_POINT('Ctrl Pts',(-0.38607079032701,1.,-1.72162022246158));
#34622=CARTESIAN_POINT('Ctrl Pts',(-0.388877023509191,1.,-1.7349317097561));
#34623=CARTESIAN_POINT('Ctrl Pts',(-0.392375812294307,1.,-1.75137405313962));
#34624=CARTESIAN_POINT('Ctrl Pts',(-0.39634619612042,1.,-1.7697556004756));
#34625=CARTESIAN_POINT('Ctrl Pts',(-0.39991940378308,1.,-1.78598826347533));
#34626=CARTESIAN_POINT('Ctrl Pts',(-0.403107976170441,1.,-1.80012077176221));
#34627=CARTESIAN_POINT('Ctrl Pts',(-0.405933518411838,1.,-1.81223801813988));
#34628=CARTESIAN_POINT('Ctrl Pts',(-0.408428948108533,1.,-1.8224702267854));
#34629=CARTESIAN_POINT('Ctrl Pts',(-0.410641256301675,1.,-1.83100408895216));
#34630=CARTESIAN_POINT('Ctrl Pts',(-0.412633125322162,1.,-1.83808953475839));
#34631=CARTESIAN_POINT('Ctrl Pts',(-0.41448743825434,1.,-1.8440575707371));
#34632=CARTESIAN_POINT('Ctrl Pts',(-0.416300022038864,1.,-1.84929312929882));
#34633=CARTESIAN_POINT('Ctrl Pts',(-0.418164129143534,1.,-1.85417632856234));
#34634=CARTESIAN_POINT('Ctrl Pts',(-0.420157287975619,1.,-1.85903281096686));
#34635=CARTESIAN_POINT('Ctrl Pts',(-0.422327307418275,1.,-1.86408083334028));
#34636=CARTESIAN_POINT('Ctrl Pts',(-0.424678177291359,1.,-1.86937803944323));
#34637=CARTESIAN_POINT('Ctrl Pts',(-0.427183828519102,1.,-1.87486989291484));
#34638=CARTESIAN_POINT('Ctrl Pts',(-0.429803062482344,1.,-1.88044229001832));
#34639=CARTESIAN_POINT('Ctrl Pts',(-0.432493038548748,1.,-1.88596913666793));
#34640=CARTESIAN_POINT('Ctrl Pts',(-0.435225660963383,1.,-1.89136993975504));
#34641=CARTESIAN_POINT('Ctrl Pts',(-0.437995003948244,1.,-1.89663648956466));
#34642=CARTESIAN_POINT('Ctrl Pts',(-0.440807833704038,1.,-1.90180124389086));
#34643=CARTESIAN_POINT('Ctrl Pts',(-0.443677556849151,1.,-1.90691756144898));
#34644=CARTESIAN_POINT('Ctrl Pts',(-0.446617343485711,1.,-1.9120369998112));
#34645=CARTESIAN_POINT('Ctrl Pts',(-0.449632260106662,1.,-1.91718342555755));
#34646=CARTESIAN_POINT('Ctrl Pts',(-0.452719478359432,1.,-1.92235380648502));
#34647=CARTESIAN_POINT('Ctrl Pts',(-0.455872005174371,1.,-1.92753067150476));
#34648=CARTESIAN_POINT('Ctrl Pts',(-0.459081234547926,1.,-1.93269066517934));
#34649=CARTESIAN_POINT('Ctrl Pts',(-0.462340031009056,1.,-1.93781486640821));
#34650=CARTESIAN_POINT('Ctrl Pts',(-0.46564546202603,1.,-1.9428979419619));
#34651=CARTESIAN_POINT('Ctrl Pts',(-0.468997482913135,1.,-1.94794381136514));
#34652=CARTESIAN_POINT('Ctrl Pts',(-0.472397672264072,1.,-1.95296148278133));
#34653=CARTESIAN_POINT('Ctrl Pts',(-0.475848034683176,1.,-1.95796111148177));
#34654=CARTESIAN_POINT('Ctrl Pts',(-0.479349583074855,1.,-1.96294933055943));
#34655=CARTESIAN_POINT('Ctrl Pts',(-0.482901662120691,1.,-1.96792703422362));
#34656=CARTESIAN_POINT('Ctrl Pts',(-0.486502692907659,1.,-1.97289186263272));
#34657=CARTESIAN_POINT('Ctrl Pts',(-0.490150627860952,1.,-1.97783973019229));
#34658=CARTESIAN_POINT('Ctrl Pts',(-0.493843476541495,1.,-1.98276658761821));
#34659=CARTESIAN_POINT('Ctrl Pts',(-0.497579909545574,1.,-1.98767044752932));
#34660=CARTESIAN_POINT('Ctrl Pts',(-0.501359287727146,1.,-1.99255149126155));
#34661=CARTESIAN_POINT('Ctrl Pts',(-0.505181361323026,1.,-1.99741107463572));
#34662=CARTESIAN_POINT('Ctrl Pts',(-0.509046069886157,1.,-2.00225107134734));
#34663=CARTESIAN_POINT('Ctrl Pts',(-0.512953306961792,1.,-2.00707309946949));
#34664=CARTESIAN_POINT('Ctrl Pts',(-0.516902681728687,1.,-2.01187773939242));
#34665=CARTESIAN_POINT('Ctrl Pts',(-0.52089359039937,1.,-2.01666477917286));
#34666=CARTESIAN_POINT('Ctrl Pts',(-0.524925318333476,1.,-2.02143356304698));
#34667=CARTESIAN_POINT('Ctrl Pts',(-0.528997127241914,1.,-2.0261832908329));
#34668=CARTESIAN_POINT('Ctrl Pts',(-0.533108355132977,1.,-2.03091336214426));
#34669=CARTESIAN_POINT('Ctrl Pts',(-0.537258489833262,1.,-2.03562362954037));
#34670=CARTESIAN_POINT('Ctrl Pts',(-0.541447120615659,1.,-2.04031422690527));
#34671=CARTESIAN_POINT('Ctrl Pts',(-0.54567390381743,1.,-2.04498544714588));
#34672=CARTESIAN_POINT('Ctrl Pts',(-0.549938525150295,1.,-2.04963761077958));
#34673=CARTESIAN_POINT('Ctrl Pts',(-0.554240657463906,1.,-2.05427091604413));
#34674=CARTESIAN_POINT('Ctrl Pts',(-0.558579940185151,1.,-2.05888537756462));
#34675=CARTESIAN_POINT('Ctrl Pts',(-0.562955993082261,1.,-2.06348090160589));
#34676=CARTESIAN_POINT('Ctrl Pts',(-0.567368421181087,1.,-2.06805732997334));
#34677=CARTESIAN_POINT('Ctrl Pts',(-0.571816823242603,1.,-2.07261449292824));
#34678=CARTESIAN_POINT('Ctrl Pts',(-0.576300797416844,1.,-2.07715226767559));
#34679=CARTESIAN_POINT('Ctrl Pts',(-0.580819952108063,1.,-2.08167059018418));
#34680=CARTESIAN_POINT('Ctrl Pts',(-0.585373918991617,1.,-2.08616943727951));
#34681=CARTESIAN_POINT('Ctrl Pts',(-0.589962365403406,1.,-2.09064881812129));
#34682=CARTESIAN_POINT('Ctrl Pts',(-0.594585006052162,1.,-2.0951087622027));
#34683=CARTESIAN_POINT('Ctrl Pts',(-0.599241616420533,1.,-2.0995493086477));
#34684=CARTESIAN_POINT('Ctrl Pts',(-0.60393203073603,1.,-2.10397049886949));
#34685=CARTESIAN_POINT('Ctrl Pts',(-0.607711315454876,1.,-2.1074919961518));
#34686=CARTESIAN_POINT('Ctrl Pts',(-0.610560911689899,1.,-2.11012443807238));
#34687=CARTESIAN_POINT('Ctrl Pts',(-0.6124673655618,1.,-2.11187554259986));
#34688=CARTESIAN_POINT('Ctrl Pts',(-0.61342227326009,1.,-2.11275013067528));
#34689=CARTESIAN_POINT('',(-0.383122945602003,0.,-1.7075470150345));
#34690=CARTESIAN_POINT('Origin',(0.,0.,0.));
#34691=CARTESIAN_POINT('',(-0.163289472382896,1.,-1.74236521665491));
#34692=CARTESIAN_POINT('Origin',(0.,1.,0.));
#34693=CARTESIAN_POINT('',(-0.163289472382896,0.,-1.74236521665491));
#34694=CARTESIAN_POINT('Ctrl Pts',(-0.0694764450219581,-1.,-2.19890268624765));
#34695=CARTESIAN_POINT('Ctrl Pts',(-0.0694764450219581,1.,-2.19890268624765));
#34696=CARTESIAN_POINT('Ctrl Pts',(-0.070114353632549,-1.,-2.19777582085423));
#34697=CARTESIAN_POINT('Ctrl Pts',(-0.070114353632549,1.,-2.19777582085423));
#34698=CARTESIAN_POINT('Ctrl Pts',(-0.0713863779526154,-1.,-2.19552129484002));
#34699=CARTESIAN_POINT('Ctrl Pts',(-0.0713863779526154,1.,-2.19552129484002));
#34700=CARTESIAN_POINT('Ctrl Pts',(-0.0732830357306725,-1.,-2.19213712013662));
#34701=CARTESIAN_POINT('Ctrl Pts',(-0.0732830357306725,1.,-2.19213712013662));
#34702=CARTESIAN_POINT('Ctrl Pts',(-0.0757891465836148,-1.,-2.1876201139953));
#34703=CARTESIAN_POINT('Ctrl Pts',(-0.0757891465836148,1.,-2.1876201139953));
#34704=CARTESIAN_POINT('Ctrl Pts',(-0.0788837727685243,-1.,-2.18196589448887));
#34705=CARTESIAN_POINT('Ctrl Pts',(-0.0788837727685243,1.,-2.18196589448887));
#34706=CARTESIAN_POINT('Ctrl Pts',(-0.0819402680872765,-1.,-2.176303712113));
#34707=CARTESIAN_POINT('Ctrl Pts',(-0.0819402680872765,1.,-2.176303712113));
#34708=CARTESIAN_POINT('Ctrl Pts',(-0.0849584620835372,-1.,-2.17063357870952));
#34709=CARTESIAN_POINT('Ctrl Pts',(-0.0849584620835372,1.,-2.17063357870952));
#34710=CARTESIAN_POINT('Ctrl Pts',(-0.0879381291386923,-1.,-2.16495552645014));
#34711=CARTESIAN_POINT('Ctrl Pts',(-0.0879381291386923,1.,-2.16495552645014));
#34712=CARTESIAN_POINT('Ctrl Pts',(-0.0908789888107265,-1.,-2.15926961544516));
#34713=CARTESIAN_POINT('Ctrl Pts',(-0.0908789888107265,1.,-2.15926961544516));
#34714=CARTESIAN_POINT('Ctrl Pts',(-0.0937807218867643,-1.,-2.1535759397817));
#34715=CARTESIAN_POINT('Ctrl Pts',(-0.0937807218867643,1.,-2.1535759397817));
#34716=CARTESIAN_POINT('Ctrl Pts',(-0.0966429852305459,-1.,-2.14787463531795));
#34717=CARTESIAN_POINT('Ctrl Pts',(-0.0966429852305459,1.,-2.14787463531795));
#34718=CARTESIAN_POINT('Ctrl Pts',(-0.0994654261990915,-1.,-2.14216588396025));
#34719=CARTESIAN_POINT('Ctrl Pts',(-0.0994654261990915,1.,-2.14216588396025));
#34720=CARTESIAN_POINT('Ctrl Pts',(-0.1022477005561,-1.,-2.13644992667165));
#34721=CARTESIAN_POINT('Ctrl Pts',(-0.1022477005561,1.,-2.13644992667165));
#34722=CARTESIAN_POINT('Ctrl Pts',(-0.104989479152739,-1.,-2.13072704887293));
#34723=CARTESIAN_POINT('Ctrl Pts',(-0.104989479152739,1.,-2.13072704887293));
#34724=CARTESIAN_POINT('Ctrl Pts',(-0.10769043523109,-1.,-2.12499752307));
#34725=CARTESIAN_POINT('Ctrl Pts',(-0.10769043523109,1.,-2.12499752307));
#34726=CARTESIAN_POINT('Ctrl Pts',(-0.110350236135025,-1.,-2.11926155590865));
#34727=CARTESIAN_POINT('Ctrl Pts',(-0.110350236135025,1.,-2.11926155590865));
#34728=CARTESIAN_POINT('Ctrl Pts',(-0.112968534419737,-1.,-2.11351924490306));
#34729=CARTESIAN_POINT('Ctrl Pts',(-0.112968534419737,1.,-2.11351924490306));
#34730=CARTESIAN_POINT('Ctrl Pts',(-0.115544957687926,-1.,-2.10777050261309));
#34731=CARTESIAN_POINT('Ctrl Pts',(-0.115544957687926,1.,-2.10777050261309));
#34732=CARTESIAN_POINT('Ctrl Pts',(-0.118079107988355,-1.,-2.102015121329));
#34733=CARTESIAN_POINT('Ctrl Pts',(-0.118079107988355,1.,-2.102015121329));
#34734=CARTESIAN_POINT('Ctrl Pts',(-0.120570567965122,-1.,-2.0962529286773));
#34735=CARTESIAN_POINT('Ctrl Pts',(-0.120570567965122,1.,-2.0962529286773));
#34736=CARTESIAN_POINT('Ctrl Pts',(-0.123018905621083,-1.,-2.09048392424825));
#34737=CARTESIAN_POINT('Ctrl Pts',(-0.123018905621083,1.,-2.09048392424825));
#34738=CARTESIAN_POINT('Ctrl Pts',(-0.125423679412061,-1.,-2.08470840653643));
#34739=CARTESIAN_POINT('Ctrl Pts',(-0.125423679412061,1.,-2.08470840653643));
#34740=CARTESIAN_POINT('Ctrl Pts',(-0.12778444527612,-1.,-2.07892715110987));
#34741=CARTESIAN_POINT('Ctrl Pts',(-0.12778444527612,1.,-2.07892715110987));
#34742=CARTESIAN_POINT('Ctrl Pts',(-0.130100748328403,-1.,-2.07314114713063));
#34743=CARTESIAN_POINT('Ctrl Pts',(-0.130100748328403,1.,-2.07314114713063));
#34744=CARTESIAN_POINT('Ctrl Pts',(-0.13237211154771,-1.,-2.06735123910326));
#34745=CARTESIAN_POINT('Ctrl Pts',(-0.13237211154771,1.,-2.06735123910326));
#34746=CARTESIAN_POINT('Ctrl Pts',(-0.134598026192106,-1.,-2.06155781517842));
#34747=CARTESIAN_POINT('Ctrl Pts',(-0.134598026192106,1.,-2.06155781517842));
#34748=CARTESIAN_POINT('Ctrl Pts',(-0.136777941218044,-1.,-2.05576044414264));
#34749=CARTESIAN_POINT('Ctrl Pts',(-0.136777941218044,1.,-2.05576044414264));
#34750=CARTESIAN_POINT('Ctrl Pts',(-0.138911255368966,-1.,-2.04995762001328));
#34751=CARTESIAN_POINT('Ctrl Pts',(-0.138911255368966,1.,-2.04995762001328));
#34752=CARTESIAN_POINT('Ctrl Pts',(-0.140997332152546,-1.,-2.04414757947916));
#34753=CARTESIAN_POINT('Ctrl Pts',(-0.140997332152546,1.,-2.04414757947916));
#34754=CARTESIAN_POINT('Ctrl Pts',(-0.143035515058209,-1.,-2.03832911025912));
#34755=CARTESIAN_POINT('Ctrl Pts',(-0.143035515058209,1.,-2.03832911025912));
#34756=CARTESIAN_POINT('Ctrl Pts',(-0.145025140186057,-1.,-2.03250223739942));
#34757=CARTESIAN_POINT('Ctrl Pts',(-0.145025140186057,1.,-2.03250223739942));
#34758=CARTESIAN_POINT('Ctrl Pts',(-0.146965557332583,-1.,-2.02666926182017));
#34759=CARTESIAN_POINT('Ctrl Pts',(-0.146965557332583,1.,-2.02666926182017));
#34760=CARTESIAN_POINT('Ctrl Pts',(-0.148856124775337,-1.,-2.02083464969894));
#34761=CARTESIAN_POINT('Ctrl Pts',(-0.148856124775337,1.,-2.02083464969894));
#34762=CARTESIAN_POINT('Ctrl Pts',(-0.150696157673078,-1.,-2.01500291940238));
#34763=CARTESIAN_POINT('Ctrl Pts',(-0.150696157673078,1.,-2.01500291940238));
#34764=CARTESIAN_POINT('Ctrl Pts',(-0.15248488362145,-1.,-2.00917680318424));
#34765=CARTESIAN_POINT('Ctrl Pts',(-0.15248488362145,1.,-2.00917680318424));
#34766=CARTESIAN_POINT('Ctrl Pts',(-0.154221403049722,-1.,-2.00335565310543));
#34767=CARTESIAN_POINT('Ctrl Pts',(-0.154221403049722,1.,-2.00335565310543));
#34768=CARTESIAN_POINT('Ctrl Pts',(-0.155904629548783,-1.,-1.99753284771497));
#34769=CARTESIAN_POINT('Ctrl Pts',(-0.155904629548783,1.,-1.99753284771497));
#34770=CARTESIAN_POINT('Ctrl Pts',(-0.157533331459227,-1.,-1.99169810931908));
#34771=CARTESIAN_POINT('Ctrl Pts',(-0.157533331459227,1.,-1.99169810931908));
#34772=CARTESIAN_POINT('Ctrl Pts',(-0.159106226437299,-1.,-1.98584238283292));
#34773=CARTESIAN_POINT('Ctrl Pts',(-0.159106226437299,1.,-1.98584238283292));
#34774=CARTESIAN_POINT('Ctrl Pts',(-0.160622060784611,-1.,-1.97996195437559));
#34775=CARTESIAN_POINT('Ctrl Pts',(-0.160622060784611,1.,-1.97996195437559));
#34776=CARTESIAN_POINT('Ctrl Pts',(-0.162079693556289,-1.,-1.97406280235188));
#34777=CARTESIAN_POINT('Ctrl Pts',(-0.162079693556289,1.,-1.97406280235188));
#34778=CARTESIAN_POINT('Ctrl Pts',(-0.163478185457734,-1.,-1.96816512677967));
#34779=CARTESIAN_POINT('Ctrl Pts',(-0.163478185457734,1.,-1.96816512677967));
#34780=CARTESIAN_POINT('Ctrl Pts',(-0.164816568920269,-1.,-1.96229379940136));
#34781=CARTESIAN_POINT('Ctrl Pts',(-0.164816568920269,1.,-1.96229379940136));
#34782=CARTESIAN_POINT('Ctrl Pts',(-0.166093592002812,-1.,-1.9564675971873));
#34783=CARTESIAN_POINT('Ctrl Pts',(-0.166093592002812,1.,-1.9564675971873));
#34784=CARTESIAN_POINT('Ctrl Pts',(-0.167307501784475,-1.,-1.95069027794294));
#34785=CARTESIAN_POINT('Ctrl Pts',(-0.167307501784475,1.,-1.95069027794294));
#34786=CARTESIAN_POINT('Ctrl Pts',(-0.168455741607556,-1.,-1.94493757756931));
#34787=CARTESIAN_POINT('Ctrl Pts',(-0.168455741607556,1.,-1.94493757756931));
#34788=CARTESIAN_POINT('Ctrl Pts',(-0.169534904817491,-1.,-1.93915639211581));
#34789=CARTESIAN_POINT('Ctrl Pts',(-0.169534904817491,1.,-1.93915639211581));
#34790=CARTESIAN_POINT('Ctrl Pts',(-0.170541253116202,-1.,-1.93329183155539));
#34791=CARTESIAN_POINT('Ctrl Pts',(-0.170541253116202,1.,-1.93329183155539));
#34792=CARTESIAN_POINT('Ctrl Pts',(-0.171471191532988,-1.,-1.92731093582036));
#34793=CARTESIAN_POINT('Ctrl Pts',(-0.171471191532988,1.,-1.92731093582036));
#34794=CARTESIAN_POINT('Ctrl Pts',(-0.172321621259514,-1.,-1.9212233439798));
#34795=CARTESIAN_POINT('Ctrl Pts',(-0.172321621259514,1.,-1.9212233439798));
#34796=CARTESIAN_POINT('Ctrl Pts',(-0.173090695383496,-1.,-1.91511429159527));
#34797=CARTESIAN_POINT('Ctrl Pts',(-0.173090695383496,1.,-1.91511429159527));
#34798=CARTESIAN_POINT('Ctrl Pts',(-0.173776635257817,-1.,-1.90911693975267));
#34799=CARTESIAN_POINT('Ctrl Pts',(-0.173776635257817,1.,-1.90911693975267));
#34800=CARTESIAN_POINT('Ctrl Pts',(-0.174375518661085,-1.,-1.90335253862834));
#34801=CARTESIAN_POINT('Ctrl Pts',(-0.174375518661085,1.,-1.90335253862834));
#34802=CARTESIAN_POINT('Ctrl Pts',(-0.174879405091263,-1.,-1.89788101117132));
#34803=CARTESIAN_POINT('Ctrl Pts',(-0.174879405091263,1.,-1.89788101117132));
#34804=CARTESIAN_POINT('Ctrl Pts',(-0.175274276190844,-1.,-1.892646301985));
#34805=CARTESIAN_POINT('Ctrl Pts',(-0.175274276190844,1.,-1.892646301985));
#34806=CARTESIAN_POINT('Ctrl Pts',(-0.175538155840648,-1.,-1.88742606273259));
#34807=CARTESIAN_POINT('Ctrl Pts',(-0.175538155840648,1.,-1.88742606273259));
#34808=CARTESIAN_POINT('Ctrl Pts',(-0.175644148889699,-1.,-1.88188663145367));
#34809=CARTESIAN_POINT('Ctrl Pts',(-0.175644148889699,1.,-1.88188663145367));
#34810=CARTESIAN_POINT('Ctrl Pts',(-0.175563480746485,-1.,-1.87563767773588));
#34811=CARTESIAN_POINT('Ctrl Pts',(-0.175563480746485,1.,-1.87563767773588));
#34812=CARTESIAN_POINT('Ctrl Pts',(-0.175268337590758,-1.,-1.86828349694799));
#34813=CARTESIAN_POINT('Ctrl Pts',(-0.175268337590758,1.,-1.86828349694799));
#34814=CARTESIAN_POINT('Ctrl Pts',(-0.17473525927603,-1.,-1.85948367088837));
#34815=CARTESIAN_POINT('Ctrl Pts',(-0.17473525927603,1.,-1.85948367088837));
#34816=CARTESIAN_POINT('Ctrl Pts',(-0.173946627587731,-1.,-1.8489811319852));
#34817=CARTESIAN_POINT('Ctrl Pts',(-0.173946627587731,1.,-1.8489811319852));
#34818=CARTESIAN_POINT('Ctrl Pts',(-0.1728894428919,-1.,-1.83658380527692));
#34819=CARTESIAN_POINT('Ctrl Pts',(-0.1728894428919,1.,-1.83658380527692));
#34820=CARTESIAN_POINT('Ctrl Pts',(-0.171554770204119,-1.,-1.82215766811545));
#34821=CARTESIAN_POINT('Ctrl Pts',(-0.171554770204119,1.,-1.82215766811545));
#34822=CARTESIAN_POINT('Ctrl Pts',(-0.169936923904608,-1.,-1.80561530629706));
#34823=CARTESIAN_POINT('Ctrl Pts',(-0.169936923904608,1.,-1.80561530629706));
#34824=CARTESIAN_POINT('Ctrl Pts',(-0.168032772805197,-1.,-1.7869064998507));
#34825=CARTESIAN_POINT('Ctrl Pts',(-0.168032772805197,1.,-1.7869064998507));
#34826=CARTESIAN_POINT('Ctrl Pts',(-0.1662793551464,-1.,-1.77018771684844));
#34827=CARTESIAN_POINT('Ctrl Pts',(-0.1662793551464,1.,-1.77018771684844));
#34828=CARTESIAN_POINT('Ctrl Pts',(-0.164834765707158,-1.,-1.75666056638427));
#34829=CARTESIAN_POINT('Ctrl Pts',(-0.164834765707158,1.,-1.75666056638427));
#34830=CARTESIAN_POINT('Ctrl Pts',(-0.163814161002002,-1.,-1.7472034950333));
#34831=CARTESIAN_POINT('Ctrl Pts',(-0.163814161002002,1.,-1.7472034950333));
#34832=CARTESIAN_POINT('Ctrl Pts',(-0.163289472382896,-1.,-1.74236521665491));
#34833=CARTESIAN_POINT('Ctrl Pts',(-0.163289472382896,1.,-1.74236521665491));
#34834=CARTESIAN_POINT('',(-0.0694764450219581,1.,-2.19890268624765));
#34835=CARTESIAN_POINT('Ctrl Pts',(-0.0694764450219581,1.,-2.19890268624765));
#34836=CARTESIAN_POINT('Ctrl Pts',(-0.070114353632549,1.,-2.19777582085423));
#34837=CARTESIAN_POINT('Ctrl Pts',(-0.0713863779526154,1.,-2.19552129484002));
#34838=CARTESIAN_POINT('Ctrl Pts',(-0.0732830357306725,1.,-2.19213712013662));
#34839=CARTESIAN_POINT('Ctrl Pts',(-0.0757891465836148,1.,-2.1876201139953));
#34840=CARTESIAN_POINT('Ctrl Pts',(-0.0788837727685243,1.,-2.18196589448887));
#34841=CARTESIAN_POINT('Ctrl Pts',(-0.0819402680872765,1.,-2.176303712113));
#34842=CARTESIAN_POINT('Ctrl Pts',(-0.0849584620835372,1.,-2.17063357870952));
#34843=CARTESIAN_POINT('Ctrl Pts',(-0.0879381291386923,1.,-2.16495552645014));
#34844=CARTESIAN_POINT('Ctrl Pts',(-0.0908789888107265,1.,-2.15926961544516));
#34845=CARTESIAN_POINT('Ctrl Pts',(-0.0937807218867643,1.,-2.1535759397817));
#34846=CARTESIAN_POINT('Ctrl Pts',(-0.0966429852305459,1.,-2.14787463531795));
#34847=CARTESIAN_POINT('Ctrl Pts',(-0.0994654261990915,1.,-2.14216588396025));
#34848=CARTESIAN_POINT('Ctrl Pts',(-0.1022477005561,1.,-2.13644992667165));
#34849=CARTESIAN_POINT('Ctrl Pts',(-0.104989479152739,1.,-2.13072704887293));
#34850=CARTESIAN_POINT('Ctrl Pts',(-0.10769043523109,1.,-2.12499752307));
#34851=CARTESIAN_POINT('Ctrl Pts',(-0.110350236135025,1.,-2.11926155590865));
#34852=CARTESIAN_POINT('Ctrl Pts',(-0.112968534419737,1.,-2.11351924490306));
#34853=CARTESIAN_POINT('Ctrl Pts',(-0.115544957687926,1.,-2.10777050261309));
#34854=CARTESIAN_POINT('Ctrl Pts',(-0.118079107988355,1.,-2.102015121329));
#34855=CARTESIAN_POINT('Ctrl Pts',(-0.120570567965122,1.,-2.0962529286773));
#34856=CARTESIAN_POINT('Ctrl Pts',(-0.123018905621083,1.,-2.09048392424825));
#34857=CARTESIAN_POINT('Ctrl Pts',(-0.125423679412061,1.,-2.08470840653643));
#34858=CARTESIAN_POINT('Ctrl Pts',(-0.12778444527612,1.,-2.07892715110987));
#34859=CARTESIAN_POINT('Ctrl Pts',(-0.130100748328403,1.,-2.07314114713063));
#34860=CARTESIAN_POINT('Ctrl Pts',(-0.13237211154771,1.,-2.06735123910326));
#34861=CARTESIAN_POINT('Ctrl Pts',(-0.134598026192106,1.,-2.06155781517842));
#34862=CARTESIAN_POINT('Ctrl Pts',(-0.136777941218044,1.,-2.05576044414264));
#34863=CARTESIAN_POINT('Ctrl Pts',(-0.138911255368966,1.,-2.04995762001328));
#34864=CARTESIAN_POINT('Ctrl Pts',(-0.140997332152546,1.,-2.04414757947916));
#34865=CARTESIAN_POINT('Ctrl Pts',(-0.143035515058209,1.,-2.03832911025912));
#34866=CARTESIAN_POINT('Ctrl Pts',(-0.145025140186057,1.,-2.03250223739942));
#34867=CARTESIAN_POINT('Ctrl Pts',(-0.146965557332583,1.,-2.02666926182017));
#34868=CARTESIAN_POINT('Ctrl Pts',(-0.148856124775337,1.,-2.02083464969894));
#34869=CARTESIAN_POINT('Ctrl Pts',(-0.150696157673078,1.,-2.01500291940238));
#34870=CARTESIAN_POINT('Ctrl Pts',(-0.15248488362145,1.,-2.00917680318424));
#34871=CARTESIAN_POINT('Ctrl Pts',(-0.154221403049722,1.,-2.00335565310543));
#34872=CARTESIAN_POINT('Ctrl Pts',(-0.155904629548783,1.,-1.99753284771497));
#34873=CARTESIAN_POINT('Ctrl Pts',(-0.157533331459227,1.,-1.99169810931908));
#34874=CARTESIAN_POINT('Ctrl Pts',(-0.159106226437299,1.,-1.98584238283292));
#34875=CARTESIAN_POINT('Ctrl Pts',(-0.160622060784611,1.,-1.97996195437559));
#34876=CARTESIAN_POINT('Ctrl Pts',(-0.162079693556289,1.,-1.97406280235188));
#34877=CARTESIAN_POINT('Ctrl Pts',(-0.163478185457734,1.,-1.96816512677967));
#34878=CARTESIAN_POINT('Ctrl Pts',(-0.164816568920269,1.,-1.96229379940136));
#34879=CARTESIAN_POINT('Ctrl Pts',(-0.166093592002812,1.,-1.9564675971873));
#34880=CARTESIAN_POINT('Ctrl Pts',(-0.167307501784475,1.,-1.95069027794294));
#34881=CARTESIAN_POINT('Ctrl Pts',(-0.168455741607556,1.,-1.94493757756931));
#34882=CARTESIAN_POINT('Ctrl Pts',(-0.169534904817491,1.,-1.93915639211581));
#34883=CARTESIAN_POINT('Ctrl Pts',(-0.170541253116202,1.,-1.93329183155539));
#34884=CARTESIAN_POINT('Ctrl Pts',(-0.171471191532988,1.,-1.92731093582036));
#34885=CARTESIAN_POINT('Ctrl Pts',(-0.172321621259514,1.,-1.9212233439798));
#34886=CARTESIAN_POINT('Ctrl Pts',(-0.173090695383496,1.,-1.91511429159527));
#34887=CARTESIAN_POINT('Ctrl Pts',(-0.173776635257817,1.,-1.90911693975267));
#34888=CARTESIAN_POINT('Ctrl Pts',(-0.174375518661085,1.,-1.90335253862834));
#34889=CARTESIAN_POINT('Ctrl Pts',(-0.174879405091263,1.,-1.89788101117132));
#34890=CARTESIAN_POINT('Ctrl Pts',(-0.175274276190844,1.,-1.892646301985));
#34891=CARTESIAN_POINT('Ctrl Pts',(-0.175538155840648,1.,-1.88742606273259));
#34892=CARTESIAN_POINT('Ctrl Pts',(-0.175644148889699,1.,-1.88188663145367));
#34893=CARTESIAN_POINT('Ctrl Pts',(-0.175563480746485,1.,-1.87563767773588));
#34894=CARTESIAN_POINT('Ctrl Pts',(-0.175268337590758,1.,-1.86828349694799));
#34895=CARTESIAN_POINT('Ctrl Pts',(-0.17473525927603,1.,-1.85948367088837));
#34896=CARTESIAN_POINT('Ctrl Pts',(-0.173946627587731,1.,-1.8489811319852));
#34897=CARTESIAN_POINT('Ctrl Pts',(-0.1728894428919,1.,-1.83658380527692));
#34898=CARTESIAN_POINT('Ctrl Pts',(-0.171554770204119,1.,-1.82215766811545));
#34899=CARTESIAN_POINT('Ctrl Pts',(-0.169936923904608,1.,-1.80561530629706));
#34900=CARTESIAN_POINT('Ctrl Pts',(-0.168032772805197,1.,-1.7869064998507));
#34901=CARTESIAN_POINT('Ctrl Pts',(-0.1662793551464,1.,-1.77018771684844));
#34902=CARTESIAN_POINT('Ctrl Pts',(-0.164834765707158,1.,-1.75666056638427));
#34903=CARTESIAN_POINT('Ctrl Pts',(-0.163814161002002,1.,-1.7472034950333));
#34904=CARTESIAN_POINT('Ctrl Pts',(-0.163289472382896,1.,-1.74236521665491));
#34905=CARTESIAN_POINT('',(-0.0694764450219581,0.,-2.19890268624765));
#34906=CARTESIAN_POINT('Origin',(0.0694764450219584,0.,-2.19890268624765));
#34907=CARTESIAN_POINT('',(0.0694764450219584,1.,-2.19890268624765));
#34908=CARTESIAN_POINT('',(-0.0694764450219581,1.,-2.19890268624765));
#34909=CARTESIAN_POINT('',(0.0694764450219584,0.,-2.19890268624765));
#34910=CARTESIAN_POINT('Ctrl Pts',(0.163289472382896,-1.,-1.74236521665491));
#34911=CARTESIAN_POINT('Ctrl Pts',(0.163289472382896,1.,-1.74236521665491));
#34912=CARTESIAN_POINT('Ctrl Pts',(0.163814161002474,-1.,-1.74720349503904));
#34913=CARTESIAN_POINT('Ctrl Pts',(0.163814161002474,1.,-1.74720349503904));
#34914=CARTESIAN_POINT('Ctrl Pts',(0.164834765708484,-1.,-1.75666056640041));
#34915=CARTESIAN_POINT('Ctrl Pts',(0.164834765708484,1.,-1.75666056640041));
#34916=CARTESIAN_POINT('Ctrl Pts',(0.166279355148738,-1.,-1.77018771687692));
#34917=CARTESIAN_POINT('Ctrl Pts',(0.166279355148738,1.,-1.77018771687692));
#34918=CARTESIAN_POINT('Ctrl Pts',(0.16803277280837,-1.,-1.78690649988931));
#34919=CARTESIAN_POINT('Ctrl Pts',(0.16803277280837,1.,-1.78690649988931));
#34920=CARTESIAN_POINT('Ctrl Pts',(0.169936923908078,-1.,-1.80561530633924));
#34921=CARTESIAN_POINT('Ctrl Pts',(0.169936923908078,1.,-1.80561530633924));
#34922=CARTESIAN_POINT('Ctrl Pts',(0.171554770207306,-1.,-1.82215766815414));
#34923=CARTESIAN_POINT('Ctrl Pts',(0.171554770207306,1.,-1.82215766815414));
#34924=CARTESIAN_POINT('Ctrl Pts',(0.17288944289442,-1.,-1.83658380530747));
#34925=CARTESIAN_POINT('Ctrl Pts',(0.17288944289442,1.,-1.83658380530747));
#34926=CARTESIAN_POINT('Ctrl Pts',(0.173946627589401,-1.,-1.84898113200543));
#34927=CARTESIAN_POINT('Ctrl Pts',(0.173946627589401,1.,-1.84898113200543));
#34928=CARTESIAN_POINT('Ctrl Pts',(0.174735259276856,-1.,-1.85948367089838));
#34929=CARTESIAN_POINT('Ctrl Pts',(0.174735259276856,1.,-1.85948367089838));
#34930=CARTESIAN_POINT('Ctrl Pts',(0.175268337590901,-1.,-1.86828349694972));
#34931=CARTESIAN_POINT('Ctrl Pts',(0.175268337590901,1.,-1.86828349694972));
#34932=CARTESIAN_POINT('Ctrl Pts',(0.175563480746205,-1.,-1.87563767773249));
#34933=CARTESIAN_POINT('Ctrl Pts',(0.175563480746205,1.,-1.87563767773249));
#34934=CARTESIAN_POINT('Ctrl Pts',(0.175644148889271,-1.,-1.88188663144846));
#34935=CARTESIAN_POINT('Ctrl Pts',(0.175644148889271,1.,-1.88188663144846));
#34936=CARTESIAN_POINT('Ctrl Pts',(0.175538155840286,-1.,-1.88742606272818));
#34937=CARTESIAN_POINT('Ctrl Pts',(0.175538155840286,1.,-1.88742606272818));
#34938=CARTESIAN_POINT('Ctrl Pts',(0.175274276190664,-1.,-1.89264630198279));
#34939=CARTESIAN_POINT('Ctrl Pts',(0.175274276190664,1.,-1.89264630198279));
#34940=CARTESIAN_POINT('Ctrl Pts',(0.174879405091277,-1.,-1.89788101117148));
#34941=CARTESIAN_POINT('Ctrl Pts',(0.174879405091277,1.,-1.89788101117148));
#34942=CARTESIAN_POINT('Ctrl Pts',(0.174375518661222,-1.,-1.90335253863003));
#34943=CARTESIAN_POINT('Ctrl Pts',(0.174375518661222,1.,-1.90335253863003));
#34944=CARTESIAN_POINT('Ctrl Pts',(0.173776635257984,-1.,-1.90911693975475));
#34945=CARTESIAN_POINT('Ctrl Pts',(0.173776635257984,1.,-1.90911693975475));
#34946=CARTESIAN_POINT('Ctrl Pts',(0.173090695383619,-1.,-1.91511429159681));
#34947=CARTESIAN_POINT('Ctrl Pts',(0.173090695383619,1.,-1.91511429159681));
#34948=CARTESIAN_POINT('Ctrl Pts',(0.172321621259557,-1.,-1.92122334398034));
#34949=CARTESIAN_POINT('Ctrl Pts',(0.172321621259557,1.,-1.92122334398034));
#34950=CARTESIAN_POINT('Ctrl Pts',(0.17147119153296,-1.,-1.92731093582));
#34951=CARTESIAN_POINT('Ctrl Pts',(0.17147119153296,1.,-1.92731093582));
#34952=CARTESIAN_POINT('Ctrl Pts',(0.170541253116136,-1.,-1.93329183155455));
#34953=CARTESIAN_POINT('Ctrl Pts',(0.170541253116136,1.,-1.93329183155455));
#34954=CARTESIAN_POINT('Ctrl Pts',(0.169534904817425,-1.,-1.93915639211497));
#34955=CARTESIAN_POINT('Ctrl Pts',(0.169534904817425,1.,-1.93915639211497));
#34956=CARTESIAN_POINT('Ctrl Pts',(0.168455741607516,-1.,-1.94493757756879));
#34957=CARTESIAN_POINT('Ctrl Pts',(0.168455741607516,1.,-1.94493757756879));
#34958=CARTESIAN_POINT('Ctrl Pts',(0.167307501784469,-1.,-1.95069027794286));
#34959=CARTESIAN_POINT('Ctrl Pts',(0.167307501784469,1.,-1.95069027794286));
#34960=CARTESIAN_POINT('Ctrl Pts',(0.166093592002833,-1.,-1.95646759718755));
#34961=CARTESIAN_POINT('Ctrl Pts',(0.166093592002833,1.,-1.95646759718755));
#34962=CARTESIAN_POINT('Ctrl Pts',(0.1648165689203,-1.,-1.96229379940174));
#34963=CARTESIAN_POINT('Ctrl Pts',(0.1648165689203,1.,-1.96229379940174));
#34964=CARTESIAN_POINT('Ctrl Pts',(0.16347818545776,-1.,-1.96816512678));
#34965=CARTESIAN_POINT('Ctrl Pts',(0.16347818545776,1.,-1.96816512678));
#34966=CARTESIAN_POINT('Ctrl Pts',(0.162079693556302,-1.,-1.97406280235204));
#34967=CARTESIAN_POINT('Ctrl Pts',(0.162079693556302,1.,-1.97406280235204));
#34968=CARTESIAN_POINT('Ctrl Pts',(0.16062206078461,-1.,-1.97996195437557));
#34969=CARTESIAN_POINT('Ctrl Pts',(0.16062206078461,1.,-1.97996195437557));
#34970=CARTESIAN_POINT('Ctrl Pts',(0.159106226437288,-1.,-1.98584238283279));
#34971=CARTESIAN_POINT('Ctrl Pts',(0.159106226437288,1.,-1.98584238283279));
#34972=CARTESIAN_POINT('Ctrl Pts',(0.157533331459215,-1.,-1.99169810931893));
#34973=CARTESIAN_POINT('Ctrl Pts',(0.157533331459215,1.,-1.99169810931893));
#34974=CARTESIAN_POINT('Ctrl Pts',(0.155904629548774,-1.,-1.99753284771487));
#34975=CARTESIAN_POINT('Ctrl Pts',(0.155904629548774,1.,-1.99753284771487));
#34976=CARTESIAN_POINT('Ctrl Pts',(0.154221403049719,-1.,-2.00335565310539));
#34977=CARTESIAN_POINT('Ctrl Pts',(0.154221403049719,1.,-2.00335565310539));
#34978=CARTESIAN_POINT('Ctrl Pts',(0.152484883621452,-1.,-2.00917680318426));
#34979=CARTESIAN_POINT('Ctrl Pts',(0.152484883621452,1.,-2.00917680318426));
#34980=CARTESIAN_POINT('Ctrl Pts',(0.150696157673084,-1.,-2.01500291940243));
#34981=CARTESIAN_POINT('Ctrl Pts',(0.150696157673084,1.,-2.01500291940243));
#34982=CARTESIAN_POINT('Ctrl Pts',(0.148856124775343,-1.,-2.02083464969897));
#34983=CARTESIAN_POINT('Ctrl Pts',(0.148856124775343,1.,-2.02083464969897));
#34984=CARTESIAN_POINT('Ctrl Pts',(0.146965557332586,-1.,-2.02666926182017));
#34985=CARTESIAN_POINT('Ctrl Pts',(0.146965557332586,1.,-2.02666926182017));
#34986=CARTESIAN_POINT('Ctrl Pts',(0.145025140186058,-1.,-2.03250223739941));
#34987=CARTESIAN_POINT('Ctrl Pts',(0.145025140186058,1.,-2.03250223739941));
#34988=CARTESIAN_POINT('Ctrl Pts',(0.143035515058208,-1.,-2.03832911025913));
#34989=CARTESIAN_POINT('Ctrl Pts',(0.143035515058208,1.,-2.03832911025913));
#34990=CARTESIAN_POINT('Ctrl Pts',(0.140997332152545,-1.,-2.04414757947919));
#34991=CARTESIAN_POINT('Ctrl Pts',(0.140997332152545,1.,-2.04414757947919));
#34992=CARTESIAN_POINT('Ctrl Pts',(0.138911255368966,-1.,-2.04995762001333));
#34993=CARTESIAN_POINT('Ctrl Pts',(0.138911255368966,1.,-2.04995762001333));
#34994=CARTESIAN_POINT('Ctrl Pts',(0.136777941218044,-1.,-2.0557604441427));
#34995=CARTESIAN_POINT('Ctrl Pts',(0.136777941218044,1.,-2.0557604441427));
#34996=CARTESIAN_POINT('Ctrl Pts',(0.134598026192107,-1.,-2.06155781517844));
#34997=CARTESIAN_POINT('Ctrl Pts',(0.134598026192107,1.,-2.06155781517844));
#34998=CARTESIAN_POINT('Ctrl Pts',(0.13237211154771,-1.,-2.06735123910319));
#34999=CARTESIAN_POINT('Ctrl Pts',(0.13237211154771,1.,-2.06735123910319));
#35000=CARTESIAN_POINT('Ctrl Pts',(0.1301007483284,-1.,-2.07314114713047));
#35001=CARTESIAN_POINT('Ctrl Pts',(0.1301007483284,1.,-2.07314114713047));
#35002=CARTESIAN_POINT('Ctrl Pts',(0.127784445276116,-1.,-2.07892715110967));
#35003=CARTESIAN_POINT('Ctrl Pts',(0.127784445276116,1.,-2.07892715110967));
#35004=CARTESIAN_POINT('Ctrl Pts',(0.125423679412058,-1.,-2.08470840653628));
#35005=CARTESIAN_POINT('Ctrl Pts',(0.125423679412058,1.,-2.08470840653628));
#35006=CARTESIAN_POINT('Ctrl Pts',(0.123018905621083,-1.,-2.09048392424826));
#35007=CARTESIAN_POINT('Ctrl Pts',(0.123018905621083,1.,-2.09048392424826));
#35008=CARTESIAN_POINT('Ctrl Pts',(0.120570567965129,-1.,-2.09625292867756));
#35009=CARTESIAN_POINT('Ctrl Pts',(0.120570567965129,1.,-2.09625292867756));
#35010=CARTESIAN_POINT('Ctrl Pts',(0.118079107988368,-1.,-2.10201512132945));
#35011=CARTESIAN_POINT('Ctrl Pts',(0.118079107988368,1.,-2.10201512132945));
#35012=CARTESIAN_POINT('Ctrl Pts',(0.11554495768794,-1.,-2.10777050261359));
#35013=CARTESIAN_POINT('Ctrl Pts',(0.11554495768794,1.,-2.10777050261359));
#35014=CARTESIAN_POINT('Ctrl Pts',(0.112968534419746,-1.,-2.11351924490335));
#35015=CARTESIAN_POINT('Ctrl Pts',(0.112968534419746,1.,-2.11351924490335));
#35016=CARTESIAN_POINT('Ctrl Pts',(0.11035023613502,-1.,-2.11926155590849));
#35017=CARTESIAN_POINT('Ctrl Pts',(0.11035023613502,1.,-2.11926155590849));
#35018=CARTESIAN_POINT('Ctrl Pts',(0.107690435231068,-1.,-2.12499752306927));
#35019=CARTESIAN_POINT('Ctrl Pts',(0.107690435231068,1.,-2.12499752306927));
#35020=CARTESIAN_POINT('Ctrl Pts',(0.104989479152703,-1.,-2.1307270488718));
#35021=CARTESIAN_POINT('Ctrl Pts',(0.104989479152703,1.,-2.1307270488718));
#35022=CARTESIAN_POINT('Ctrl Pts',(0.102247700556064,-1.,-2.13644992667052));
#35023=CARTESIAN_POINT('Ctrl Pts',(0.102247700556064,1.,-2.13644992667052));
#35024=CARTESIAN_POINT('Ctrl Pts',(0.0994654261990743,-1.,-2.14216588395974));
#35025=CARTESIAN_POINT('Ctrl Pts',(0.0994654261990743,1.,-2.14216588395974));
#35026=CARTESIAN_POINT('Ctrl Pts',(0.0966429852305689,-1.,-2.14787463531864));
#35027=CARTESIAN_POINT('Ctrl Pts',(0.0966429852305689,1.,-2.14787463531864));
#35028=CARTESIAN_POINT('Ctrl Pts',(0.0937807218868345,-1.,-2.15357593978377));
#35029=CARTESIAN_POINT('Ctrl Pts',(0.0937807218868345,1.,-2.15357593978377));
#35030=CARTESIAN_POINT('Ctrl Pts',(0.0908789888108266,-1.,-2.15926961544808));
#35031=CARTESIAN_POINT('Ctrl Pts',(0.0908789888108266,1.,-2.15926961544808));
#35032=CARTESIAN_POINT('Ctrl Pts',(0.0879381291387823,-1.,-2.16495552645275));
#35033=CARTESIAN_POINT('Ctrl Pts',(0.0879381291387823,1.,-2.16495552645275));
#35034=CARTESIAN_POINT('Ctrl Pts',(0.0849584620835643,-1.,-2.17063357871031));
#35035=CARTESIAN_POINT('Ctrl Pts',(0.0849584620835643,1.,-2.17063357871031));
#35036=CARTESIAN_POINT('Ctrl Pts',(0.0819402680871939,-1.,-2.1763037121106));
#35037=CARTESIAN_POINT('Ctrl Pts',(0.0819402680871939,1.,-2.1763037121106));
#35038=CARTESIAN_POINT('Ctrl Pts',(0.0788837727683228,-1.,-2.18196589448304));
#35039=CARTESIAN_POINT('Ctrl Pts',(0.0788837727683228,1.,-2.18196589448304));
#35040=CARTESIAN_POINT('Ctrl Pts',(0.0757891465833411,-1.,-2.1876201139874));
#35041=CARTESIAN_POINT('Ctrl Pts',(0.0757891465833411,1.,-2.1876201139874));
#35042=CARTESIAN_POINT('Ctrl Pts',(0.0732830357304276,-1.,-2.19213712012956));
#35043=CARTESIAN_POINT('Ctrl Pts',(0.0732830357304276,1.,-2.19213712012956));
#35044=CARTESIAN_POINT('Ctrl Pts',(0.0713863779524627,-1.,-2.19552129483562));
#35045=CARTESIAN_POINT('Ctrl Pts',(0.0713863779524627,1.,-2.19552129483562));
#35046=CARTESIAN_POINT('Ctrl Pts',(0.0701143536324926,-1.,-2.19777582085261));
#35047=CARTESIAN_POINT('Ctrl Pts',(0.0701143536324926,1.,-2.19777582085261));
#35048=CARTESIAN_POINT('Ctrl Pts',(0.0694764450219584,-1.,-2.19890268624765));
#35049=CARTESIAN_POINT('Ctrl Pts',(0.0694764450219584,1.,-2.19890268624765));
#35050=CARTESIAN_POINT('',(0.163289472382896,1.,-1.74236521665491));
#35051=CARTESIAN_POINT('Ctrl Pts',(0.163289472382896,1.,-1.74236521665491));
#35052=CARTESIAN_POINT('Ctrl Pts',(0.163814161002474,1.,-1.74720349503904));
#35053=CARTESIAN_POINT('Ctrl Pts',(0.164834765708484,1.,-1.75666056640041));
#35054=CARTESIAN_POINT('Ctrl Pts',(0.166279355148738,1.,-1.77018771687692));
#35055=CARTESIAN_POINT('Ctrl Pts',(0.16803277280837,1.,-1.78690649988931));
#35056=CARTESIAN_POINT('Ctrl Pts',(0.169936923908078,1.,-1.80561530633924));
#35057=CARTESIAN_POINT('Ctrl Pts',(0.171554770207306,1.,-1.82215766815414));
#35058=CARTESIAN_POINT('Ctrl Pts',(0.17288944289442,1.,-1.83658380530747));
#35059=CARTESIAN_POINT('Ctrl Pts',(0.173946627589401,1.,-1.84898113200543));
#35060=CARTESIAN_POINT('Ctrl Pts',(0.174735259276856,1.,-1.85948367089838));
#35061=CARTESIAN_POINT('Ctrl Pts',(0.175268337590901,1.,-1.86828349694972));
#35062=CARTESIAN_POINT('Ctrl Pts',(0.175563480746205,1.,-1.87563767773249));
#35063=CARTESIAN_POINT('Ctrl Pts',(0.175644148889271,1.,-1.88188663144846));
#35064=CARTESIAN_POINT('Ctrl Pts',(0.175538155840286,1.,-1.88742606272818));
#35065=CARTESIAN_POINT('Ctrl Pts',(0.175274276190664,1.,-1.89264630198279));
#35066=CARTESIAN_POINT('Ctrl Pts',(0.174879405091277,1.,-1.89788101117148));
#35067=CARTESIAN_POINT('Ctrl Pts',(0.174375518661222,1.,-1.90335253863003));
#35068=CARTESIAN_POINT('Ctrl Pts',(0.173776635257984,1.,-1.90911693975475));
#35069=CARTESIAN_POINT('Ctrl Pts',(0.173090695383619,1.,-1.91511429159681));
#35070=CARTESIAN_POINT('Ctrl Pts',(0.172321621259557,1.,-1.92122334398034));
#35071=CARTESIAN_POINT('Ctrl Pts',(0.17147119153296,1.,-1.92731093582));
#35072=CARTESIAN_POINT('Ctrl Pts',(0.170541253116136,1.,-1.93329183155455));
#35073=CARTESIAN_POINT('Ctrl Pts',(0.169534904817425,1.,-1.93915639211497));
#35074=CARTESIAN_POINT('Ctrl Pts',(0.168455741607516,1.,-1.94493757756879));
#35075=CARTESIAN_POINT('Ctrl Pts',(0.167307501784469,1.,-1.95069027794286));
#35076=CARTESIAN_POINT('Ctrl Pts',(0.166093592002833,1.,-1.95646759718755));
#35077=CARTESIAN_POINT('Ctrl Pts',(0.1648165689203,1.,-1.96229379940174));
#35078=CARTESIAN_POINT('Ctrl Pts',(0.16347818545776,1.,-1.96816512678));
#35079=CARTESIAN_POINT('Ctrl Pts',(0.162079693556302,1.,-1.97406280235204));
#35080=CARTESIAN_POINT('Ctrl Pts',(0.16062206078461,1.,-1.97996195437557));
#35081=CARTESIAN_POINT('Ctrl Pts',(0.159106226437288,1.,-1.98584238283279));
#35082=CARTESIAN_POINT('Ctrl Pts',(0.157533331459215,1.,-1.99169810931893));
#35083=CARTESIAN_POINT('Ctrl Pts',(0.155904629548774,1.,-1.99753284771487));
#35084=CARTESIAN_POINT('Ctrl Pts',(0.154221403049719,1.,-2.00335565310539));
#35085=CARTESIAN_POINT('Ctrl Pts',(0.152484883621452,1.,-2.00917680318426));
#35086=CARTESIAN_POINT('Ctrl Pts',(0.150696157673084,1.,-2.01500291940243));
#35087=CARTESIAN_POINT('Ctrl Pts',(0.148856124775343,1.,-2.02083464969897));
#35088=CARTESIAN_POINT('Ctrl Pts',(0.146965557332586,1.,-2.02666926182017));
#35089=CARTESIAN_POINT('Ctrl Pts',(0.145025140186058,1.,-2.03250223739941));
#35090=CARTESIAN_POINT('Ctrl Pts',(0.143035515058208,1.,-2.03832911025913));
#35091=CARTESIAN_POINT('Ctrl Pts',(0.140997332152545,1.,-2.04414757947919));
#35092=CARTESIAN_POINT('Ctrl Pts',(0.138911255368966,1.,-2.04995762001333));
#35093=CARTESIAN_POINT('Ctrl Pts',(0.136777941218044,1.,-2.0557604441427));
#35094=CARTESIAN_POINT('Ctrl Pts',(0.134598026192107,1.,-2.06155781517844));
#35095=CARTESIAN_POINT('Ctrl Pts',(0.13237211154771,1.,-2.06735123910319));
#35096=CARTESIAN_POINT('Ctrl Pts',(0.1301007483284,1.,-2.07314114713047));
#35097=CARTESIAN_POINT('Ctrl Pts',(0.127784445276116,1.,-2.07892715110967));
#35098=CARTESIAN_POINT('Ctrl Pts',(0.125423679412058,1.,-2.08470840653628));
#35099=CARTESIAN_POINT('Ctrl Pts',(0.123018905621083,1.,-2.09048392424826));
#35100=CARTESIAN_POINT('Ctrl Pts',(0.120570567965129,1.,-2.09625292867756));
#35101=CARTESIAN_POINT('Ctrl Pts',(0.118079107988368,1.,-2.10201512132945));
#35102=CARTESIAN_POINT('Ctrl Pts',(0.11554495768794,1.,-2.10777050261359));
#35103=CARTESIAN_POINT('Ctrl Pts',(0.112968534419746,1.,-2.11351924490335));
#35104=CARTESIAN_POINT('Ctrl Pts',(0.11035023613502,1.,-2.11926155590849));
#35105=CARTESIAN_POINT('Ctrl Pts',(0.107690435231068,1.,-2.12499752306927));
#35106=CARTESIAN_POINT('Ctrl Pts',(0.104989479152703,1.,-2.1307270488718));
#35107=CARTESIAN_POINT('Ctrl Pts',(0.102247700556064,1.,-2.13644992667052));
#35108=CARTESIAN_POINT('Ctrl Pts',(0.0994654261990743,1.,-2.14216588395974));
#35109=CARTESIAN_POINT('Ctrl Pts',(0.0966429852305689,1.,-2.14787463531864));
#35110=CARTESIAN_POINT('Ctrl Pts',(0.0937807218868345,1.,-2.15357593978377));
#35111=CARTESIAN_POINT('Ctrl Pts',(0.0908789888108266,1.,-2.15926961544808));
#35112=CARTESIAN_POINT('Ctrl Pts',(0.0879381291387823,1.,-2.16495552645275));
#35113=CARTESIAN_POINT('Ctrl Pts',(0.0849584620835643,1.,-2.17063357871031));
#35114=CARTESIAN_POINT('Ctrl Pts',(0.0819402680871939,1.,-2.1763037121106));
#35115=CARTESIAN_POINT('Ctrl Pts',(0.0788837727683228,1.,-2.18196589448304));
#35116=CARTESIAN_POINT('Ctrl Pts',(0.0757891465833411,1.,-2.1876201139874));
#35117=CARTESIAN_POINT('Ctrl Pts',(0.0732830357304276,1.,-2.19213712012956));
#35118=CARTESIAN_POINT('Ctrl Pts',(0.0713863779524627,1.,-2.19552129483562));
#35119=CARTESIAN_POINT('Ctrl Pts',(0.0701143536324926,1.,-2.19777582085261));
#35120=CARTESIAN_POINT('Ctrl Pts',(0.0694764450219584,1.,-2.19890268624765));
#35121=CARTESIAN_POINT('',(0.163289472382896,0.,-1.74236521665491));
#35122=CARTESIAN_POINT('Origin',(0.,0.,0.));
#35123=CARTESIAN_POINT('',(0.383122945602004,1.,-1.7075470150345));
#35124=CARTESIAN_POINT('Origin',(0.,1.,0.));
#35125=CARTESIAN_POINT('',(0.383122945602004,0.,-1.7075470150345));
#35126=CARTESIAN_POINT('Ctrl Pts',(0.61342227326009,-1.,-2.11275013067528));
#35127=CARTESIAN_POINT('Ctrl Pts',(0.61342227326009,1.,-2.11275013067528));
#35128=CARTESIAN_POINT('Ctrl Pts',(0.61246736556225,-1.,-2.11187554260142));
#35129=CARTESIAN_POINT('Ctrl Pts',(0.61246736556225,1.,-2.11187554260142));
#35130=CARTESIAN_POINT('Ctrl Pts',(0.610560911691113,-1.,-2.11012443807661));
#35131=CARTESIAN_POINT('Ctrl Pts',(0.610560911691113,1.,-2.11012443807661));
#35132=CARTESIAN_POINT('Ctrl Pts',(0.607711315456826,-1.,-2.10749199615859));
#35133=CARTESIAN_POINT('Ctrl Pts',(0.607711315456826,1.,-2.10749199615859));
#35134=CARTESIAN_POINT('Ctrl Pts',(0.603932030738212,-1.,-2.10397049887709));
#35135=CARTESIAN_POINT('Ctrl Pts',(0.603932030738212,1.,-2.10397049887709));
#35136=CARTESIAN_POINT('Ctrl Pts',(0.599241616422144,-1.,-2.09954930865331));
#35137=CARTESIAN_POINT('Ctrl Pts',(0.599241616422144,1.,-2.09954930865331));
#35138=CARTESIAN_POINT('Ctrl Pts',(0.594585006052823,-1.,-2.09510876220501));
#35139=CARTESIAN_POINT('Ctrl Pts',(0.594585006052823,1.,-2.09510876220501));
#35140=CARTESIAN_POINT('Ctrl Pts',(0.589962365403189,-1.,-2.09064881812053));
#35141=CARTESIAN_POINT('Ctrl Pts',(0.589962365403189,1.,-2.09064881812053));
#35142=CARTESIAN_POINT('Ctrl Pts',(0.585373918990895,-1.,-2.086169437277));
#35143=CARTESIAN_POINT('Ctrl Pts',(0.585373918990895,1.,-2.086169437277));
#35144=CARTESIAN_POINT('Ctrl Pts',(0.580819952107256,-1.,-2.08167059018138));
#35145=CARTESIAN_POINT('Ctrl Pts',(0.580819952107256,1.,-2.08167059018138));
#35146=CARTESIAN_POINT('Ctrl Pts',(0.576300797416274,-1.,-2.07715226767361));
#35147=CARTESIAN_POINT('Ctrl Pts',(0.576300797416274,1.,-2.07715226767361));
#35148=CARTESIAN_POINT('Ctrl Pts',(0.571816823242411,-1.,-2.07261449292758));
#35149=CARTESIAN_POINT('Ctrl Pts',(0.571816823242411,1.,-2.07261449292758));
#35150=CARTESIAN_POINT('Ctrl Pts',(0.567368421181229,-1.,-2.06805732997383));
#35151=CARTESIAN_POINT('Ctrl Pts',(0.567368421181229,1.,-2.06805732997383));
#35152=CARTESIAN_POINT('Ctrl Pts',(0.562955993082574,-1.,-2.06348090160697));
#35153=CARTESIAN_POINT('Ctrl Pts',(0.562955993082574,1.,-2.06348090160697));
#35154=CARTESIAN_POINT('Ctrl Pts',(0.558579940185467,-1.,-2.05888537756571));
#35155=CARTESIAN_POINT('Ctrl Pts',(0.558579940185467,1.,-2.05888537756571));
#35156=CARTESIAN_POINT('Ctrl Pts',(0.554240657464109,-1.,-2.05427091604482));
#35157=CARTESIAN_POINT('Ctrl Pts',(0.554240657464109,1.,-2.05427091604482));
#35158=CARTESIAN_POINT('Ctrl Pts',(0.549938525150342,-1.,-2.04963761077974));
#35159=CARTESIAN_POINT('Ctrl Pts',(0.549938525150342,1.,-2.04963761077974));
#35160=CARTESIAN_POINT('Ctrl Pts',(0.545673903817348,-1.,-2.0449854471456));
#35161=CARTESIAN_POINT('Ctrl Pts',(0.545673903817348,1.,-2.0449854471456));
#35162=CARTESIAN_POINT('Ctrl Pts',(0.54144712061552,-1.,-2.0403142269048));
#35163=CARTESIAN_POINT('Ctrl Pts',(0.54144712061552,1.,-2.0403142269048));
#35164=CARTESIAN_POINT('Ctrl Pts',(0.537258489833134,-1.,-2.03562362953993));
#35165=CARTESIAN_POINT('Ctrl Pts',(0.537258489833134,1.,-2.03562362953993));
#35166=CARTESIAN_POINT('Ctrl Pts',(0.533108355132905,-1.,-2.03091336214401));
#35167=CARTESIAN_POINT('Ctrl Pts',(0.533108355132905,1.,-2.03091336214401));
#35168=CARTESIAN_POINT('Ctrl Pts',(0.52899712724191,-1.,-2.02618329083289));
#35169=CARTESIAN_POINT('Ctrl Pts',(0.52899712724191,1.,-2.02618329083289));
#35170=CARTESIAN_POINT('Ctrl Pts',(0.524925318333518,-1.,-2.02143356304712));
#35171=CARTESIAN_POINT('Ctrl Pts',(0.524925318333518,1.,-2.02143356304712));
#35172=CARTESIAN_POINT('Ctrl Pts',(0.520893590399428,-1.,-2.01666477917306));
#35173=CARTESIAN_POINT('Ctrl Pts',(0.520893590399428,1.,-2.01666477917306));
#35174=CARTESIAN_POINT('Ctrl Pts',(0.516902681728733,-1.,-2.01187773939257));
#35175=CARTESIAN_POINT('Ctrl Pts',(0.516902681728733,1.,-2.01187773939257));
#35176=CARTESIAN_POINT('Ctrl Pts',(0.512953306961813,-1.,-2.00707309946955));
#35177=CARTESIAN_POINT('Ctrl Pts',(0.512953306961813,1.,-2.00707309946955));
#35178=CARTESIAN_POINT('Ctrl Pts',(0.509046069886152,-1.,-2.00225107134733));
#35179=CARTESIAN_POINT('Ctrl Pts',(0.509046069886152,1.,-2.00225107134733));
#35180=CARTESIAN_POINT('Ctrl Pts',(0.505181361323011,-1.,-1.99741107463567));
#35181=CARTESIAN_POINT('Ctrl Pts',(0.505181361323011,1.,-1.99741107463567));
#35182=CARTESIAN_POINT('Ctrl Pts',(0.501359287727129,-1.,-1.9925514912615));
#35183=CARTESIAN_POINT('Ctrl Pts',(0.501359287727129,1.,-1.9925514912615));
#35184=CARTESIAN_POINT('Ctrl Pts',(0.497579909545564,-1.,-1.98767044752929));
#35185=CARTESIAN_POINT('Ctrl Pts',(0.497579909545564,1.,-1.98767044752929));
#35186=CARTESIAN_POINT('Ctrl Pts',(0.493843476541492,-1.,-1.9827665876182));
#35187=CARTESIAN_POINT('Ctrl Pts',(0.493843476541492,1.,-1.9827665876182));
#35188=CARTESIAN_POINT('Ctrl Pts',(0.490150627860955,-1.,-1.97783973019229));
#35189=CARTESIAN_POINT('Ctrl Pts',(0.490150627860955,1.,-1.97783973019229));
#35190=CARTESIAN_POINT('Ctrl Pts',(0.486502692907661,-1.,-1.97289186263272));
#35191=CARTESIAN_POINT('Ctrl Pts',(0.486502692907661,1.,-1.97289186263272));
#35192=CARTESIAN_POINT('Ctrl Pts',(0.482901662120686,-1.,-1.96792703422358));
#35193=CARTESIAN_POINT('Ctrl Pts',(0.482901662120686,1.,-1.96792703422358));
#35194=CARTESIAN_POINT('Ctrl Pts',(0.479349583074846,-1.,-1.96294933055938));
#35195=CARTESIAN_POINT('Ctrl Pts',(0.479349583074846,1.,-1.96294933055938));
#35196=CARTESIAN_POINT('Ctrl Pts',(0.475848034683171,-1.,-1.95796111148175));
#35197=CARTESIAN_POINT('Ctrl Pts',(0.475848034683171,1.,-1.95796111148175));
#35198=CARTESIAN_POINT('Ctrl Pts',(0.472397672264079,-1.,-1.95296148278136));
#35199=CARTESIAN_POINT('Ctrl Pts',(0.472397672264079,1.,-1.95296148278136));
#35200=CARTESIAN_POINT('Ctrl Pts',(0.468997482913158,-1.,-1.94794381136524));
#35201=CARTESIAN_POINT('Ctrl Pts',(0.468997482913158,1.,-1.94794381136524));
#35202=CARTESIAN_POINT('Ctrl Pts',(0.465645462026064,-1.,-1.94289794196205));
#35203=CARTESIAN_POINT('Ctrl Pts',(0.465645462026064,1.,-1.94289794196205));
#35204=CARTESIAN_POINT('Ctrl Pts',(0.462340031009087,-1.,-1.93781486640834));
#35205=CARTESIAN_POINT('Ctrl Pts',(0.462340031009087,1.,-1.93781486640834));
#35206=CARTESIAN_POINT('Ctrl Pts',(0.459081234547931,-1.,-1.93269066517936));
#35207=CARTESIAN_POINT('Ctrl Pts',(0.459081234547931,1.,-1.93269066517936));
#35208=CARTESIAN_POINT('Ctrl Pts',(0.455872005174335,-1.,-1.92753067150461));
#35209=CARTESIAN_POINT('Ctrl Pts',(0.455872005174335,1.,-1.92753067150461));
#35210=CARTESIAN_POINT('Ctrl Pts',(0.452719478359356,-1.,-1.9223538064847));
#35211=CARTESIAN_POINT('Ctrl Pts',(0.452719478359356,1.,-1.9223538064847));
#35212=CARTESIAN_POINT('Ctrl Pts',(0.449632260106572,-1.,-1.91718342555717));
#35213=CARTESIAN_POINT('Ctrl Pts',(0.449632260106572,1.,-1.91718342555717));
#35214=CARTESIAN_POINT('Ctrl Pts',(0.446617343485651,-1.,-1.91203699981095));
#35215=CARTESIAN_POINT('Ctrl Pts',(0.446617343485651,1.,-1.91203699981095));
#35216=CARTESIAN_POINT('Ctrl Pts',(0.44367755684917,-1.,-1.90691756144906));
#35217=CARTESIAN_POINT('Ctrl Pts',(0.44367755684917,1.,-1.90691756144906));
#35218=CARTESIAN_POINT('Ctrl Pts',(0.44080783370416,-1.,-1.90180124389137));
#35219=CARTESIAN_POINT('Ctrl Pts',(0.44080783370416,1.,-1.90180124389137));
#35220=CARTESIAN_POINT('Ctrl Pts',(0.437995003948443,-1.,-1.89663648956549));
#35221=CARTESIAN_POINT('Ctrl Pts',(0.437995003948443,1.,-1.89663648956549));
#35222=CARTESIAN_POINT('Ctrl Pts',(0.43522566096358,-1.,-1.89136993975585));
#35223=CARTESIAN_POINT('Ctrl Pts',(0.43522566096358,1.,-1.89136993975585));
#35224=CARTESIAN_POINT('Ctrl Pts',(0.432493038548833,-1.,-1.88596913666828));
#35225=CARTESIAN_POINT('Ctrl Pts',(0.432493038548833,1.,-1.88596913666828));
#35226=CARTESIAN_POINT('Ctrl Pts',(0.429803062482217,-1.,-1.88044229001779));
#35227=CARTESIAN_POINT('Ctrl Pts',(0.429803062482217,1.,-1.88044229001779));
#35228=CARTESIAN_POINT('Ctrl Pts',(0.427183828518743,-1.,-1.87486989291334));
#35229=CARTESIAN_POINT('Ctrl Pts',(0.427183828518743,1.,-1.87486989291334));
#35230=CARTESIAN_POINT('Ctrl Pts',(0.424678177290876,-1.,-1.8693780394412));
#35231=CARTESIAN_POINT('Ctrl Pts',(0.424678177290876,1.,-1.8693780394412));
#35232=CARTESIAN_POINT('Ctrl Pts',(0.422327307417884,-1.,-1.86408083333863));
#35233=CARTESIAN_POINT('Ctrl Pts',(0.422327307417884,1.,-1.86408083333863));
#35234=CARTESIAN_POINT('Ctrl Pts',(0.420157287975583,-1.,-1.8590328109667));
#35235=CARTESIAN_POINT('Ctrl Pts',(0.420157287975583,1.,-1.8590328109667));
#35236=CARTESIAN_POINT('Ctrl Pts',(0.418164129144045,-1.,-1.8541763285645));
#35237=CARTESIAN_POINT('Ctrl Pts',(0.418164129144045,1.,-1.8541763285645));
#35238=CARTESIAN_POINT('Ctrl Pts',(0.416300022039885,-1.,-1.84929312930314));
#35239=CARTESIAN_POINT('Ctrl Pts',(0.416300022039885,1.,-1.84929312930314));
#35240=CARTESIAN_POINT('Ctrl Pts',(0.414487438255542,-1.,-1.84405757074218));
#35241=CARTESIAN_POINT('Ctrl Pts',(0.414487438255542,1.,-1.84405757074218));
#35242=CARTESIAN_POINT('Ctrl Pts',(0.412633125322945,-1.,-1.8380895347617));
#35243=CARTESIAN_POINT('Ctrl Pts',(0.412633125322945,1.,-1.8380895347617));
#35244=CARTESIAN_POINT('Ctrl Pts',(0.410641256301276,-1.,-1.83100408895047));
#35245=CARTESIAN_POINT('Ctrl Pts',(0.410641256301276,1.,-1.83100408895047));
#35246=CARTESIAN_POINT('Ctrl Pts',(0.408428948106227,-1.,-1.82247022677562));
#35247=CARTESIAN_POINT('Ctrl Pts',(0.408428948106227,1.,-1.82247022677562));
#35248=CARTESIAN_POINT('Ctrl Pts',(0.405933518407175,-1.,-1.81223801812013));
#35249=CARTESIAN_POINT('Ctrl Pts',(0.405933518407175,1.,-1.81223801812013));
#35250=CARTESIAN_POINT('Ctrl Pts',(0.403107976163396,-1.,-1.80012077173238));
#35251=CARTESIAN_POINT('Ctrl Pts',(0.403107976163396,1.,-1.80012077173238));
#35252=CARTESIAN_POINT('Ctrl Pts',(0.399919403774155,-1.,-1.78598826343754));
#35253=CARTESIAN_POINT('Ctrl Pts',(0.399919403774155,1.,-1.78598826343754));
#35254=CARTESIAN_POINT('Ctrl Pts',(0.396346196110688,-1.,-1.76975560043442));
#35255=CARTESIAN_POINT('Ctrl Pts',(0.396346196110688,1.,-1.76975560043442));
#35256=CARTESIAN_POINT('Ctrl Pts',(0.392375812285395,-1.,-1.75137405310193));
#35257=CARTESIAN_POINT('Ctrl Pts',(0.392375812285395,1.,-1.75137405310193));
#35258=CARTESIAN_POINT('Ctrl Pts',(0.388877023502615,-1.,-1.73493170972829));
#35259=CARTESIAN_POINT('Ctrl Pts',(0.388877023502615,1.,-1.73493170972829));
#35260=CARTESIAN_POINT('Ctrl Pts',(0.386070790323281,-1.,-1.72162022244582));
#35261=CARTESIAN_POINT('Ctrl Pts',(0.386070790323281,1.,-1.72162022244582));
#35262=CARTESIAN_POINT('Ctrl Pts',(0.384119047314215,-1.,-1.71231062891398));
#35263=CARTESIAN_POINT('Ctrl Pts',(0.384119047314215,1.,-1.71231062891398));
#35264=CARTESIAN_POINT('Ctrl Pts',(0.383122945602004,-1.,-1.7075470150345));
#35265=CARTESIAN_POINT('Ctrl Pts',(0.383122945602004,1.,-1.7075470150345));
#35266=CARTESIAN_POINT('',(0.61342227326009,1.,-2.11275013067528));
#35267=CARTESIAN_POINT('Ctrl Pts',(0.61342227326009,1.,-2.11275013067528));
#35268=CARTESIAN_POINT('Ctrl Pts',(0.61246736556225,1.,-2.11187554260142));
#35269=CARTESIAN_POINT('Ctrl Pts',(0.610560911691113,1.,-2.11012443807661));
#35270=CARTESIAN_POINT('Ctrl Pts',(0.607711315456826,1.,-2.10749199615859));
#35271=CARTESIAN_POINT('Ctrl Pts',(0.603932030738212,1.,-2.10397049887709));
#35272=CARTESIAN_POINT('Ctrl Pts',(0.599241616422144,1.,-2.09954930865331));
#35273=CARTESIAN_POINT('Ctrl Pts',(0.594585006052823,1.,-2.09510876220501));
#35274=CARTESIAN_POINT('Ctrl Pts',(0.589962365403189,1.,-2.09064881812053));
#35275=CARTESIAN_POINT('Ctrl Pts',(0.585373918990895,1.,-2.086169437277));
#35276=CARTESIAN_POINT('Ctrl Pts',(0.580819952107256,1.,-2.08167059018138));
#35277=CARTESIAN_POINT('Ctrl Pts',(0.576300797416274,1.,-2.07715226767361));
#35278=CARTESIAN_POINT('Ctrl Pts',(0.571816823242411,1.,-2.07261449292758));
#35279=CARTESIAN_POINT('Ctrl Pts',(0.567368421181229,1.,-2.06805732997383));
#35280=CARTESIAN_POINT('Ctrl Pts',(0.562955993082574,1.,-2.06348090160697));
#35281=CARTESIAN_POINT('Ctrl Pts',(0.558579940185467,1.,-2.05888537756571));
#35282=CARTESIAN_POINT('Ctrl Pts',(0.554240657464109,1.,-2.05427091604482));
#35283=CARTESIAN_POINT('Ctrl Pts',(0.549938525150342,1.,-2.04963761077974));
#35284=CARTESIAN_POINT('Ctrl Pts',(0.545673903817348,1.,-2.0449854471456));
#35285=CARTESIAN_POINT('Ctrl Pts',(0.54144712061552,1.,-2.0403142269048));
#35286=CARTESIAN_POINT('Ctrl Pts',(0.537258489833134,1.,-2.03562362953993));
#35287=CARTESIAN_POINT('Ctrl Pts',(0.533108355132905,1.,-2.03091336214401));
#35288=CARTESIAN_POINT('Ctrl Pts',(0.52899712724191,1.,-2.02618329083289));
#35289=CARTESIAN_POINT('Ctrl Pts',(0.524925318333518,1.,-2.02143356304712));
#35290=CARTESIAN_POINT('Ctrl Pts',(0.520893590399428,1.,-2.01666477917306));
#35291=CARTESIAN_POINT('Ctrl Pts',(0.516902681728733,1.,-2.01187773939257));
#35292=CARTESIAN_POINT('Ctrl Pts',(0.512953306961813,1.,-2.00707309946955));
#35293=CARTESIAN_POINT('Ctrl Pts',(0.509046069886152,1.,-2.00225107134733));
#35294=CARTESIAN_POINT('Ctrl Pts',(0.505181361323011,1.,-1.99741107463567));
#35295=CARTESIAN_POINT('Ctrl Pts',(0.501359287727129,1.,-1.9925514912615));
#35296=CARTESIAN_POINT('Ctrl Pts',(0.497579909545564,1.,-1.98767044752929));
#35297=CARTESIAN_POINT('Ctrl Pts',(0.493843476541492,1.,-1.9827665876182));
#35298=CARTESIAN_POINT('Ctrl Pts',(0.490150627860955,1.,-1.97783973019229));
#35299=CARTESIAN_POINT('Ctrl Pts',(0.486502692907661,1.,-1.97289186263272));
#35300=CARTESIAN_POINT('Ctrl Pts',(0.482901662120686,1.,-1.96792703422358));
#35301=CARTESIAN_POINT('Ctrl Pts',(0.479349583074846,1.,-1.96294933055938));
#35302=CARTESIAN_POINT('Ctrl Pts',(0.475848034683171,1.,-1.95796111148175));
#35303=CARTESIAN_POINT('Ctrl Pts',(0.472397672264079,1.,-1.95296148278136));
#35304=CARTESIAN_POINT('Ctrl Pts',(0.468997482913158,1.,-1.94794381136524));
#35305=CARTESIAN_POINT('Ctrl Pts',(0.465645462026064,1.,-1.94289794196205));
#35306=CARTESIAN_POINT('Ctrl Pts',(0.462340031009087,1.,-1.93781486640834));
#35307=CARTESIAN_POINT('Ctrl Pts',(0.459081234547931,1.,-1.93269066517936));
#35308=CARTESIAN_POINT('Ctrl Pts',(0.455872005174335,1.,-1.92753067150461));
#35309=CARTESIAN_POINT('Ctrl Pts',(0.452719478359356,1.,-1.9223538064847));
#35310=CARTESIAN_POINT('Ctrl Pts',(0.449632260106572,1.,-1.91718342555717));
#35311=CARTESIAN_POINT('Ctrl Pts',(0.446617343485651,1.,-1.91203699981095));
#35312=CARTESIAN_POINT('Ctrl Pts',(0.44367755684917,1.,-1.90691756144906));
#35313=CARTESIAN_POINT('Ctrl Pts',(0.44080783370416,1.,-1.90180124389137));
#35314=CARTESIAN_POINT('Ctrl Pts',(0.437995003948443,1.,-1.89663648956549));
#35315=CARTESIAN_POINT('Ctrl Pts',(0.43522566096358,1.,-1.89136993975585));
#35316=CARTESIAN_POINT('Ctrl Pts',(0.432493038548833,1.,-1.88596913666828));
#35317=CARTESIAN_POINT('Ctrl Pts',(0.429803062482217,1.,-1.88044229001779));
#35318=CARTESIAN_POINT('Ctrl Pts',(0.427183828518743,1.,-1.87486989291334));
#35319=CARTESIAN_POINT('Ctrl Pts',(0.424678177290876,1.,-1.8693780394412));
#35320=CARTESIAN_POINT('Ctrl Pts',(0.422327307417884,1.,-1.86408083333863));
#35321=CARTESIAN_POINT('Ctrl Pts',(0.420157287975583,1.,-1.8590328109667));
#35322=CARTESIAN_POINT('Ctrl Pts',(0.418164129144045,1.,-1.8541763285645));
#35323=CARTESIAN_POINT('Ctrl Pts',(0.416300022039885,1.,-1.84929312930314));
#35324=CARTESIAN_POINT('Ctrl Pts',(0.414487438255542,1.,-1.84405757074218));
#35325=CARTESIAN_POINT('Ctrl Pts',(0.412633125322945,1.,-1.8380895347617));
#35326=CARTESIAN_POINT('Ctrl Pts',(0.410641256301276,1.,-1.83100408895047));
#35327=CARTESIAN_POINT('Ctrl Pts',(0.408428948106227,1.,-1.82247022677562));
#35328=CARTESIAN_POINT('Ctrl Pts',(0.405933518407175,1.,-1.81223801812013));
#35329=CARTESIAN_POINT('Ctrl Pts',(0.403107976163396,1.,-1.80012077173238));
#35330=CARTESIAN_POINT('Ctrl Pts',(0.399919403774155,1.,-1.78598826343754));
#35331=CARTESIAN_POINT('Ctrl Pts',(0.396346196110688,1.,-1.76975560043442));
#35332=CARTESIAN_POINT('Ctrl Pts',(0.392375812285395,1.,-1.75137405310193));
#35333=CARTESIAN_POINT('Ctrl Pts',(0.388877023502615,1.,-1.73493170972829));
#35334=CARTESIAN_POINT('Ctrl Pts',(0.386070790323281,1.,-1.72162022244582));
#35335=CARTESIAN_POINT('Ctrl Pts',(0.384119047314215,1.,-1.71231062891398));
#35336=CARTESIAN_POINT('Ctrl Pts',(0.383122945602004,1.,-1.7075470150345));
#35337=CARTESIAN_POINT('',(0.61342227326009,0.,-2.11275013067528));
#35338=CARTESIAN_POINT('Origin',(0.745574324794401,0.,-2.0698113262342));
#35339=CARTESIAN_POINT('',(0.745574324794401,1.,-2.0698113262342));
#35340=CARTESIAN_POINT('',(0.61342227326009,1.,-2.11275013067528));
#35341=CARTESIAN_POINT('',(0.745574324794401,0.,-2.0698113262342));
#35342=CARTESIAN_POINT('Ctrl Pts',(0.693717979106306,-1.,-1.60662857109684));
#35343=CARTESIAN_POINT('Ctrl Pts',(0.693717979106306,1.,-1.60662857109684));
#35344=CARTESIAN_POINT('Ctrl Pts',(0.695712097881194,-1.,-1.61106790958151));
#35345=CARTESIAN_POINT('Ctrl Pts',(0.695712097881194,1.,-1.61106790958151));
#35346=CARTESIAN_POINT('Ctrl Pts',(0.699605146405088,-1.,-1.61974673472612));
#35347=CARTESIAN_POINT('Ctrl Pts',(0.699605146405088,1.,-1.61974673472612));
#35348=CARTESIAN_POINT('Ctrl Pts',(0.705159151988319,-1.,-1.63216541664676));
#35349=CARTESIAN_POINT('Ctrl Pts',(0.705159151988319,1.,-1.63216541664676));
#35350=CARTESIAN_POINT('Ctrl Pts',(0.711993139355394,-1.,-1.64752408832016));
#35351=CARTESIAN_POINT('Ctrl Pts',(0.711993139355394,1.,-1.64752408832016));
#35352=CARTESIAN_POINT('Ctrl Pts',(0.719585433804282,-1.,-1.6647288055568));
#35353=CARTESIAN_POINT('Ctrl Pts',(0.719585433804282,1.,-1.6647288055568));
#35354=CARTESIAN_POINT('Ctrl Pts',(0.726235967997433,-1.,-1.67996158455503));
#35355=CARTESIAN_POINT('Ctrl Pts',(0.726235967997433,1.,-1.67996158455503));
#35356=CARTESIAN_POINT('Ctrl Pts',(0.731963238697195,-1.,-1.69326921975743));
#35357=CARTESIAN_POINT('Ctrl Pts',(0.731963238697195,1.,-1.69326921975743));
#35358=CARTESIAN_POINT('Ctrl Pts',(0.736799665724771,-1.,-1.70473309006121));
#35359=CARTESIAN_POINT('Ctrl Pts',(0.736799665724771,1.,-1.70473309006121));
#35360=CARTESIAN_POINT('Ctrl Pts',(0.740795162032087,-1.,-1.71447789751927));
#35361=CARTESIAN_POINT('Ctrl Pts',(0.740795162032087,1.,-1.71447789751927));
#35362=CARTESIAN_POINT('Ctrl Pts',(0.744021445433764,-1.,-1.7226822991693));
#35363=CARTESIAN_POINT('Ctrl Pts',(0.744021445433764,1.,-1.7226822991693));
#35364=CARTESIAN_POINT('Ctrl Pts',(0.746574710096436,-1.,-1.72958533647399));
#35365=CARTESIAN_POINT('Ctrl Pts',(0.746574710096436,1.,-1.72958533647399));
#35366=CARTESIAN_POINT('Ctrl Pts',(0.748582462954854,-1.,-1.73550351679848));
#35367=CARTESIAN_POINT('Ctrl Pts',(0.748582462954854,1.,-1.73550351679848));
#35368=CARTESIAN_POINT('Ctrl Pts',(0.75019343597954,-1.,-1.74080458266705));
#35369=CARTESIAN_POINT('Ctrl Pts',(0.75019343597954,1.,-1.74080458266705));
#35370=CARTESIAN_POINT('Ctrl Pts',(0.751555614163629,-1.,-1.74585086852298));
#35371=CARTESIAN_POINT('Ctrl Pts',(0.751555614163629,1.,-1.74585086852298));
#35372=CARTESIAN_POINT('Ctrl Pts',(0.752797683531377,-1.,-1.75095139468809));
#35373=CARTESIAN_POINT('Ctrl Pts',(0.752797683531377,1.,-1.75095139468809));
#35374=CARTESIAN_POINT('Ctrl Pts',(0.75400925402848,-1.,-1.75631083600175));
#35375=CARTESIAN_POINT('Ctrl Pts',(0.75400925402848,1.,-1.75631083600175));
#35376=CARTESIAN_POINT('Ctrl Pts',(0.755220979975262,-1.,-1.7619781724032));
#35377=CARTESIAN_POINT('Ctrl Pts',(0.755220979975262,1.,-1.7619781724032));
#35378=CARTESIAN_POINT('Ctrl Pts',(0.756421896028403,-1.,-1.76789396003141));
#35379=CARTESIAN_POINT('Ctrl Pts',(0.756421896028403,1.,-1.76789396003141));
#35380=CARTESIAN_POINT('Ctrl Pts',(0.757578264077238,-1.,-1.77394167108342));
#35381=CARTESIAN_POINT('Ctrl Pts',(0.757578264077238,1.,-1.77394167108342));
#35382=CARTESIAN_POINT('Ctrl Pts',(0.75865062667738,-1.,-1.77999411220912));
#35383=CARTESIAN_POINT('Ctrl Pts',(0.75865062667738,1.,-1.77999411220912));
#35384=CARTESIAN_POINT('Ctrl Pts',(0.759614401109868,-1.,-1.78596964884527));
#35385=CARTESIAN_POINT('Ctrl Pts',(0.759614401109868,1.,-1.78596964884527));
#35386=CARTESIAN_POINT('Ctrl Pts',(0.760469555880425,-1.,-1.79185815610802));
#35387=CARTESIAN_POINT('Ctrl Pts',(0.760469555880425,1.,-1.79185815610802));
#35388=CARTESIAN_POINT('Ctrl Pts',(0.761229695230359,-1.,-1.79768986997735));
#35389=CARTESIAN_POINT('Ctrl Pts',(0.761229695230359,1.,-1.79768986997735));
#35390=CARTESIAN_POINT('Ctrl Pts',(0.761915336443515,-1.,-1.80351583877334));
#35391=CARTESIAN_POINT('Ctrl Pts',(0.761915336443515,1.,-1.80351583877334));
#35392=CARTESIAN_POINT('Ctrl Pts',(0.762546129464036,-1.,-1.80938551463989));
#35393=CARTESIAN_POINT('Ctrl Pts',(0.762546129464036,1.,-1.80938551463989));
#35394=CARTESIAN_POINT('Ctrl Pts',(0.763132003836783,-1.,-1.81532118405566));
#35395=CARTESIAN_POINT('Ctrl Pts',(0.763132003836783,1.,-1.81532118405566));
#35396=CARTESIAN_POINT('Ctrl Pts',(0.763673465462854,-1.,-1.82131873145297));
#35397=CARTESIAN_POINT('Ctrl Pts',(0.763673465462854,1.,-1.82131873145297));
#35398=CARTESIAN_POINT('Ctrl Pts',(0.764165902606055,-1.,-1.8273599120008));
#35399=CARTESIAN_POINT('Ctrl Pts',(0.764165902606055,1.,-1.8273599120008));
#35400=CARTESIAN_POINT('Ctrl Pts',(0.764602549687845,-1.,-1.8334207722714));
#35401=CARTESIAN_POINT('Ctrl Pts',(0.764602549687845,1.,-1.8334207722714));
#35402=CARTESIAN_POINT('Ctrl Pts',(0.764978057881687,-1.,-1.83948181064823));
#35403=CARTESIAN_POINT('Ctrl Pts',(0.764978057881687,1.,-1.83948181064823));
#35404=CARTESIAN_POINT('Ctrl Pts',(0.765291664861971,-1.,-1.84553698875911));
#35405=CARTESIAN_POINT('Ctrl Pts',(0.765291664861971,1.,-1.84553698875911));
#35406=CARTESIAN_POINT('Ctrl Pts',(0.765545710619023,-1.,-1.85158945130054));
#35407=CARTESIAN_POINT('Ctrl Pts',(0.765545710619023,1.,-1.85158945130054));
#35408=CARTESIAN_POINT('Ctrl Pts',(0.765744212909305,-1.,-1.85764741390391));
#35409=CARTESIAN_POINT('Ctrl Pts',(0.765744212909305,1.,-1.85764741390391));
#35410=CARTESIAN_POINT('Ctrl Pts',(0.765891519092557,-1.,-1.86372027063315));
#35411=CARTESIAN_POINT('Ctrl Pts',(0.765891519092557,1.,-1.86372027063315));
#35412=CARTESIAN_POINT('Ctrl Pts',(0.765990708546111,-1.,-1.86981398314345));
#35413=CARTESIAN_POINT('Ctrl Pts',(0.765990708546111,1.,-1.86981398314345));
#35414=CARTESIAN_POINT('Ctrl Pts',(0.766042837036759,-1.,-1.87592888967886));
#35415=CARTESIAN_POINT('Ctrl Pts',(0.766042837036759,1.,-1.87592888967886));
#35416=CARTESIAN_POINT('Ctrl Pts',(0.766047794851868,-1.,-1.88206215302561));
#35417=CARTESIAN_POINT('Ctrl Pts',(0.766047794851868,1.,-1.88206215302561));
#35418=CARTESIAN_POINT('Ctrl Pts',(0.76600483706209,-1.,-1.88820926433409));
#35419=CARTESIAN_POINT('Ctrl Pts',(0.76600483706209,1.,-1.88820926433409));
#35420=CARTESIAN_POINT('Ctrl Pts',(0.765913193856979,-1.,-1.89436577771389));
#35421=CARTESIAN_POINT('Ctrl Pts',(0.765913193856979,1.,-1.89436577771389));
#35422=CARTESIAN_POINT('Ctrl Pts',(0.765772772593395,-1.,-1.90052930393599));
#35423=CARTESIAN_POINT('Ctrl Pts',(0.765772772593395,1.,-1.90052930393599));
#35424=CARTESIAN_POINT('Ctrl Pts',(0.765584196937936,-1.,-1.90669961402362));
#35425=CARTESIAN_POINT('Ctrl Pts',(0.765584196937936,1.,-1.90669961402362));
#35426=CARTESIAN_POINT('Ctrl Pts',(0.765348465884739,-1.,-1.91287765805174));
#35427=CARTESIAN_POINT('Ctrl Pts',(0.765348465884739,1.,-1.91287765805174));
#35428=CARTESIAN_POINT('Ctrl Pts',(0.765066729667095,-1.,-1.91906491634197));
#35429=CARTESIAN_POINT('Ctrl Pts',(0.765066729667095,1.,-1.91906491634197));
#35430=CARTESIAN_POINT('Ctrl Pts',(0.764740025488189,-1.,-1.92526263537041));
#35431=CARTESIAN_POINT('Ctrl Pts',(0.764740025488189,1.,-1.92526263537041));
#35432=CARTESIAN_POINT('Ctrl Pts',(0.764369010673889,-1.,-1.93147105496367));
#35433=CARTESIAN_POINT('Ctrl Pts',(0.764369010673889,1.,-1.93147105496367));
#35434=CARTESIAN_POINT('Ctrl Pts',(0.763954049121393,-1.,-1.93768964875867));
#35435=CARTESIAN_POINT('Ctrl Pts',(0.763954049121393,1.,-1.93768964875867));
#35436=CARTESIAN_POINT('Ctrl Pts',(0.76349533353858,-1.,-1.94391746617626));
#35437=CARTESIAN_POINT('Ctrl Pts',(0.76349533353858,1.,-1.94391746617626));
#35438=CARTESIAN_POINT('Ctrl Pts',(0.762992990878774,-1.,-1.95015342590025));
#35439=CARTESIAN_POINT('Ctrl Pts',(0.762992990878774,1.,-1.95015342590025));
#35440=CARTESIAN_POINT('Ctrl Pts',(0.762447203806263,-1.,-1.95639665309893));
#35441=CARTESIAN_POINT('Ctrl Pts',(0.762447203806263,1.,-1.95639665309893));
#35442=CARTESIAN_POINT('Ctrl Pts',(0.761858300014575,-1.,-1.96264672744229));
#35443=CARTESIAN_POINT('Ctrl Pts',(0.761858300014575,1.,-1.96264672744229));
#35444=CARTESIAN_POINT('Ctrl Pts',(0.761226690483986,-1.,-1.96890351582545));
#35445=CARTESIAN_POINT('Ctrl Pts',(0.761226690483986,1.,-1.96890351582545));
#35446=CARTESIAN_POINT('Ctrl Pts',(0.760552825409855,-1.,-1.97516705321521));
#35447=CARTESIAN_POINT('Ctrl Pts',(0.760552825409855,1.,-1.97516705321521));
#35448=CARTESIAN_POINT('Ctrl Pts',(0.759837147452135,-1.,-1.98143741418156));
#35449=CARTESIAN_POINT('Ctrl Pts',(0.759837147452135,1.,-1.98143741418156));
#35450=CARTESIAN_POINT('Ctrl Pts',(0.759080037802242,-1.,-1.98771456680806));
#35451=CARTESIAN_POINT('Ctrl Pts',(0.759080037802242,1.,-1.98771456680806));
#35452=CARTESIAN_POINT('Ctrl Pts',(0.758281796766377,-1.,-1.9939983109871));
#35453=CARTESIAN_POINT('Ctrl Pts',(0.758281796766377,1.,-1.9939983109871));
#35454=CARTESIAN_POINT('Ctrl Pts',(0.757442676862341,-1.,-2.00028834739072));
#35455=CARTESIAN_POINT('Ctrl Pts',(0.757442676862341,1.,-2.00028834739072));
#35456=CARTESIAN_POINT('Ctrl Pts',(0.756562904646496,-1.,-2.00658431587682));
#35457=CARTESIAN_POINT('Ctrl Pts',(0.756562904646496,1.,-2.00658431587682));
#35458=CARTESIAN_POINT('Ctrl Pts',(0.7556427049581,-1.,-2.01288584328149));
#35459=CARTESIAN_POINT('Ctrl Pts',(0.7556427049581,1.,-2.01288584328149));
#35460=CARTESIAN_POINT('Ctrl Pts',(0.75468233072352,-1.,-2.01919259406003));
#35461=CARTESIAN_POINT('Ctrl Pts',(0.75468233072352,1.,-2.01919259406003));
#35462=CARTESIAN_POINT('Ctrl Pts',(0.753682061113765,-1.,-2.02550428623587));
#35463=CARTESIAN_POINT('Ctrl Pts',(0.753682061113765,1.,-2.02550428623587));
#35464=CARTESIAN_POINT('Ctrl Pts',(0.752642180488104,-1.,-2.03182068456467));
#35465=CARTESIAN_POINT('Ctrl Pts',(0.752642180488104,1.,-2.03182068456467));
#35466=CARTESIAN_POINT('Ctrl Pts',(0.751562963361383,-1.,-2.03814160092173));
#35467=CARTESIAN_POINT('Ctrl Pts',(0.751562963361383,1.,-2.03814160092173));
#35468=CARTESIAN_POINT('Ctrl Pts',(0.750444657874758,-1.,-2.04446689147754));
#35469=CARTESIAN_POINT('Ctrl Pts',(0.750444657874758,1.,-2.04446689147754));
#35470=CARTESIAN_POINT('Ctrl Pts',(0.749287468663053,-1.,-2.05079645591606));
#35471=CARTESIAN_POINT('Ctrl Pts',(0.749287468663053,1.,-2.05079645591606));
#35472=CARTESIAN_POINT('Ctrl Pts',(0.748091554181101,-1.,-2.05713023030263));
#35473=CARTESIAN_POINT('Ctrl Pts',(0.748091554181101,1.,-2.05713023030263));
#35474=CARTESIAN_POINT('Ctrl Pts',(0.747103932785504,-1.,-2.06220058927162));
#35475=CARTESIAN_POINT('Ctrl Pts',(0.747103932785504,1.,-2.06220058927162));
#35476=CARTESIAN_POINT('Ctrl Pts',(0.746345871542695,-1.,-2.06600523016401));
#35477=CARTESIAN_POINT('Ctrl Pts',(0.746345871542695,1.,-2.06600523016401));
#35478=CARTESIAN_POINT('Ctrl Pts',(0.74583279137781,-1.,-2.06854248895575));
#35479=CARTESIAN_POINT('Ctrl Pts',(0.74583279137781,1.,-2.06854248895575));
#35480=CARTESIAN_POINT('Ctrl Pts',(0.745574324794401,-1.,-2.0698113262342));
#35481=CARTESIAN_POINT('Ctrl Pts',(0.745574324794401,1.,-2.0698113262342));
#35482=CARTESIAN_POINT('',(0.693717979106306,1.,-1.60662857109684));
#35483=CARTESIAN_POINT('Ctrl Pts',(0.693717979106306,1.,-1.60662857109684));
#35484=CARTESIAN_POINT('Ctrl Pts',(0.695712097881194,1.,-1.61106790958151));
#35485=CARTESIAN_POINT('Ctrl Pts',(0.699605146405088,1.,-1.61974673472612));
#35486=CARTESIAN_POINT('Ctrl Pts',(0.705159151988319,1.,-1.63216541664676));
#35487=CARTESIAN_POINT('Ctrl Pts',(0.711993139355394,1.,-1.64752408832016));
#35488=CARTESIAN_POINT('Ctrl Pts',(0.719585433804282,1.,-1.6647288055568));
#35489=CARTESIAN_POINT('Ctrl Pts',(0.726235967997433,1.,-1.67996158455503));
#35490=CARTESIAN_POINT('Ctrl Pts',(0.731963238697195,1.,-1.69326921975743));
#35491=CARTESIAN_POINT('Ctrl Pts',(0.736799665724771,1.,-1.70473309006121));
#35492=CARTESIAN_POINT('Ctrl Pts',(0.740795162032087,1.,-1.71447789751927));
#35493=CARTESIAN_POINT('Ctrl Pts',(0.744021445433764,1.,-1.7226822991693));
#35494=CARTESIAN_POINT('Ctrl Pts',(0.746574710096436,1.,-1.72958533647399));
#35495=CARTESIAN_POINT('Ctrl Pts',(0.748582462954854,1.,-1.73550351679848));
#35496=CARTESIAN_POINT('Ctrl Pts',(0.75019343597954,1.,-1.74080458266705));
#35497=CARTESIAN_POINT('Ctrl Pts',(0.751555614163629,1.,-1.74585086852298));
#35498=CARTESIAN_POINT('Ctrl Pts',(0.752797683531377,1.,-1.75095139468809));
#35499=CARTESIAN_POINT('Ctrl Pts',(0.75400925402848,1.,-1.75631083600175));
#35500=CARTESIAN_POINT('Ctrl Pts',(0.755220979975262,1.,-1.7619781724032));
#35501=CARTESIAN_POINT('Ctrl Pts',(0.756421896028403,1.,-1.76789396003141));
#35502=CARTESIAN_POINT('Ctrl Pts',(0.757578264077238,1.,-1.77394167108342));
#35503=CARTESIAN_POINT('Ctrl Pts',(0.75865062667738,1.,-1.77999411220912));
#35504=CARTESIAN_POINT('Ctrl Pts',(0.759614401109868,1.,-1.78596964884527));
#35505=CARTESIAN_POINT('Ctrl Pts',(0.760469555880425,1.,-1.79185815610802));
#35506=CARTESIAN_POINT('Ctrl Pts',(0.761229695230359,1.,-1.79768986997735));
#35507=CARTESIAN_POINT('Ctrl Pts',(0.761915336443515,1.,-1.80351583877334));
#35508=CARTESIAN_POINT('Ctrl Pts',(0.762546129464036,1.,-1.80938551463989));
#35509=CARTESIAN_POINT('Ctrl Pts',(0.763132003836783,1.,-1.81532118405566));
#35510=CARTESIAN_POINT('Ctrl Pts',(0.763673465462854,1.,-1.82131873145297));
#35511=CARTESIAN_POINT('Ctrl Pts',(0.764165902606055,1.,-1.8273599120008));
#35512=CARTESIAN_POINT('Ctrl Pts',(0.764602549687845,1.,-1.8334207722714));
#35513=CARTESIAN_POINT('Ctrl Pts',(0.764978057881687,1.,-1.83948181064823));
#35514=CARTESIAN_POINT('Ctrl Pts',(0.765291664861971,1.,-1.84553698875911));
#35515=CARTESIAN_POINT('Ctrl Pts',(0.765545710619023,1.,-1.85158945130054));
#35516=CARTESIAN_POINT('Ctrl Pts',(0.765744212909305,1.,-1.85764741390391));
#35517=CARTESIAN_POINT('Ctrl Pts',(0.765891519092557,1.,-1.86372027063315));
#35518=CARTESIAN_POINT('Ctrl Pts',(0.765990708546111,1.,-1.86981398314345));
#35519=CARTESIAN_POINT('Ctrl Pts',(0.766042837036759,1.,-1.87592888967886));
#35520=CARTESIAN_POINT('Ctrl Pts',(0.766047794851868,1.,-1.88206215302561));
#35521=CARTESIAN_POINT('Ctrl Pts',(0.76600483706209,1.,-1.88820926433409));
#35522=CARTESIAN_POINT('Ctrl Pts',(0.765913193856979,1.,-1.89436577771389));
#35523=CARTESIAN_POINT('Ctrl Pts',(0.765772772593395,1.,-1.90052930393599));
#35524=CARTESIAN_POINT('Ctrl Pts',(0.765584196937936,1.,-1.90669961402362));
#35525=CARTESIAN_POINT('Ctrl Pts',(0.765348465884739,1.,-1.91287765805174));
#35526=CARTESIAN_POINT('Ctrl Pts',(0.765066729667095,1.,-1.91906491634197));
#35527=CARTESIAN_POINT('Ctrl Pts',(0.764740025488189,1.,-1.92526263537041));
#35528=CARTESIAN_POINT('Ctrl Pts',(0.764369010673889,1.,-1.93147105496367));
#35529=CARTESIAN_POINT('Ctrl Pts',(0.763954049121393,1.,-1.93768964875867));
#35530=CARTESIAN_POINT('Ctrl Pts',(0.76349533353858,1.,-1.94391746617626));
#35531=CARTESIAN_POINT('Ctrl Pts',(0.762992990878774,1.,-1.95015342590025));
#35532=CARTESIAN_POINT('Ctrl Pts',(0.762447203806263,1.,-1.95639665309893));
#35533=CARTESIAN_POINT('Ctrl Pts',(0.761858300014575,1.,-1.96264672744229));
#35534=CARTESIAN_POINT('Ctrl Pts',(0.761226690483986,1.,-1.96890351582545));
#35535=CARTESIAN_POINT('Ctrl Pts',(0.760552825409855,1.,-1.97516705321521));
#35536=CARTESIAN_POINT('Ctrl Pts',(0.759837147452135,1.,-1.98143741418156));
#35537=CARTESIAN_POINT('Ctrl Pts',(0.759080037802242,1.,-1.98771456680806));
#35538=CARTESIAN_POINT('Ctrl Pts',(0.758281796766377,1.,-1.9939983109871));
#35539=CARTESIAN_POINT('Ctrl Pts',(0.757442676862341,1.,-2.00028834739072));
#35540=CARTESIAN_POINT('Ctrl Pts',(0.756562904646496,1.,-2.00658431587682));
#35541=CARTESIAN_POINT('Ctrl Pts',(0.7556427049581,1.,-2.01288584328149));
#35542=CARTESIAN_POINT('Ctrl Pts',(0.75468233072352,1.,-2.01919259406003));
#35543=CARTESIAN_POINT('Ctrl Pts',(0.753682061113765,1.,-2.02550428623587));
#35544=CARTESIAN_POINT('Ctrl Pts',(0.752642180488104,1.,-2.03182068456467));
#35545=CARTESIAN_POINT('Ctrl Pts',(0.751562963361383,1.,-2.03814160092173));
#35546=CARTESIAN_POINT('Ctrl Pts',(0.750444657874758,1.,-2.04446689147754));
#35547=CARTESIAN_POINT('Ctrl Pts',(0.749287468663053,1.,-2.05079645591606));
#35548=CARTESIAN_POINT('Ctrl Pts',(0.748091554181101,1.,-2.05713023030263));
#35549=CARTESIAN_POINT('Ctrl Pts',(0.747103932785504,1.,-2.06220058927162));
#35550=CARTESIAN_POINT('Ctrl Pts',(0.746345871542695,1.,-2.06600523016401));
#35551=CARTESIAN_POINT('Ctrl Pts',(0.74583279137781,1.,-2.06854248895575));
#35552=CARTESIAN_POINT('Ctrl Pts',(0.745574324794401,1.,-2.0698113262342));
#35553=CARTESIAN_POINT('',(0.693717979106306,0.,-1.60662857109684));
#35554=CARTESIAN_POINT('Origin',(0.,0.,0.));
#35555=CARTESIAN_POINT('',(0.892032620296855,1.,-1.5055822144029));
#35556=CARTESIAN_POINT('Origin',(0.,1.,0.));
#35557=CARTESIAN_POINT('',(0.892032620296855,0.,-1.5055822144029));
#35558=CARTESIAN_POINT('Ctrl Pts',(1.23627494547115,-1.,-1.81978687191668));
#35559=CARTESIAN_POINT('Ctrl Pts',(1.23627494547115,1.,-1.81978687191668));
#35560=CARTESIAN_POINT('Ctrl Pts',(1.23509651170476,-1.,-1.81925017193666));
#35561=CARTESIAN_POINT('Ctrl Pts',(1.23509651170476,1.,-1.81925017193666));
#35562=CARTESIAN_POINT('Ctrl Pts',(1.2327422452705,-1.,-1.81817389921279));
#35563=CARTESIAN_POINT('Ctrl Pts',(1.2327422452705,1.,-1.81817389921279));
#35564=CARTESIAN_POINT('Ctrl Pts',(1.2292186489137,-1.,-1.8165508718364));
#35565=CARTESIAN_POINT('Ctrl Pts',(1.2292186489137,1.,-1.8165508718364));
#35566=CARTESIAN_POINT('Ctrl Pts',(1.2245361330495,-1.,-1.81436959210434));
#35567=CARTESIAN_POINT('Ctrl Pts',(1.2245361330495,1.,-1.81436959210434));
#35568=CARTESIAN_POINT('Ctrl Pts',(1.21870906103557,-1.,-1.81161420806656));
#35569=CARTESIAN_POINT('Ctrl Pts',(1.21870906103557,1.,-1.81161420806656));
#35570=CARTESIAN_POINT('Ctrl Pts',(1.21290815708314,-1.,-1.80882996917129));
#35571=CARTESIAN_POINT('Ctrl Pts',(1.21290815708314,1.,-1.80882996917129));
#35572=CARTESIAN_POINT('Ctrl Pts',(1.20713356605475,-1.,-1.80601678480707));
#35573=CARTESIAN_POINT('Ctrl Pts',(1.20713356605475,1.,-1.80601678480707));
#35574=CARTESIAN_POINT('Ctrl Pts',(1.20138548938974,-1.,-1.80317454838603));
#35575=CARTESIAN_POINT('Ctrl Pts',(1.20138548938974,1.,-1.80317454838603));
#35576=CARTESIAN_POINT('Ctrl Pts',(1.19566418930242,-1.,-1.80030314369879));
#35577=CARTESIAN_POINT('Ctrl Pts',(1.19566418930242,1.,-1.80030314369879));
#35578=CARTESIAN_POINT('Ctrl Pts',(1.18996997934445,-1.,-1.79740245923478));
#35579=CARTESIAN_POINT('Ctrl Pts',(1.18996997934445,1.,-1.79740245923478));
#35580=CARTESIAN_POINT('Ctrl Pts',(1.18430321697432,-1.,-1.79447240321515));
#35581=CARTESIAN_POINT('Ctrl Pts',(1.18430321697432,1.,-1.79447240321515));
#35582=CARTESIAN_POINT('Ctrl Pts',(1.17866429440809,-1.,-1.79151291552689));
#35583=CARTESIAN_POINT('Ctrl Pts',(1.17866429440809,1.,-1.79151291552689));
#35584=CARTESIAN_POINT('Ctrl Pts',(1.17305363177328,-1.,-1.78852398877617));
#35585=CARTESIAN_POINT('Ctrl Pts',(1.17305363177328,1.,-1.78852398877617));
#35586=CARTESIAN_POINT('Ctrl Pts',(1.16747166312303,-1.,-1.78550566040443));
#35587=CARTESIAN_POINT('Ctrl Pts',(1.16747166312303,1.,-1.78550566040443));
#35588=CARTESIAN_POINT('Ctrl Pts',(1.16191881298499,-1.,-1.78245795881009));
#35589=CARTESIAN_POINT('Ctrl Pts',(1.16191881298499,1.,-1.78245795881009));
#35590=CARTESIAN_POINT('Ctrl Pts',(1.15639547194698,-1.,-1.77938085564275));
#35591=CARTESIAN_POINT('Ctrl Pts',(1.15639547194698,1.,-1.77938085564275));
#35592=CARTESIAN_POINT('Ctrl Pts',(1.15090197841514,-1.,-1.7762742255701));
#35593=CARTESIAN_POINT('Ctrl Pts',(1.15090197841514,1.,-1.7762742255701));
#35594=CARTESIAN_POINT('Ctrl Pts',(1.1454385822692,-1.,-1.77313777896194));
#35595=CARTESIAN_POINT('Ctrl Pts',(1.1454385822692,1.,-1.77313777896194));
#35596=CARTESIAN_POINT('Ctrl Pts',(1.14000548336975,-1.,-1.76997111386769));
#35597=CARTESIAN_POINT('Ctrl Pts',(1.14000548336975,1.,-1.76997111386769));
#35598=CARTESIAN_POINT('Ctrl Pts',(1.1346029180462,-1.,-1.76677384551862));
#35599=CARTESIAN_POINT('Ctrl Pts',(1.1346029180462,1.,-1.76677384551862));
#35600=CARTESIAN_POINT('Ctrl Pts',(1.12923123555075,-1.,-1.7635457196617));
#35601=CARTESIAN_POINT('Ctrl Pts',(1.12923123555075,1.,-1.7635457196617));
#35602=CARTESIAN_POINT('Ctrl Pts',(1.12389096855086,-1.,-1.76028671825096));
#35603=CARTESIAN_POINT('Ctrl Pts',(1.12389096855086,1.,-1.76028671825096));
#35604=CARTESIAN_POINT('Ctrl Pts',(1.11858293216763,-1.,-1.75699720772105));
#35605=CARTESIAN_POINT('Ctrl Pts',(1.11858293216763,1.,-1.75699720772105));
#35606=CARTESIAN_POINT('Ctrl Pts',(1.11330807582551,-1.,-1.7536777209463));
#35607=CARTESIAN_POINT('Ctrl Pts',(1.11330807582551,1.,-1.7536777209463));
#35608=CARTESIAN_POINT('Ctrl Pts',(1.10806728183007,-1.,-1.7503286607592));
#35609=CARTESIAN_POINT('Ctrl Pts',(1.10806728183007,1.,-1.7503286607592));
#35610=CARTESIAN_POINT('Ctrl Pts',(1.10286118991143,-1.,-1.74695004214923));
#35611=CARTESIAN_POINT('Ctrl Pts',(1.10286118991143,1.,-1.74695004214923));
#35612=CARTESIAN_POINT('Ctrl Pts',(1.09768999241225,-1.,-1.74354119236208));
#35613=CARTESIAN_POINT('Ctrl Pts',(1.09768999241225,1.,-1.74354119236208));
#35614=CARTESIAN_POINT('Ctrl Pts',(1.09255329056493,-1.,-1.74010053962247));
#35615=CARTESIAN_POINT('Ctrl Pts',(1.09255329056493,1.,-1.74010053962247));
#35616=CARTESIAN_POINT('Ctrl Pts',(1.08745056285427,-1.,-1.73662628326091));
#35617=CARTESIAN_POINT('Ctrl Pts',(1.08745056285427,1.,-1.73662628326091));
#35618=CARTESIAN_POINT('Ctrl Pts',(1.08238162784749,-1.,-1.73311705663407));
#35619=CARTESIAN_POINT('Ctrl Pts',(1.08238162784749,1.,-1.73311705663407));
#35620=CARTESIAN_POINT('Ctrl Pts',(1.0773470373727,-1.,-1.72957248977424));
#35621=CARTESIAN_POINT('Ctrl Pts',(1.0773470373727,1.,-1.72957248977424));
#35622=CARTESIAN_POINT('Ctrl Pts',(1.07234866990252,-1.,-1.72599406198488));
#35623=CARTESIAN_POINT('Ctrl Pts',(1.07234866990252,1.,-1.72599406198488));
#35624=CARTESIAN_POINT('Ctrl Pts',(1.06738966975462,-1.,-1.72238500928453));
#35625=CARTESIAN_POINT('Ctrl Pts',(1.06738966975462,1.,-1.72238500928453));
#35626=CARTESIAN_POINT('Ctrl Pts',(1.06247324680647,-1.,-1.71874858456904));
#35627=CARTESIAN_POINT('Ctrl Pts',(1.06247324680647,1.,-1.71874858456904));
#35628=CARTESIAN_POINT('Ctrl Pts',(1.05760163192479,-1.,-1.7150865442702));
#35629=CARTESIAN_POINT('Ctrl Pts',(1.05760163192479,1.,-1.7150865442702));
#35630=CARTESIAN_POINT('Ctrl Pts',(1.05277517202855,-1.,-1.71139783543989));
#35631=CARTESIAN_POINT('Ctrl Pts',(1.05277517202855,1.,-1.71139783543989));
#35632=CARTESIAN_POINT('Ctrl Pts',(1.04799085404995,-1.,-1.70767646263649));
#35633=CARTESIAN_POINT('Ctrl Pts',(1.04799085404995,1.,-1.70767646263649));
#35634=CARTESIAN_POINT('Ctrl Pts',(1.04324363334554,-1.,-1.70391338707982));
#35635=CARTESIAN_POINT('Ctrl Pts',(1.04324363334554,1.,-1.70391338707982));
#35636=CARTESIAN_POINT('Ctrl Pts',(1.03852922490789,-1.,-1.70010052930962));
#35637=CARTESIAN_POINT('Ctrl Pts',(1.03852922490789,1.,-1.70010052930962));
#35638=CARTESIAN_POINT('Ctrl Pts',(1.03384646003588,-1.,-1.69623414782771));
#35639=CARTESIAN_POINT('Ctrl Pts',(1.03384646003588,1.,-1.69623414782771));
#35640=CARTESIAN_POINT('Ctrl Pts',(1.02919977579147,-1.,-1.69231840863458));
#35641=CARTESIAN_POINT('Ctrl Pts',(1.02919977579147,1.,-1.69231840863458));
#35642=CARTESIAN_POINT('Ctrl Pts',(1.02460180535255,-1.,-1.68836910178447));
#35643=CARTESIAN_POINT('Ctrl Pts',(1.02460180535255,1.,-1.68836910178447));
#35644=CARTESIAN_POINT('Ctrl Pts',(1.02006795074201,-1.,-1.68440578021706));
#35645=CARTESIAN_POINT('Ctrl Pts',(1.02006795074201,1.,-1.68440578021706));
#35646=CARTESIAN_POINT('Ctrl Pts',(1.01561026162773,-1.,-1.68044289894798));
#35647=CARTESIAN_POINT('Ctrl Pts',(1.01561026162773,1.,-1.68044289894798));
#35648=CARTESIAN_POINT('Ctrl Pts',(1.01123236493511,-1.,-1.67648246776464));
#35649=CARTESIAN_POINT('Ctrl Pts',(1.01123236493511,1.,-1.67648246776464));
#35650=CARTESIAN_POINT('Ctrl Pts',(1.00692206696414,-1.,-1.67250335383293));
#35651=CARTESIAN_POINT('Ctrl Pts',(1.00692206696414,1.,-1.67250335383293));
#35652=CARTESIAN_POINT('Ctrl Pts',(1.00265091003727,-1.,-1.66846059277303));
#35653=CARTESIAN_POINT('Ctrl Pts',(1.00265091003727,1.,-1.66846059277303));
#35654=CARTESIAN_POINT('Ctrl Pts',(0.998389654952757,-1.,-1.66430758030376));
#35655=CARTESIAN_POINT('Ctrl Pts',(0.998389654952757,1.,-1.66430758030376));
#35656=CARTESIAN_POINT('Ctrl Pts',(0.994121836661305,-1.,-1.66001553809947));
#35657=CARTESIAN_POINT('Ctrl Pts',(0.994121836661305,1.,-1.66001553809947));
#35658=CARTESIAN_POINT('Ctrl Pts',(0.989855627854164,-1.,-1.65559044289699));
#35659=CARTESIAN_POINT('Ctrl Pts',(0.989855627854164,1.,-1.65559044289699));
#35660=CARTESIAN_POINT('Ctrl Pts',(0.98564262292082,-1.,-1.65110016612638));
#35661=CARTESIAN_POINT('Ctrl Pts',(0.98564262292082,1.,-1.65110016612638));
#35662=CARTESIAN_POINT('Ctrl Pts',(0.981562530939489,-1.,-1.64665139190656));
#35663=CARTESIAN_POINT('Ctrl Pts',(0.981562530939489,1.,-1.64665139190656));
#35664=CARTESIAN_POINT('Ctrl Pts',(0.977689794119416,-1.,-1.64233990826687));
#35665=CARTESIAN_POINT('Ctrl Pts',(0.977689794119416,1.,-1.64233990826687));
#35666=CARTESIAN_POINT('Ctrl Pts',(0.974066058287418,-1.,-1.63820952658144));
#35667=CARTESIAN_POINT('Ctrl Pts',(0.974066058287418,1.,-1.63820952658144));
#35668=CARTESIAN_POINT('Ctrl Pts',(0.970669715997509,-1.,-1.63420665729798));
#35669=CARTESIAN_POINT('Ctrl Pts',(0.970669715997509,1.,-1.63420665729798));
#35670=CARTESIAN_POINT('Ctrl Pts',(0.967387853230345,-1.,-1.63013849959462));
#35671=CARTESIAN_POINT('Ctrl Pts',(0.967387853230345,1.,-1.63013849959462));
#35672=CARTESIAN_POINT('Ctrl Pts',(0.964046107040535,-1.,-1.62571930670187));
#35673=CARTESIAN_POINT('Ctrl Pts',(0.964046107040535,1.,-1.62571930670187));
#35674=CARTESIAN_POINT('Ctrl Pts',(0.960438326101728,-1.,-1.62061638140221));
#35675=CARTESIAN_POINT('Ctrl Pts',(0.960438326101728,1.,-1.62061638140221));
#35676=CARTESIAN_POINT('Ctrl Pts',(0.95635442292067,-1.,-1.61449324337085));
#35677=CARTESIAN_POINT('Ctrl Pts',(0.95635442292067,1.,-1.61449324337085));
#35678=CARTESIAN_POINT('Ctrl Pts',(0.951613284356035,-1.,-1.60706069896936));
#35679=CARTESIAN_POINT('Ctrl Pts',(0.951613284356035,1.,-1.60706069896936));
#35680=CARTESIAN_POINT('Ctrl Pts',(0.946078063315257,-1.,-1.59810042043673));
#35681=CARTESIAN_POINT('Ctrl Pts',(0.946078063315257,1.,-1.59810042043673));
#35682=CARTESIAN_POINT('Ctrl Pts',(0.939646377893399,-1.,-1.58744937487176));
#35683=CARTESIAN_POINT('Ctrl Pts',(0.939646377893399,1.,-1.58744937487176));
#35684=CARTESIAN_POINT('Ctrl Pts',(0.932246680108685,-1.,-1.57499388382243));
#35685=CARTESIAN_POINT('Ctrl Pts',(0.932246680108685,1.,-1.57499388382243));
#35686=CARTESIAN_POINT('Ctrl Pts',(0.923832188944341,-1.,-1.56065988578893));
#35687=CARTESIAN_POINT('Ctrl Pts',(0.923832188944341,1.,-1.56065988578893));
#35688=CARTESIAN_POINT('Ctrl Pts',(0.914375919026456,-1.,-1.54440491149498));
#35689=CARTESIAN_POINT('Ctrl Pts',(0.914375919026456,1.,-1.54440491149498));
#35690=CARTESIAN_POINT('Ctrl Pts',(0.905967409625651,-1.,-1.52984849887993));
#35691=CARTESIAN_POINT('Ctrl Pts',(0.905967409625651,1.,-1.52984849887993));
#35692=CARTESIAN_POINT('Ctrl Pts',(0.89918504748351,-1.,-1.51805569590094));
#35693=CARTESIAN_POINT('Ctrl Pts',(0.89918504748351,1.,-1.51805569590094));
#35694=CARTESIAN_POINT('Ctrl Pts',(0.894452006964543,-1.,-1.50980486806688));
#35695=CARTESIAN_POINT('Ctrl Pts',(0.894452006964543,1.,-1.50980486806688));
#35696=CARTESIAN_POINT('Ctrl Pts',(0.892032620296855,-1.,-1.5055822144029));
#35697=CARTESIAN_POINT('Ctrl Pts',(0.892032620296855,1.,-1.5055822144029));
#35698=CARTESIAN_POINT('',(1.23627494547115,1.,-1.81978687191668));
#35699=CARTESIAN_POINT('Ctrl Pts',(1.23627494547115,1.,-1.81978687191668));
#35700=CARTESIAN_POINT('Ctrl Pts',(1.23509651170476,1.,-1.81925017193666));
#35701=CARTESIAN_POINT('Ctrl Pts',(1.2327422452705,1.,-1.81817389921279));
#35702=CARTESIAN_POINT('Ctrl Pts',(1.2292186489137,1.,-1.8165508718364));
#35703=CARTESIAN_POINT('Ctrl Pts',(1.2245361330495,1.,-1.81436959210434));
#35704=CARTESIAN_POINT('Ctrl Pts',(1.21870906103557,1.,-1.81161420806656));
#35705=CARTESIAN_POINT('Ctrl Pts',(1.21290815708314,1.,-1.80882996917129));
#35706=CARTESIAN_POINT('Ctrl Pts',(1.20713356605475,1.,-1.80601678480707));
#35707=CARTESIAN_POINT('Ctrl Pts',(1.20138548938974,1.,-1.80317454838603));
#35708=CARTESIAN_POINT('Ctrl Pts',(1.19566418930242,1.,-1.80030314369879));
#35709=CARTESIAN_POINT('Ctrl Pts',(1.18996997934445,1.,-1.79740245923478));
#35710=CARTESIAN_POINT('Ctrl Pts',(1.18430321697432,1.,-1.79447240321515));
#35711=CARTESIAN_POINT('Ctrl Pts',(1.17866429440809,1.,-1.79151291552689));
#35712=CARTESIAN_POINT('Ctrl Pts',(1.17305363177328,1.,-1.78852398877617));
#35713=CARTESIAN_POINT('Ctrl Pts',(1.16747166312303,1.,-1.78550566040443));
#35714=CARTESIAN_POINT('Ctrl Pts',(1.16191881298499,1.,-1.78245795881009));
#35715=CARTESIAN_POINT('Ctrl Pts',(1.15639547194698,1.,-1.77938085564275));
#35716=CARTESIAN_POINT('Ctrl Pts',(1.15090197841514,1.,-1.7762742255701));
#35717=CARTESIAN_POINT('Ctrl Pts',(1.1454385822692,1.,-1.77313777896194));
#35718=CARTESIAN_POINT('Ctrl Pts',(1.14000548336975,1.,-1.76997111386769));
#35719=CARTESIAN_POINT('Ctrl Pts',(1.1346029180462,1.,-1.76677384551862));
#35720=CARTESIAN_POINT('Ctrl Pts',(1.12923123555075,1.,-1.7635457196617));
#35721=CARTESIAN_POINT('Ctrl Pts',(1.12389096855086,1.,-1.76028671825096));
#35722=CARTESIAN_POINT('Ctrl Pts',(1.11858293216763,1.,-1.75699720772105));
#35723=CARTESIAN_POINT('Ctrl Pts',(1.11330807582551,1.,-1.7536777209463));
#35724=CARTESIAN_POINT('Ctrl Pts',(1.10806728183007,1.,-1.7503286607592));
#35725=CARTESIAN_POINT('Ctrl Pts',(1.10286118991143,1.,-1.74695004214923));
#35726=CARTESIAN_POINT('Ctrl Pts',(1.09768999241225,1.,-1.74354119236208));
#35727=CARTESIAN_POINT('Ctrl Pts',(1.09255329056493,1.,-1.74010053962247));
#35728=CARTESIAN_POINT('Ctrl Pts',(1.08745056285427,1.,-1.73662628326091));
#35729=CARTESIAN_POINT('Ctrl Pts',(1.08238162784749,1.,-1.73311705663407));
#35730=CARTESIAN_POINT('Ctrl Pts',(1.0773470373727,1.,-1.72957248977424));
#35731=CARTESIAN_POINT('Ctrl Pts',(1.07234866990252,1.,-1.72599406198488));
#35732=CARTESIAN_POINT('Ctrl Pts',(1.06738966975462,1.,-1.72238500928453));
#35733=CARTESIAN_POINT('Ctrl Pts',(1.06247324680647,1.,-1.71874858456904));
#35734=CARTESIAN_POINT('Ctrl Pts',(1.05760163192479,1.,-1.7150865442702));
#35735=CARTESIAN_POINT('Ctrl Pts',(1.05277517202855,1.,-1.71139783543989));
#35736=CARTESIAN_POINT('Ctrl Pts',(1.04799085404995,1.,-1.70767646263649));
#35737=CARTESIAN_POINT('Ctrl Pts',(1.04324363334554,1.,-1.70391338707982));
#35738=CARTESIAN_POINT('Ctrl Pts',(1.03852922490789,1.,-1.70010052930962));
#35739=CARTESIAN_POINT('Ctrl Pts',(1.03384646003588,1.,-1.69623414782771));
#35740=CARTESIAN_POINT('Ctrl Pts',(1.02919977579147,1.,-1.69231840863458));
#35741=CARTESIAN_POINT('Ctrl Pts',(1.02460180535255,1.,-1.68836910178447));
#35742=CARTESIAN_POINT('Ctrl Pts',(1.02006795074201,1.,-1.68440578021706));
#35743=CARTESIAN_POINT('Ctrl Pts',(1.01561026162773,1.,-1.68044289894798));
#35744=CARTESIAN_POINT('Ctrl Pts',(1.01123236493511,1.,-1.67648246776464));
#35745=CARTESIAN_POINT('Ctrl Pts',(1.00692206696414,1.,-1.67250335383293));
#35746=CARTESIAN_POINT('Ctrl Pts',(1.00265091003727,1.,-1.66846059277303));
#35747=CARTESIAN_POINT('Ctrl Pts',(0.998389654952757,1.,-1.66430758030376));
#35748=CARTESIAN_POINT('Ctrl Pts',(0.994121836661305,1.,-1.66001553809947));
#35749=CARTESIAN_POINT('Ctrl Pts',(0.989855627854164,1.,-1.65559044289699));
#35750=CARTESIAN_POINT('Ctrl Pts',(0.98564262292082,1.,-1.65110016612638));
#35751=CARTESIAN_POINT('Ctrl Pts',(0.981562530939489,1.,-1.64665139190656));
#35752=CARTESIAN_POINT('Ctrl Pts',(0.977689794119416,1.,-1.64233990826687));
#35753=CARTESIAN_POINT('Ctrl Pts',(0.974066058287418,1.,-1.63820952658144));
#35754=CARTESIAN_POINT('Ctrl Pts',(0.970669715997509,1.,-1.63420665729798));
#35755=CARTESIAN_POINT('Ctrl Pts',(0.967387853230345,1.,-1.63013849959462));
#35756=CARTESIAN_POINT('Ctrl Pts',(0.964046107040535,1.,-1.62571930670187));
#35757=CARTESIAN_POINT('Ctrl Pts',(0.960438326101728,1.,-1.62061638140221));
#35758=CARTESIAN_POINT('Ctrl Pts',(0.95635442292067,1.,-1.61449324337085));
#35759=CARTESIAN_POINT('Ctrl Pts',(0.951613284356035,1.,-1.60706069896936));
#35760=CARTESIAN_POINT('Ctrl Pts',(0.946078063315257,1.,-1.59810042043673));
#35761=CARTESIAN_POINT('Ctrl Pts',(0.939646377893399,1.,-1.58744937487176));
#35762=CARTESIAN_POINT('Ctrl Pts',(0.932246680108685,1.,-1.57499388382243));
#35763=CARTESIAN_POINT('Ctrl Pts',(0.923832188944341,1.,-1.56065988578893));
#35764=CARTESIAN_POINT('Ctrl Pts',(0.914375919026456,1.,-1.54440491149498));
#35765=CARTESIAN_POINT('Ctrl Pts',(0.905967409625651,1.,-1.52984849887993));
#35766=CARTESIAN_POINT('Ctrl Pts',(0.89918504748351,1.,-1.51805569590094));
#35767=CARTESIAN_POINT('Ctrl Pts',(0.894452006964543,1.,-1.50980486806688));
#35768=CARTESIAN_POINT('Ctrl Pts',(0.892032620296855,1.,-1.5055822144029));
#35769=CARTESIAN_POINT('',(1.23627494547115,0.,-1.81978687191668));
#35770=CARTESIAN_POINT('Origin',(1.34869019493419,0.,-1.73811241238545));
#35771=CARTESIAN_POINT('',(1.34869019493419,1.,-1.73811241238545));
#35772=CARTESIAN_POINT('',(1.23627494547115,1.,-1.81978687191668));
#35773=CARTESIAN_POINT('',(1.34869019493419,0.,-1.73811241238545));
#35774=CARTESIAN_POINT('Ctrl Pts',(1.15624053661742,-1.,-1.31362392696032));
#35775=CARTESIAN_POINT('Ctrl Pts',(1.15624053661742,1.,-1.31362392696032));
#35776=CARTESIAN_POINT('Ctrl Pts',(1.15950888730809,-1.,-1.31722977216397));
#35777=CARTESIAN_POINT('Ctrl Pts',(1.15950888730809,1.,-1.31722977216397));
#35778=CARTESIAN_POINT('Ctrl Pts',(1.16589330093588,-1.,-1.32428080721772));
#35779=CARTESIAN_POINT('Ctrl Pts',(1.16589330093588,1.,-1.32428080721772));
#35780=CARTESIAN_POINT('Ctrl Pts',(1.17501305789857,-1.,-1.33437539347008));
#35781=CARTESIAN_POINT('Ctrl Pts',(1.17501305789857,1.,-1.33437539347008));
#35782=CARTESIAN_POINT('Ctrl Pts',(1.18625865667441,-1.,-1.34687054001093));
#35783=CARTESIAN_POINT('Ctrl Pts',(1.18625865667441,1.,-1.34687054001093));
#35784=CARTESIAN_POINT('Ctrl Pts',(1.1987959077932,-1.,-1.36088705043885));
#35785=CARTESIAN_POINT('Ctrl Pts',(1.1987959077932,1.,-1.36088705043885));
#35786=CARTESIAN_POINT('Ctrl Pts',(1.20982812925645,-1.,-1.37331915607905));
#35787=CARTESIAN_POINT('Ctrl Pts',(1.20982812925645,1.,-1.37331915607905));
#35788=CARTESIAN_POINT('Ctrl Pts',(1.21938737280852,-1.,-1.38420564527715));
#35789=CARTESIAN_POINT('Ctrl Pts',(1.21938737280852,1.,-1.38420564527715));
#35790=CARTESIAN_POINT('Ctrl Pts',(1.22752961899387,-1.,-1.39361389568796));
#35791=CARTESIAN_POINT('Ctrl Pts',(1.22752961899387,1.,-1.39361389568796));
#35792=CARTESIAN_POINT('Ctrl Pts',(1.23434087290423,-1.,-1.40164708206106));
#35793=CARTESIAN_POINT('Ctrl Pts',(1.23434087290423,1.,-1.40164708206106));
#35794=CARTESIAN_POINT('Ctrl Pts',(1.23994455029534,-1.,-1.40845295531283));
#35795=CARTESIAN_POINT('Ctrl Pts',(1.23994455029534,1.,-1.40845295531283));
#35796=CARTESIAN_POINT('Ctrl Pts',(1.24450600513056,-1.,-1.41422913175179));
#35797=CARTESIAN_POINT('Ctrl Pts',(1.24450600513056,1.,-1.41422913175179));
#35798=CARTESIAN_POINT('Ctrl Pts',(1.24824430986571,-1.,-1.41923722596025));
#35799=CARTESIAN_POINT('Ctrl Pts',(1.24824430986571,1.,-1.41923722596025));
#35800=CARTESIAN_POINT('Ctrl Pts',(1.2514145557001,-1.,-1.42378102115575));
#35801=CARTESIAN_POINT('Ctrl Pts',(1.2514145557001,1.,-1.42378102115575));
#35802=CARTESIAN_POINT('Ctrl Pts',(1.25426945222639,-1.,-1.42815938799387));
#35803=CARTESIAN_POINT('Ctrl Pts',(1.25426945222639,1.,-1.42815938799387));
#35804=CARTESIAN_POINT('Ctrl Pts',(1.25702687965755,-1.,-1.43262645609691));
#35805=CARTESIAN_POINT('Ctrl Pts',(1.25702687965755,1.,-1.43262645609691));
#35806=CARTESIAN_POINT('Ctrl Pts',(1.25983531012005,-1.,-1.43734919180848));
#35807=CARTESIAN_POINT('Ctrl Pts',(1.25983531012005,1.,-1.43734919180848));
#35808=CARTESIAN_POINT('Ctrl Pts',(1.26273903323858,-1.,-1.44236470511303));
#35809=CARTESIAN_POINT('Ctrl Pts',(1.26273903323858,1.,-1.44236470511303));
#35810=CARTESIAN_POINT('Ctrl Pts',(1.26570925118868,-1.,-1.44761985001662));
#35811=CARTESIAN_POINT('Ctrl Pts',(1.26570925118868,1.,-1.44761985001662));
#35812=CARTESIAN_POINT('Ctrl Pts',(1.2686778680489,-1.,-1.45301422764247));
#35813=CARTESIAN_POINT('Ctrl Pts',(1.2686778680489,1.,-1.45301422764247));
#35814=CARTESIAN_POINT('Ctrl Pts',(1.27156805265289,-1.,-1.45843906294697));
#35815=CARTESIAN_POINT('Ctrl Pts',(1.27156805265289,1.,-1.45843906294697));
#35816=CARTESIAN_POINT('Ctrl Pts',(1.27433119897822,-1.,-1.46382431332476));
#35817=CARTESIAN_POINT('Ctrl Pts',(1.27433119897822,1.,-1.46382431332476));
#35818=CARTESIAN_POINT('Ctrl Pts',(1.27696414831089,-1.,-1.46916035917133));
#35819=CARTESIAN_POINT('Ctrl Pts',(1.27696414831089,1.,-1.46916035917133));
#35820=CARTESIAN_POINT('Ctrl Pts',(1.2794891824849,-1.,-1.4744717526707));
#35821=CARTESIAN_POINT('Ctrl Pts',(1.2794891824849,1.,-1.4744717526707));
#35822=CARTESIAN_POINT('Ctrl Pts',(1.28194158939517,-1.,-1.47980070347096));
#35823=CARTESIAN_POINT('Ctrl Pts',(1.28194158939517,1.,-1.47980070347096));
#35824=CARTESIAN_POINT('Ctrl Pts',(1.28435533880201,-1.,-1.4851881711891));
#35825=CARTESIAN_POINT('Ctrl Pts',(1.28435533880201,1.,-1.4851881711891));
#35826=CARTESIAN_POINT('Ctrl Pts',(1.2867467611644,-1.,-1.4906522831278));
#35827=CARTESIAN_POINT('Ctrl Pts',(1.2867467611644,1.,-1.4906522831278));
#35828=CARTESIAN_POINT('Ctrl Pts',(1.28911506584254,-1.,-1.49618896881754));
#35829=CARTESIAN_POINT('Ctrl Pts',(1.28911506584254,1.,-1.49618896881754));
#35830=CARTESIAN_POINT('Ctrl Pts',(1.29145022885181,-1.,-1.50178230149776));
#35831=CARTESIAN_POINT('Ctrl Pts',(1.29145022885181,1.,-1.50178230149776));
#35832=CARTESIAN_POINT('Ctrl Pts',(1.29373841372842,-1.,-1.50741159078365));
#35833=CARTESIAN_POINT('Ctrl Pts',(1.29373841372842,1.,-1.50741159078365));
#35834=CARTESIAN_POINT('Ctrl Pts',(1.29596850710509,-1.,-1.51305994241402));
#35835=CARTESIAN_POINT('Ctrl Pts',(1.29596850710509,1.,-1.51305994241402));
#35836=CARTESIAN_POINT('Ctrl Pts',(1.29813791800747,-1.,-1.51872184912724));
#35837=CARTESIAN_POINT('Ctrl Pts',(1.29813791800747,1.,-1.51872184912724));
#35838=CARTESIAN_POINT('Ctrl Pts',(1.30024984366328,-1.,-1.52439957861062));
#35839=CARTESIAN_POINT('Ctrl Pts',(1.30024984366328,1.,-1.52439957861062));
#35840=CARTESIAN_POINT('Ctrl Pts',(1.30231064395568,-1.,-1.53009970283891));
#35841=CARTESIAN_POINT('Ctrl Pts',(1.30231064395568,1.,-1.53009970283891));
#35842=CARTESIAN_POINT('Ctrl Pts',(1.30432735639489,-1.,-1.53582981268977));
#35843=CARTESIAN_POINT('Ctrl Pts',(1.30432735639489,1.,-1.53582981268977));
#35844=CARTESIAN_POINT('Ctrl Pts',(1.30630475189556,-1.,-1.54159462645432));
#35845=CARTESIAN_POINT('Ctrl Pts',(1.30630475189556,1.,-1.54159462645432));
#35846=CARTESIAN_POINT('Ctrl Pts',(1.30824393907473,-1.,-1.54739413957185));
#35847=CARTESIAN_POINT('Ctrl Pts',(1.30824393907473,1.,-1.54739413957185));
#35848=CARTESIAN_POINT('Ctrl Pts',(1.31014393684222,-1.,-1.55322568759481));
#35849=CARTESIAN_POINT('Ctrl Pts',(1.31014393684222,1.,-1.55322568759481));
#35850=CARTESIAN_POINT('Ctrl Pts',(1.31200264341696,-1.,-1.55908521254821));
#35851=CARTESIAN_POINT('Ctrl Pts',(1.31200264341696,1.,-1.55908521254821));
#35852=CARTESIAN_POINT('Ctrl Pts',(1.31381795281002,-1.,-1.56496872402353));
#35853=CARTESIAN_POINT('Ctrl Pts',(1.31381795281002,1.,-1.56496872402353));
#35854=CARTESIAN_POINT('Ctrl Pts',(1.31558903860016,-1.,-1.57087397835723));
#35855=CARTESIAN_POINT('Ctrl Pts',(1.31558903860016,1.,-1.57087397835723));
#35856=CARTESIAN_POINT('Ctrl Pts',(1.31731642317187,-1.,-1.5768005650559));
#35857=CARTESIAN_POINT('Ctrl Pts',(1.31731642317187,1.,-1.5768005650559));
#35858=CARTESIAN_POINT('Ctrl Pts',(1.31900135021432,-1.,-1.58274907898834));
#35859=CARTESIAN_POINT('Ctrl Pts',(1.31900135021432,1.,-1.58274907898834));
#35860=CARTESIAN_POINT('Ctrl Pts',(1.32064537110892,-1.,-1.58872057258245));
#35861=CARTESIAN_POINT('Ctrl Pts',(1.32064537110892,1.,-1.58872057258245));
#35862=CARTESIAN_POINT('Ctrl Pts',(1.32224985747682,-1.,-1.59471591079403));
#35863=CARTESIAN_POINT('Ctrl Pts',(1.32224985747682,1.,-1.59471591079403));
#35864=CARTESIAN_POINT('Ctrl Pts',(1.32381550858256,-1.,-1.60073511858687));
#35865=CARTESIAN_POINT('Ctrl Pts',(1.32381550858256,1.,-1.60073511858687));
#35866=CARTESIAN_POINT('Ctrl Pts',(1.32534250785782,-1.,-1.60677758290954));
#35867=CARTESIAN_POINT('Ctrl Pts',(1.32534250785782,1.,-1.60677758290954));
#35868=CARTESIAN_POINT('Ctrl Pts',(1.32683074483356,-1.,-1.6128423401575));
#35869=CARTESIAN_POINT('Ctrl Pts',(1.32683074483356,1.,-1.6128423401575));
#35870=CARTESIAN_POINT('Ctrl Pts',(1.32828000610449,-1.,-1.61892832270724));
#35871=CARTESIAN_POINT('Ctrl Pts',(1.32828000610449,1.,-1.61892832270724));
#35872=CARTESIAN_POINT('Ctrl Pts',(1.3296901950568,-1.,-1.62503464209797));
#35873=CARTESIAN_POINT('Ctrl Pts',(1.3296901950568,1.,-1.62503464209797));
#35874=CARTESIAN_POINT('Ctrl Pts',(1.33106149345645,-1.,-1.63116079730923));
#35875=CARTESIAN_POINT('Ctrl Pts',(1.33106149345645,1.,-1.63116079730923));
#35876=CARTESIAN_POINT('Ctrl Pts',(1.33239425103724,-1.,-1.63730653475089));
#35877=CARTESIAN_POINT('Ctrl Pts',(1.33239425103724,1.,-1.63730653475089));
#35878=CARTESIAN_POINT('Ctrl Pts',(1.33368890676572,-1.,-1.6434717485603));
#35879=CARTESIAN_POINT('Ctrl Pts',(1.33368890676572,1.,-1.6434717485603));
#35880=CARTESIAN_POINT('Ctrl Pts',(1.33494590467993,-1.,-1.6496563728683));
#35881=CARTESIAN_POINT('Ctrl Pts',(1.33494590467993,1.,-1.6496563728683));
#35882=CARTESIAN_POINT('Ctrl Pts',(1.33616559745172,-1.,-1.65586025952593));
#35883=CARTESIAN_POINT('Ctrl Pts',(1.33616559745172,1.,-1.65586025952593));
#35884=CARTESIAN_POINT('Ctrl Pts',(1.33734820885262,-1.,-1.66208312541983));
#35885=CARTESIAN_POINT('Ctrl Pts',(1.33734820885262,1.,-1.66208312541983));
#35886=CARTESIAN_POINT('Ctrl Pts',(1.33849388654388,-1.,-1.66832460783989));
#35887=CARTESIAN_POINT('Ctrl Pts',(1.33849388654388,1.,-1.66832460783989));
#35888=CARTESIAN_POINT('Ctrl Pts',(1.3396027347034,-1.,-1.67458429426086));
#35889=CARTESIAN_POINT('Ctrl Pts',(1.3396027347034,1.,-1.67458429426086));
#35890=CARTESIAN_POINT('Ctrl Pts',(1.34067485185203,-1.,-1.68086176030362));
#35891=CARTESIAN_POINT('Ctrl Pts',(1.34067485185203,1.,-1.68086176030362));
#35892=CARTESIAN_POINT('Ctrl Pts',(1.341710374848,-1.,-1.68715660868764));
#35893=CARTESIAN_POINT('Ctrl Pts',(1.341710374848,1.,-1.68715660868764));
#35894=CARTESIAN_POINT('Ctrl Pts',(1.34270948206319,-1.,-1.6934684849687));
#35895=CARTESIAN_POINT('Ctrl Pts',(1.34270948206319,1.,-1.6934684849687));
#35896=CARTESIAN_POINT('Ctrl Pts',(1.34367237124483,-1.,-1.69979707754427));
#35897=CARTESIAN_POINT('Ctrl Pts',(1.34367237124483,1.,-1.69979707754427));
#35898=CARTESIAN_POINT('Ctrl Pts',(1.34459924533831,-1.,-1.70614212266738));
#35899=CARTESIAN_POINT('Ctrl Pts',(1.34459924533831,1.,-1.70614212266738));
#35900=CARTESIAN_POINT('Ctrl Pts',(1.34549029589416,-1.,-1.71250340686822));
#35901=CARTESIAN_POINT('Ctrl Pts',(1.34549029589416,1.,-1.71250340686822));
#35902=CARTESIAN_POINT('Ctrl Pts',(1.34634568653227,-1.,-1.7188807715049));
#35903=CARTESIAN_POINT('Ctrl Pts',(1.34634568653227,1.,-1.7188807715049));
#35904=CARTESIAN_POINT('Ctrl Pts',(1.34716554819527,-1.,-1.72527410680674));
#35905=CARTESIAN_POINT('Ctrl Pts',(1.34716554819527,1.,-1.72527410680674));
#35906=CARTESIAN_POINT('Ctrl Pts',(1.34779309152035,-1.,-1.7304014965394));
#35907=CARTESIAN_POINT('Ctrl Pts',(1.34779309152035,1.,-1.7304014965394));
#35908=CARTESIAN_POINT('Ctrl Pts',(1.34824783112887,-1.,-1.73425417885907));
#35909=CARTESIAN_POINT('Ctrl Pts',(1.34824783112887,1.,-1.73425417885907));
#35910=CARTESIAN_POINT('Ctrl Pts',(1.34854391898045,-1.,-1.73682580585691));
#35911=CARTESIAN_POINT('Ctrl Pts',(1.34854391898045,1.,-1.73682580585691));
#35912=CARTESIAN_POINT('Ctrl Pts',(1.34869019493419,-1.,-1.73811241238545));
#35913=CARTESIAN_POINT('Ctrl Pts',(1.34869019493419,1.,-1.73811241238545));
#35914=CARTESIAN_POINT('',(1.15624053661742,1.,-1.31362392696032));
#35915=CARTESIAN_POINT('Ctrl Pts',(1.15624053661742,1.,-1.31362392696032));
#35916=CARTESIAN_POINT('Ctrl Pts',(1.15950888730809,1.,-1.31722977216397));
#35917=CARTESIAN_POINT('Ctrl Pts',(1.16589330093588,1.,-1.32428080721772));
#35918=CARTESIAN_POINT('Ctrl Pts',(1.17501305789857,1.,-1.33437539347008));
#35919=CARTESIAN_POINT('Ctrl Pts',(1.18625865667441,1.,-1.34687054001093));
#35920=CARTESIAN_POINT('Ctrl Pts',(1.1987959077932,1.,-1.36088705043885));
#35921=CARTESIAN_POINT('Ctrl Pts',(1.20982812925645,1.,-1.37331915607905));
#35922=CARTESIAN_POINT('Ctrl Pts',(1.21938737280852,1.,-1.38420564527715));
#35923=CARTESIAN_POINT('Ctrl Pts',(1.22752961899387,1.,-1.39361389568796));
#35924=CARTESIAN_POINT('Ctrl Pts',(1.23434087290423,1.,-1.40164708206106));
#35925=CARTESIAN_POINT('Ctrl Pts',(1.23994455029534,1.,-1.40845295531283));
#35926=CARTESIAN_POINT('Ctrl Pts',(1.24450600513056,1.,-1.41422913175179));
#35927=CARTESIAN_POINT('Ctrl Pts',(1.24824430986571,1.,-1.41923722596025));
#35928=CARTESIAN_POINT('Ctrl Pts',(1.2514145557001,1.,-1.42378102115575));
#35929=CARTESIAN_POINT('Ctrl Pts',(1.25426945222639,1.,-1.42815938799387));
#35930=CARTESIAN_POINT('Ctrl Pts',(1.25702687965755,1.,-1.43262645609691));
#35931=CARTESIAN_POINT('Ctrl Pts',(1.25983531012005,1.,-1.43734919180848));
#35932=CARTESIAN_POINT('Ctrl Pts',(1.26273903323858,1.,-1.44236470511303));
#35933=CARTESIAN_POINT('Ctrl Pts',(1.26570925118868,1.,-1.44761985001662));
#35934=CARTESIAN_POINT('Ctrl Pts',(1.2686778680489,1.,-1.45301422764247));
#35935=CARTESIAN_POINT('Ctrl Pts',(1.27156805265289,1.,-1.45843906294697));
#35936=CARTESIAN_POINT('Ctrl Pts',(1.27433119897822,1.,-1.46382431332476));
#35937=CARTESIAN_POINT('Ctrl Pts',(1.27696414831089,1.,-1.46916035917133));
#35938=CARTESIAN_POINT('Ctrl Pts',(1.2794891824849,1.,-1.4744717526707));
#35939=CARTESIAN_POINT('Ctrl Pts',(1.28194158939517,1.,-1.47980070347096));
#35940=CARTESIAN_POINT('Ctrl Pts',(1.28435533880201,1.,-1.4851881711891));
#35941=CARTESIAN_POINT('Ctrl Pts',(1.2867467611644,1.,-1.4906522831278));
#35942=CARTESIAN_POINT('Ctrl Pts',(1.28911506584254,1.,-1.49618896881754));
#35943=CARTESIAN_POINT('Ctrl Pts',(1.29145022885181,1.,-1.50178230149776));
#35944=CARTESIAN_POINT('Ctrl Pts',(1.29373841372842,1.,-1.50741159078365));
#35945=CARTESIAN_POINT('Ctrl Pts',(1.29596850710509,1.,-1.51305994241402));
#35946=CARTESIAN_POINT('Ctrl Pts',(1.29813791800747,1.,-1.51872184912724));
#35947=CARTESIAN_POINT('Ctrl Pts',(1.30024984366328,1.,-1.52439957861062));
#35948=CARTESIAN_POINT('Ctrl Pts',(1.30231064395568,1.,-1.53009970283891));
#35949=CARTESIAN_POINT('Ctrl Pts',(1.30432735639489,1.,-1.53582981268977));
#35950=CARTESIAN_POINT('Ctrl Pts',(1.30630475189556,1.,-1.54159462645432));
#35951=CARTESIAN_POINT('Ctrl Pts',(1.30824393907473,1.,-1.54739413957185));
#35952=CARTESIAN_POINT('Ctrl Pts',(1.31014393684222,1.,-1.55322568759481));
#35953=CARTESIAN_POINT('Ctrl Pts',(1.31200264341696,1.,-1.55908521254821));
#35954=CARTESIAN_POINT('Ctrl Pts',(1.31381795281002,1.,-1.56496872402353));
#35955=CARTESIAN_POINT('Ctrl Pts',(1.31558903860016,1.,-1.57087397835723));
#35956=CARTESIAN_POINT('Ctrl Pts',(1.31731642317187,1.,-1.5768005650559));
#35957=CARTESIAN_POINT('Ctrl Pts',(1.31900135021432,1.,-1.58274907898834));
#35958=CARTESIAN_POINT('Ctrl Pts',(1.32064537110892,1.,-1.58872057258245));
#35959=CARTESIAN_POINT('Ctrl Pts',(1.32224985747682,1.,-1.59471591079403));
#35960=CARTESIAN_POINT('Ctrl Pts',(1.32381550858256,1.,-1.60073511858687));
#35961=CARTESIAN_POINT('Ctrl Pts',(1.32534250785782,1.,-1.60677758290954));
#35962=CARTESIAN_POINT('Ctrl Pts',(1.32683074483356,1.,-1.6128423401575));
#35963=CARTESIAN_POINT('Ctrl Pts',(1.32828000610449,1.,-1.61892832270724));
#35964=CARTESIAN_POINT('Ctrl Pts',(1.3296901950568,1.,-1.62503464209797));
#35965=CARTESIAN_POINT('Ctrl Pts',(1.33106149345645,1.,-1.63116079730923));
#35966=CARTESIAN_POINT('Ctrl Pts',(1.33239425103724,1.,-1.63730653475089));
#35967=CARTESIAN_POINT('Ctrl Pts',(1.33368890676572,1.,-1.6434717485603));
#35968=CARTESIAN_POINT('Ctrl Pts',(1.33494590467993,1.,-1.6496563728683));
#35969=CARTESIAN_POINT('Ctrl Pts',(1.33616559745172,1.,-1.65586025952593));
#35970=CARTESIAN_POINT('Ctrl Pts',(1.33734820885262,1.,-1.66208312541983));
#35971=CARTESIAN_POINT('Ctrl Pts',(1.33849388654388,1.,-1.66832460783989));
#35972=CARTESIAN_POINT('Ctrl Pts',(1.3396027347034,1.,-1.67458429426086));
#35973=CARTESIAN_POINT('Ctrl Pts',(1.34067485185203,1.,-1.68086176030362));
#35974=CARTESIAN_POINT('Ctrl Pts',(1.341710374848,1.,-1.68715660868764));
#35975=CARTESIAN_POINT('Ctrl Pts',(1.34270948206319,1.,-1.6934684849687));
#35976=CARTESIAN_POINT('Ctrl Pts',(1.34367237124483,1.,-1.69979707754427));
#35977=CARTESIAN_POINT('Ctrl Pts',(1.34459924533831,1.,-1.70614212266738));
#35978=CARTESIAN_POINT('Ctrl Pts',(1.34549029589416,1.,-1.71250340686822));
#35979=CARTESIAN_POINT('Ctrl Pts',(1.34634568653227,1.,-1.7188807715049));
#35980=CARTESIAN_POINT('Ctrl Pts',(1.34716554819527,1.,-1.72527410680674));
#35981=CARTESIAN_POINT('Ctrl Pts',(1.34779309152035,1.,-1.7304014965394));
#35982=CARTESIAN_POINT('Ctrl Pts',(1.34824783112887,1.,-1.73425417885907));
#35983=CARTESIAN_POINT('Ctrl Pts',(1.34854391898045,1.,-1.73682580585691));
#35984=CARTESIAN_POINT('Ctrl Pts',(1.34869019493419,1.,-1.73811241238545));
#35985=CARTESIAN_POINT('',(1.15624053661742,0.,-1.31362392696032));
#35986=CARTESIAN_POINT('Origin',(0.,0.,0.));
#35987=CARTESIAN_POINT('',(1.31362392696032,1.,-1.15624053661742));
#35988=CARTESIAN_POINT('Origin',(0.,1.,0.));
#35989=CARTESIAN_POINT('',(1.31362392696032,0.,-1.15624053661742));
#35990=CARTESIAN_POINT('Ctrl Pts',(1.73811241238545,-1.,-1.34869019493419));
#35991=CARTESIAN_POINT('Ctrl Pts',(1.73811241238545,1.,-1.34869019493419));
#35992=CARTESIAN_POINT('Ctrl Pts',(1.73682580585819,-1.,-1.34854391898145));
#35993=CARTESIAN_POINT('Ctrl Pts',(1.73682580585819,1.,-1.34854391898145));
#35994=CARTESIAN_POINT('Ctrl Pts',(1.73425417886254,-1.,-1.34824783113158));
#35995=CARTESIAN_POINT('Ctrl Pts',(1.73425417886254,1.,-1.34824783113158));
#35996=CARTESIAN_POINT('Ctrl Pts',(1.73040149654497,-1.,-1.3477930915247));
#35997=CARTESIAN_POINT('Ctrl Pts',(1.73040149654497,1.,-1.3477930915247));
#35998=CARTESIAN_POINT('Ctrl Pts',(1.72527410681298,-1.,-1.34716554820013));
#35999=CARTESIAN_POINT('Ctrl Pts',(1.72527410681298,1.,-1.34716554820013));
#36000=CARTESIAN_POINT('Ctrl Pts',(1.7188807715095,-1.,-1.34634568653586));
#36001=CARTESIAN_POINT('Ctrl Pts',(1.7188807715095,1.,-1.34634568653586));
#36002=CARTESIAN_POINT('Ctrl Pts',(1.71250340687011,-1.,-1.34549029589563));
#36003=CARTESIAN_POINT('Ctrl Pts',(1.71250340687011,1.,-1.34549029589563));
#36004=CARTESIAN_POINT('Ctrl Pts',(1.70614212266676,-1.,-1.34459924533783));
#36005=CARTESIAN_POINT('Ctrl Pts',(1.70614212266676,1.,-1.34459924533783));
#36006=CARTESIAN_POINT('Ctrl Pts',(1.69979707754221,-1.,-1.34367237124322));
#36007=CARTESIAN_POINT('Ctrl Pts',(1.69979707754221,1.,-1.34367237124322));
#36008=CARTESIAN_POINT('Ctrl Pts',(1.6934684849664,-1.,-1.34270948206139));
#36009=CARTESIAN_POINT('Ctrl Pts',(1.6934684849664,1.,-1.34270948206139));
#36010=CARTESIAN_POINT('Ctrl Pts',(1.68715660868602,-1.,-1.34171037484673));
#36011=CARTESIAN_POINT('Ctrl Pts',(1.68715660868602,1.,-1.34171037484673));
#36012=CARTESIAN_POINT('Ctrl Pts',(1.68086176030308,-1.,-1.3406748518516));
#36013=CARTESIAN_POINT('Ctrl Pts',(1.68086176030308,1.,-1.3406748518516));
#36014=CARTESIAN_POINT('Ctrl Pts',(1.67458429426126,-1.,-1.33960273470372));
#36015=CARTESIAN_POINT('Ctrl Pts',(1.67458429426126,1.,-1.33960273470372));
#36016=CARTESIAN_POINT('Ctrl Pts',(1.66832460784078,-1.,-1.33849388654458));
#36017=CARTESIAN_POINT('Ctrl Pts',(1.66832460784078,1.,-1.33849388654458));
#36018=CARTESIAN_POINT('Ctrl Pts',(1.66208312542073,-1.,-1.33734820885331));
#36019=CARTESIAN_POINT('Ctrl Pts',(1.66208312542073,1.,-1.33734820885331));
#36020=CARTESIAN_POINT('Ctrl Pts',(1.65586025952651,-1.,-1.33616559745217));
#36021=CARTESIAN_POINT('Ctrl Pts',(1.65586025952651,1.,-1.33616559745217));
#36022=CARTESIAN_POINT('Ctrl Pts',(1.64965637286843,-1.,-1.33494590468003));
#36023=CARTESIAN_POINT('Ctrl Pts',(1.64965637286843,1.,-1.33494590468003));
#36024=CARTESIAN_POINT('Ctrl Pts',(1.64347174856007,-1.,-1.33368890676554));
#36025=CARTESIAN_POINT('Ctrl Pts',(1.64347174856007,1.,-1.33368890676554));
#36026=CARTESIAN_POINT('Ctrl Pts',(1.63730653475049,-1.,-1.33239425103694));
#36027=CARTESIAN_POINT('Ctrl Pts',(1.63730653475049,1.,-1.33239425103694));
#36028=CARTESIAN_POINT('Ctrl Pts',(1.63116079730887,-1.,-1.33106149345618));
#36029=CARTESIAN_POINT('Ctrl Pts',(1.63116079730887,1.,-1.33106149345618));
#36030=CARTESIAN_POINT('Ctrl Pts',(1.62503464209777,-1.,-1.32969019505665));
#36031=CARTESIAN_POINT('Ctrl Pts',(1.62503464209777,1.,-1.32969019505665));
#36032=CARTESIAN_POINT('Ctrl Pts',(1.61892832270723,-1.,-1.32828000610448));
#36033=CARTESIAN_POINT('Ctrl Pts',(1.61892832270723,1.,-1.32828000610448));
#36034=CARTESIAN_POINT('Ctrl Pts',(1.61284234015762,-1.,-1.32683074483365));
#36035=CARTESIAN_POINT('Ctrl Pts',(1.61284234015762,1.,-1.32683074483365));
#36036=CARTESIAN_POINT('Ctrl Pts',(1.6067775829097,-1.,-1.32534250785794));
#36037=CARTESIAN_POINT('Ctrl Pts',(1.6067775829097,1.,-1.32534250785794));
#36038=CARTESIAN_POINT('Ctrl Pts',(1.600735118587,-1.,-1.32381550858266));
#36039=CARTESIAN_POINT('Ctrl Pts',(1.600735118587,1.,-1.32381550858266));
#36040=CARTESIAN_POINT('Ctrl Pts',(1.59471591079408,-1.,-1.32224985747686));
#36041=CARTESIAN_POINT('Ctrl Pts',(1.59471591079408,1.,-1.32224985747686));
#36042=CARTESIAN_POINT('Ctrl Pts',(1.58872057258244,-1.,-1.32064537110891));
#36043=CARTESIAN_POINT('Ctrl Pts',(1.58872057258244,1.,-1.32064537110891));
#36044=CARTESIAN_POINT('Ctrl Pts',(1.58274907898829,-1.,-1.31900135021428));
#36045=CARTESIAN_POINT('Ctrl Pts',(1.58274907898829,1.,-1.31900135021428));
#36046=CARTESIAN_POINT('Ctrl Pts',(1.57680056505585,-1.,-1.31731642317183));
#36047=CARTESIAN_POINT('Ctrl Pts',(1.57680056505585,1.,-1.31731642317183));
#36048=CARTESIAN_POINT('Ctrl Pts',(1.57087397835721,-1.,-1.31558903860015));
#36049=CARTESIAN_POINT('Ctrl Pts',(1.57087397835721,1.,-1.31558903860015));
#36050=CARTESIAN_POINT('Ctrl Pts',(1.56496872402352,-1.,-1.31381795281002));
#36051=CARTESIAN_POINT('Ctrl Pts',(1.56496872402352,1.,-1.31381795281002));
#36052=CARTESIAN_POINT('Ctrl Pts',(1.55908521254822,-1.,-1.31200264341696));
#36053=CARTESIAN_POINT('Ctrl Pts',(1.55908521254822,1.,-1.31200264341696));
#36054=CARTESIAN_POINT('Ctrl Pts',(1.55322568759481,-1.,-1.31014393684221));
#36055=CARTESIAN_POINT('Ctrl Pts',(1.55322568759481,1.,-1.31014393684221));
#36056=CARTESIAN_POINT('Ctrl Pts',(1.54739413957183,-1.,-1.30824393907471));
#36057=CARTESIAN_POINT('Ctrl Pts',(1.54739413957183,1.,-1.30824393907471));
#36058=CARTESIAN_POINT('Ctrl Pts',(1.54159462645428,-1.,-1.30630475189553));
#36059=CARTESIAN_POINT('Ctrl Pts',(1.54159462645428,1.,-1.30630475189553));
#36060=CARTESIAN_POINT('Ctrl Pts',(1.53582981268976,-1.,-1.30432735639487));
#36061=CARTESIAN_POINT('Ctrl Pts',(1.53582981268976,1.,-1.30432735639487));
#36062=CARTESIAN_POINT('Ctrl Pts',(1.53009970283893,-1.,-1.3023106439557));
#36063=CARTESIAN_POINT('Ctrl Pts',(1.53009970283893,1.,-1.3023106439557));
#36064=CARTESIAN_POINT('Ctrl Pts',(1.5243995786107,-1.,-1.30024984366334));
#36065=CARTESIAN_POINT('Ctrl Pts',(1.5243995786107,1.,-1.30024984366334));
#36066=CARTESIAN_POINT('Ctrl Pts',(1.51872184912735,-1.,-1.29813791800757));
#36067=CARTESIAN_POINT('Ctrl Pts',(1.51872184912735,1.,-1.29813791800757));
#36068=CARTESIAN_POINT('Ctrl Pts',(1.51305994241412,-1.,-1.29596850710518));
#36069=CARTESIAN_POINT('Ctrl Pts',(1.51305994241412,1.,-1.29596850710518));
#36070=CARTESIAN_POINT('Ctrl Pts',(1.50741159078367,-1.,-1.29373841372843));
#36071=CARTESIAN_POINT('Ctrl Pts',(1.50741159078367,1.,-1.29373841372843));
#36072=CARTESIAN_POINT('Ctrl Pts',(1.50178230149764,-1.,-1.29145022885171));
#36073=CARTESIAN_POINT('Ctrl Pts',(1.50178230149764,1.,-1.29145022885171));
#36074=CARTESIAN_POINT('Ctrl Pts',(1.49618896881729,-1.,-1.28911506584232));
#36075=CARTESIAN_POINT('Ctrl Pts',(1.49618896881729,1.,-1.28911506584232));
#36076=CARTESIAN_POINT('Ctrl Pts',(1.4906522831275,-1.,-1.28674676116415));
#36077=CARTESIAN_POINT('Ctrl Pts',(1.4906522831275,1.,-1.28674676116415));
#36078=CARTESIAN_POINT('Ctrl Pts',(1.48518817118891,-1.,-1.28435533880184));
#36079=CARTESIAN_POINT('Ctrl Pts',(1.48518817118891,1.,-1.28435533880184));
#36080=CARTESIAN_POINT('Ctrl Pts',(1.47980070347102,-1.,-1.28194158939522));
#36081=CARTESIAN_POINT('Ctrl Pts',(1.47980070347102,1.,-1.28194158939522));
#36082=CARTESIAN_POINT('Ctrl Pts',(1.4744717526711,-1.,-1.27948918248524));
#36083=CARTESIAN_POINT('Ctrl Pts',(1.4744717526711,1.,-1.27948918248524));
#36084=CARTESIAN_POINT('Ctrl Pts',(1.46916035917197,-1.,-1.27696414831144));
#36085=CARTESIAN_POINT('Ctrl Pts',(1.46916035917197,1.,-1.27696414831144));
#36086=CARTESIAN_POINT('Ctrl Pts',(1.4638243133254,-1.,-1.27433119897877));
#36087=CARTESIAN_POINT('Ctrl Pts',(1.4638243133254,1.,-1.27433119897877));
#36088=CARTESIAN_POINT('Ctrl Pts',(1.45843906294725,-1.,-1.27156805265312));
#36089=CARTESIAN_POINT('Ctrl Pts',(1.45843906294725,1.,-1.27156805265312));
#36090=CARTESIAN_POINT('Ctrl Pts',(1.45301422764205,-1.,-1.26867786804854));
#36091=CARTESIAN_POINT('Ctrl Pts',(1.45301422764205,1.,-1.26867786804854));
#36092=CARTESIAN_POINT('Ctrl Pts',(1.44761985001544,-1.,-1.26570925118767));
#36093=CARTESIAN_POINT('Ctrl Pts',(1.44761985001544,1.,-1.26570925118767));
#36094=CARTESIAN_POINT('Ctrl Pts',(1.44236470511145,-1.,-1.26273903323723));
#36095=CARTESIAN_POINT('Ctrl Pts',(1.44236470511145,1.,-1.26273903323723));
#36096=CARTESIAN_POINT('Ctrl Pts',(1.43734919180719,-1.,-1.25983531011894));
#36097=CARTESIAN_POINT('Ctrl Pts',(1.43734919180719,1.,-1.25983531011894));
#36098=CARTESIAN_POINT('Ctrl Pts',(1.43262645609679,-1.,-1.25702687965744));
#36099=CARTESIAN_POINT('Ctrl Pts',(1.43262645609679,1.,-1.25702687965744));
#36100=CARTESIAN_POINT('Ctrl Pts',(1.42815938799555,-1.,-1.25426945222783));
#36101=CARTESIAN_POINT('Ctrl Pts',(1.42815938799555,1.,-1.25426945222783));
#36102=CARTESIAN_POINT('Ctrl Pts',(1.42378102115911,-1.,-1.25141455570299));
#36103=CARTESIAN_POINT('Ctrl Pts',(1.42378102115911,1.,-1.25141455570299));
#36104=CARTESIAN_POINT('Ctrl Pts',(1.41923722596421,-1.,-1.24824430986911));
#36105=CARTESIAN_POINT('Ctrl Pts',(1.41923722596421,1.,-1.24824430986911));
#36106=CARTESIAN_POINT('Ctrl Pts',(1.41422913175437,-1.,-1.24450600513278));
#36107=CARTESIAN_POINT('Ctrl Pts',(1.41422913175437,1.,-1.24450600513278));
#36108=CARTESIAN_POINT('Ctrl Pts',(1.40845295531151,-1.,-1.23994455029421));
#36109=CARTESIAN_POINT('Ctrl Pts',(1.40845295531151,1.,-1.23994455029421));
#36110=CARTESIAN_POINT('Ctrl Pts',(1.40164708205345,-1.,-1.23434087289768));
#36111=CARTESIAN_POINT('Ctrl Pts',(1.40164708205345,1.,-1.23434087289768));
#36112=CARTESIAN_POINT('Ctrl Pts',(1.39361389567257,-1.,-1.22752961898063));
#36113=CARTESIAN_POINT('Ctrl Pts',(1.39361389567257,1.,-1.22752961898063));
#36114=CARTESIAN_POINT('Ctrl Pts',(1.38420564525391,-1.,-1.21938737278853));
#36115=CARTESIAN_POINT('Ctrl Pts',(1.38420564525391,1.,-1.21938737278853));
#36116=CARTESIAN_POINT('Ctrl Pts',(1.37331915604962,-1.,-1.20982812923113));
#36117=CARTESIAN_POINT('Ctrl Pts',(1.37331915604962,1.,-1.20982812923113));
#36118=CARTESIAN_POINT('Ctrl Pts',(1.36088705040677,-1.,-1.1987959077656));
#36119=CARTESIAN_POINT('Ctrl Pts',(1.36088705040677,1.,-1.1987959077656));
#36120=CARTESIAN_POINT('Ctrl Pts',(1.34687053998157,-1.,-1.18625865664915));
#36121=CARTESIAN_POINT('Ctrl Pts',(1.34687053998157,1.,-1.18625865664915));
#36122=CARTESIAN_POINT('Ctrl Pts',(1.33437539344842,-1.,-1.17501305787994));
#36123=CARTESIAN_POINT('Ctrl Pts',(1.33437539344842,1.,-1.17501305787994));
#36124=CARTESIAN_POINT('Ctrl Pts',(1.32428080720544,-1.,-1.16589330092532));
#36125=CARTESIAN_POINT('Ctrl Pts',(1.32428080720544,1.,-1.16589330092532));
#36126=CARTESIAN_POINT('Ctrl Pts',(1.3172297721596,-1.,-1.15950888730433));
#36127=CARTESIAN_POINT('Ctrl Pts',(1.3172297721596,1.,-1.15950888730433));
#36128=CARTESIAN_POINT('Ctrl Pts',(1.31362392696032,-1.,-1.15624053661742));
#36129=CARTESIAN_POINT('Ctrl Pts',(1.31362392696032,1.,-1.15624053661742));
#36130=CARTESIAN_POINT('',(1.73811241238545,1.,-1.34869019493419));
#36131=CARTESIAN_POINT('Ctrl Pts',(1.73811241238545,1.,-1.34869019493419));
#36132=CARTESIAN_POINT('Ctrl Pts',(1.73682580585819,1.,-1.34854391898145));
#36133=CARTESIAN_POINT('Ctrl Pts',(1.73425417886254,1.,-1.34824783113158));
#36134=CARTESIAN_POINT('Ctrl Pts',(1.73040149654497,1.,-1.3477930915247));
#36135=CARTESIAN_POINT('Ctrl Pts',(1.72527410681298,1.,-1.34716554820013));
#36136=CARTESIAN_POINT('Ctrl Pts',(1.7188807715095,1.,-1.34634568653586));
#36137=CARTESIAN_POINT('Ctrl Pts',(1.71250340687011,1.,-1.34549029589563));
#36138=CARTESIAN_POINT('Ctrl Pts',(1.70614212266676,1.,-1.34459924533783));
#36139=CARTESIAN_POINT('Ctrl Pts',(1.69979707754221,1.,-1.34367237124322));
#36140=CARTESIAN_POINT('Ctrl Pts',(1.6934684849664,1.,-1.34270948206139));
#36141=CARTESIAN_POINT('Ctrl Pts',(1.68715660868602,1.,-1.34171037484673));
#36142=CARTESIAN_POINT('Ctrl Pts',(1.68086176030308,1.,-1.3406748518516));
#36143=CARTESIAN_POINT('Ctrl Pts',(1.67458429426126,1.,-1.33960273470372));
#36144=CARTESIAN_POINT('Ctrl Pts',(1.66832460784078,1.,-1.33849388654458));
#36145=CARTESIAN_POINT('Ctrl Pts',(1.66208312542073,1.,-1.33734820885331));
#36146=CARTESIAN_POINT('Ctrl Pts',(1.65586025952651,1.,-1.33616559745217));
#36147=CARTESIAN_POINT('Ctrl Pts',(1.64965637286843,1.,-1.33494590468003));
#36148=CARTESIAN_POINT('Ctrl Pts',(1.64347174856007,1.,-1.33368890676554));
#36149=CARTESIAN_POINT('Ctrl Pts',(1.63730653475049,1.,-1.33239425103694));
#36150=CARTESIAN_POINT('Ctrl Pts',(1.63116079730887,1.,-1.33106149345618));
#36151=CARTESIAN_POINT('Ctrl Pts',(1.62503464209777,1.,-1.32969019505665));
#36152=CARTESIAN_POINT('Ctrl Pts',(1.61892832270723,1.,-1.32828000610448));
#36153=CARTESIAN_POINT('Ctrl Pts',(1.61284234015762,1.,-1.32683074483365));
#36154=CARTESIAN_POINT('Ctrl Pts',(1.6067775829097,1.,-1.32534250785794));
#36155=CARTESIAN_POINT('Ctrl Pts',(1.600735118587,1.,-1.32381550858266));
#36156=CARTESIAN_POINT('Ctrl Pts',(1.59471591079408,1.,-1.32224985747686));
#36157=CARTESIAN_POINT('Ctrl Pts',(1.58872057258244,1.,-1.32064537110891));
#36158=CARTESIAN_POINT('Ctrl Pts',(1.58274907898829,1.,-1.31900135021428));
#36159=CARTESIAN_POINT('Ctrl Pts',(1.57680056505585,1.,-1.31731642317183));
#36160=CARTESIAN_POINT('Ctrl Pts',(1.57087397835721,1.,-1.31558903860015));
#36161=CARTESIAN_POINT('Ctrl Pts',(1.56496872402352,1.,-1.31381795281002));
#36162=CARTESIAN_POINT('Ctrl Pts',(1.55908521254822,1.,-1.31200264341696));
#36163=CARTESIAN_POINT('Ctrl Pts',(1.55322568759481,1.,-1.31014393684221));
#36164=CARTESIAN_POINT('Ctrl Pts',(1.54739413957183,1.,-1.30824393907471));
#36165=CARTESIAN_POINT('Ctrl Pts',(1.54159462645428,1.,-1.30630475189553));
#36166=CARTESIAN_POINT('Ctrl Pts',(1.53582981268976,1.,-1.30432735639487));
#36167=CARTESIAN_POINT('Ctrl Pts',(1.53009970283893,1.,-1.3023106439557));
#36168=CARTESIAN_POINT('Ctrl Pts',(1.5243995786107,1.,-1.30024984366334));
#36169=CARTESIAN_POINT('Ctrl Pts',(1.51872184912735,1.,-1.29813791800757));
#36170=CARTESIAN_POINT('Ctrl Pts',(1.51305994241412,1.,-1.29596850710518));
#36171=CARTESIAN_POINT('Ctrl Pts',(1.50741159078367,1.,-1.29373841372843));
#36172=CARTESIAN_POINT('Ctrl Pts',(1.50178230149764,1.,-1.29145022885171));
#36173=CARTESIAN_POINT('Ctrl Pts',(1.49618896881729,1.,-1.28911506584232));
#36174=CARTESIAN_POINT('Ctrl Pts',(1.4906522831275,1.,-1.28674676116415));
#36175=CARTESIAN_POINT('Ctrl Pts',(1.48518817118891,1.,-1.28435533880184));
#36176=CARTESIAN_POINT('Ctrl Pts',(1.47980070347102,1.,-1.28194158939522));
#36177=CARTESIAN_POINT('Ctrl Pts',(1.4744717526711,1.,-1.27948918248524));
#36178=CARTESIAN_POINT('Ctrl Pts',(1.46916035917197,1.,-1.27696414831144));
#36179=CARTESIAN_POINT('Ctrl Pts',(1.4638243133254,1.,-1.27433119897877));
#36180=CARTESIAN_POINT('Ctrl Pts',(1.45843906294725,1.,-1.27156805265312));
#36181=CARTESIAN_POINT('Ctrl Pts',(1.45301422764205,1.,-1.26867786804854));
#36182=CARTESIAN_POINT('Ctrl Pts',(1.44761985001544,1.,-1.26570925118767));
#36183=CARTESIAN_POINT('Ctrl Pts',(1.44236470511145,1.,-1.26273903323723));
#36184=CARTESIAN_POINT('Ctrl Pts',(1.43734919180719,1.,-1.25983531011894));
#36185=CARTESIAN_POINT('Ctrl Pts',(1.43262645609679,1.,-1.25702687965744));
#36186=CARTESIAN_POINT('Ctrl Pts',(1.42815938799555,1.,-1.25426945222783));
#36187=CARTESIAN_POINT('Ctrl Pts',(1.42378102115911,1.,-1.25141455570299));
#36188=CARTESIAN_POINT('Ctrl Pts',(1.41923722596421,1.,-1.24824430986911));
#36189=CARTESIAN_POINT('Ctrl Pts',(1.41422913175437,1.,-1.24450600513278));
#36190=CARTESIAN_POINT('Ctrl Pts',(1.40845295531151,1.,-1.23994455029421));
#36191=CARTESIAN_POINT('Ctrl Pts',(1.40164708205345,1.,-1.23434087289768));
#36192=CARTESIAN_POINT('Ctrl Pts',(1.39361389567257,1.,-1.22752961898063));
#36193=CARTESIAN_POINT('Ctrl Pts',(1.38420564525391,1.,-1.21938737278853));
#36194=CARTESIAN_POINT('Ctrl Pts',(1.37331915604962,1.,-1.20982812923113));
#36195=CARTESIAN_POINT('Ctrl Pts',(1.36088705040677,1.,-1.1987959077656));
#36196=CARTESIAN_POINT('Ctrl Pts',(1.34687053998157,1.,-1.18625865664915));
#36197=CARTESIAN_POINT('Ctrl Pts',(1.33437539344842,1.,-1.17501305787994));
#36198=CARTESIAN_POINT('Ctrl Pts',(1.32428080720544,1.,-1.16589330092532));
#36199=CARTESIAN_POINT('Ctrl Pts',(1.3172297721596,1.,-1.15950888730433));
#36200=CARTESIAN_POINT('Ctrl Pts',(1.31362392696032,1.,-1.15624053661742));
#36201=CARTESIAN_POINT('',(1.73811241238545,0.,-1.34869019493419));
#36202=CARTESIAN_POINT('Origin',(1.81978687191668,0.,-1.23627494547115));
#36203=CARTESIAN_POINT('',(1.81978687191668,1.,-1.23627494547115));
#36204=CARTESIAN_POINT('',(1.73811241238545,1.,-1.34869019493419));
#36205=CARTESIAN_POINT('',(1.81978687191668,0.,-1.23627494547115));
#36206=CARTESIAN_POINT('Ctrl Pts',(1.5055822144029,-1.,-0.892032620296855));
#36207=CARTESIAN_POINT('Ctrl Pts',(1.5055822144029,1.,-0.892032620296855));
#36208=CARTESIAN_POINT('Ctrl Pts',(1.50980486807181,-1.,-0.894452006967538));
#36209=CARTESIAN_POINT('Ctrl Pts',(1.50980486807181,1.,-0.894452006967538));
#36210=CARTESIAN_POINT('Ctrl Pts',(1.51805569591479,-1.,-0.89918504749193));
#36211=CARTESIAN_POINT('Ctrl Pts',(1.51805569591479,1.,-0.89918504749193));
#36212=CARTESIAN_POINT('Ctrl Pts',(1.52984849890434,-1.,-0.905967409640499));
#36213=CARTESIAN_POINT('Ctrl Pts',(1.52984849890434,1.,-0.905967409640499));
#36214=CARTESIAN_POINT('Ctrl Pts',(1.54440491152807,-1.,-0.91437591904658));
#36215=CARTESIAN_POINT('Ctrl Pts',(1.54440491152807,1.,-0.91437591904658));
#36216=CARTESIAN_POINT('Ctrl Pts',(1.56065988582509,-1.,-0.923832188966322));
#36217=CARTESIAN_POINT('Ctrl Pts',(1.56065988582509,1.,-0.923832188966322));
#36218=CARTESIAN_POINT('Ctrl Pts',(1.57499388385561,-1.,-0.932246680128849));
#36219=CARTESIAN_POINT('Ctrl Pts',(1.57499388385561,1.,-0.932246680128849));
#36220=CARTESIAN_POINT('Ctrl Pts',(1.58744937489796,-1.,-0.939646377909319));
#36221=CARTESIAN_POINT('Ctrl Pts',(1.58744937489796,1.,-0.939646377909319));
#36222=CARTESIAN_POINT('Ctrl Pts',(1.59810042045408,-1.,-0.946078063325796));
#36223=CARTESIAN_POINT('Ctrl Pts',(1.59810042045408,1.,-0.946078063325796));
#36224=CARTESIAN_POINT('Ctrl Pts',(1.60706069897794,-1.,-0.951613284361248));
#36225=CARTESIAN_POINT('Ctrl Pts',(1.60706069897794,1.,-0.951613284361248));
#36226=CARTESIAN_POINT('Ctrl Pts',(1.61449324337233,-1.,-0.956354422921573));
#36227=CARTESIAN_POINT('Ctrl Pts',(1.61449324337233,1.,-0.956354422921573));
#36228=CARTESIAN_POINT('Ctrl Pts',(1.62061638139929,-1.,-0.960438326099958));
#36229=CARTESIAN_POINT('Ctrl Pts',(1.62061638139929,1.,-0.960438326099958));
#36230=CARTESIAN_POINT('Ctrl Pts',(1.6257193066974,-1.,-0.964046107037821));
#36231=CARTESIAN_POINT('Ctrl Pts',(1.6257193066974,1.,-0.964046107037821));
#36232=CARTESIAN_POINT('Ctrl Pts',(1.63013849959083,-1.,-0.967387853228041));
#36233=CARTESIAN_POINT('Ctrl Pts',(1.63013849959083,1.,-0.967387853228041));
#36234=CARTESIAN_POINT('Ctrl Pts',(1.63420665729609,-1.,-0.970669715996356));
#36235=CARTESIAN_POINT('Ctrl Pts',(1.63420665729609,1.,-0.970669715996356));
#36236=CARTESIAN_POINT('Ctrl Pts',(1.63820952658157,-1.,-0.974066058287501));
#36237=CARTESIAN_POINT('Ctrl Pts',(1.63820952658157,1.,-0.974066058287501));
#36238=CARTESIAN_POINT('Ctrl Pts',(1.64233990826831,-1.,-0.977689794120297));
#36239=CARTESIAN_POINT('Ctrl Pts',(1.64233990826831,1.,-0.977689794120297));
#36240=CARTESIAN_POINT('Ctrl Pts',(1.64665139190834,-1.,-0.981562530940574));
#36241=CARTESIAN_POINT('Ctrl Pts',(1.64665139190834,1.,-0.981562530940574));
#36242=CARTESIAN_POINT('Ctrl Pts',(1.6511001661277,-1.,-0.985642622921626));
#36243=CARTESIAN_POINT('Ctrl Pts',(1.6511001661277,1.,-0.985642622921626));
#36244=CARTESIAN_POINT('Ctrl Pts',(1.65559044289746,-1.,-0.98985562785445));
#36245=CARTESIAN_POINT('Ctrl Pts',(1.65559044289746,1.,-0.98985562785445));
#36246=CARTESIAN_POINT('Ctrl Pts',(1.66001553809916,-1.,-0.994121836661116));
#36247=CARTESIAN_POINT('Ctrl Pts',(1.66001553809916,1.,-0.994121836661116));
#36248=CARTESIAN_POINT('Ctrl Pts',(1.66430758030304,-1.,-0.998389654952317));
#36249=CARTESIAN_POINT('Ctrl Pts',(1.66430758030304,1.,-0.998389654952317));
#36250=CARTESIAN_POINT('Ctrl Pts',(1.66846059277231,-1.,-1.00265091003682));
#36251=CARTESIAN_POINT('Ctrl Pts',(1.66846059277231,1.,-1.00265091003682));
#36252=CARTESIAN_POINT('Ctrl Pts',(1.67250335383248,-1.,-1.00692206696387));
#36253=CARTESIAN_POINT('Ctrl Pts',(1.67250335383248,1.,-1.00692206696387));
#36254=CARTESIAN_POINT('Ctrl Pts',(1.67648246776457,-1.,-1.01123236493507));
#36255=CARTESIAN_POINT('Ctrl Pts',(1.67648246776457,1.,-1.01123236493507));
#36256=CARTESIAN_POINT('Ctrl Pts',(1.6804428989482,-1.,-1.01561026162787));
#36257=CARTESIAN_POINT('Ctrl Pts',(1.6804428989482,1.,-1.01561026162787));
#36258=CARTESIAN_POINT('Ctrl Pts',(1.68440578021739,-1.,-1.02006795074222));
#36259=CARTESIAN_POINT('Ctrl Pts',(1.68440578021739,1.,-1.02006795074222));
#36260=CARTESIAN_POINT('Ctrl Pts',(1.68836910178475,-1.,-1.02460180535272));
#36261=CARTESIAN_POINT('Ctrl Pts',(1.68836910178475,1.,-1.02460180535272));
#36262=CARTESIAN_POINT('Ctrl Pts',(1.69231840863471,-1.,-1.02919977579155));
#36263=CARTESIAN_POINT('Ctrl Pts',(1.69231840863471,1.,-1.02919977579155));
#36264=CARTESIAN_POINT('Ctrl Pts',(1.69623414782769,-1.,-1.03384646003587));
#36265=CARTESIAN_POINT('Ctrl Pts',(1.69623414782769,1.,-1.03384646003587));
#36266=CARTESIAN_POINT('Ctrl Pts',(1.70010052930951,-1.,-1.03852922490782));
#36267=CARTESIAN_POINT('Ctrl Pts',(1.70010052930951,1.,-1.03852922490782));
#36268=CARTESIAN_POINT('Ctrl Pts',(1.70391338707969,-1.,-1.04324363334546));
#36269=CARTESIAN_POINT('Ctrl Pts',(1.70391338707969,1.,-1.04324363334546));
#36270=CARTESIAN_POINT('Ctrl Pts',(1.70767646263641,-1.,-1.0479908540499));
#36271=CARTESIAN_POINT('Ctrl Pts',(1.70767646263641,1.,-1.0479908540499));
#36272=CARTESIAN_POINT('Ctrl Pts',(1.71139783543986,-1.,-1.05277517202854));
#36273=CARTESIAN_POINT('Ctrl Pts',(1.71139783543986,1.,-1.05277517202854));
#36274=CARTESIAN_POINT('Ctrl Pts',(1.71508654427022,-1.,-1.05760163192481));
#36275=CARTESIAN_POINT('Ctrl Pts',(1.71508654427022,1.,-1.05760163192481));
#36276=CARTESIAN_POINT('Ctrl Pts',(1.71874858456908,-1.,-1.0624732468065));
#36277=CARTESIAN_POINT('Ctrl Pts',(1.71874858456908,1.,-1.0624732468065));
#36278=CARTESIAN_POINT('Ctrl Pts',(1.72238500928456,-1.,-1.06738966975463));
#36279=CARTESIAN_POINT('Ctrl Pts',(1.72238500928456,1.,-1.06738966975463));
#36280=CARTESIAN_POINT('Ctrl Pts',(1.72599406198489,-1.,-1.07234866990252));
#36281=CARTESIAN_POINT('Ctrl Pts',(1.72599406198489,1.,-1.07234866990252));
#36282=CARTESIAN_POINT('Ctrl Pts',(1.72957248977424,-1.,-1.0773470373727));
#36283=CARTESIAN_POINT('Ctrl Pts',(1.72957248977424,1.,-1.0773470373727));
#36284=CARTESIAN_POINT('Ctrl Pts',(1.73311705663407,-1.,-1.08238162784749));
#36285=CARTESIAN_POINT('Ctrl Pts',(1.73311705663407,1.,-1.08238162784749));
#36286=CARTESIAN_POINT('Ctrl Pts',(1.73662628326093,-1.,-1.08745056285429));
#36287=CARTESIAN_POINT('Ctrl Pts',(1.73662628326093,1.,-1.08745056285429));
#36288=CARTESIAN_POINT('Ctrl Pts',(1.74010053962252,-1.,-1.09255329056496));
#36289=CARTESIAN_POINT('Ctrl Pts',(1.74010053962252,1.,-1.09255329056496));
#36290=CARTESIAN_POINT('Ctrl Pts',(1.74354119236212,-1.,-1.09768999241229));
#36291=CARTESIAN_POINT('Ctrl Pts',(1.74354119236212,1.,-1.09768999241229));
#36292=CARTESIAN_POINT('Ctrl Pts',(1.74695004214924,-1.,-1.10286118991144));
#36293=CARTESIAN_POINT('Ctrl Pts',(1.74695004214924,1.,-1.10286118991144));
#36294=CARTESIAN_POINT('Ctrl Pts',(1.75032866075914,-1.,-1.10806728183003));
#36295=CARTESIAN_POINT('Ctrl Pts',(1.75032866075914,1.,-1.10806728183003));
#36296=CARTESIAN_POINT('Ctrl Pts',(1.75367772094617,-1.,-1.11330807582542));
#36297=CARTESIAN_POINT('Ctrl Pts',(1.75367772094617,1.,-1.11330807582542));
#36298=CARTESIAN_POINT('Ctrl Pts',(1.75699720772089,-1.,-1.11858293216752));
#36299=CARTESIAN_POINT('Ctrl Pts',(1.75699720772089,1.,-1.11858293216752));
#36300=CARTESIAN_POINT('Ctrl Pts',(1.76028671825084,-1.,-1.12389096855078));
#36301=CARTESIAN_POINT('Ctrl Pts',(1.76028671825084,1.,-1.12389096855078));
#36302=CARTESIAN_POINT('Ctrl Pts',(1.76354571966171,-1.,-1.12923123555076));
#36303=CARTESIAN_POINT('Ctrl Pts',(1.76354571966171,1.,-1.12923123555076));
#36304=CARTESIAN_POINT('Ctrl Pts',(1.76677384551883,-1.,-1.13460291804635));
#36305=CARTESIAN_POINT('Ctrl Pts',(1.76677384551883,1.,-1.13460291804635));
#36306=CARTESIAN_POINT('Ctrl Pts',(1.76997111386806,-1.,-1.14000548337));
#36307=CARTESIAN_POINT('Ctrl Pts',(1.76997111386806,1.,-1.14000548337));
#36308=CARTESIAN_POINT('Ctrl Pts',(1.77313777896234,-1.,-1.14543858226948));
#36309=CARTESIAN_POINT('Ctrl Pts',(1.77313777896234,1.,-1.14543858226948));
#36310=CARTESIAN_POINT('Ctrl Pts',(1.77627422557034,-1.,-1.15090197841531));
#36311=CARTESIAN_POINT('Ctrl Pts',(1.77627422557034,1.,-1.15090197841531));
#36312=CARTESIAN_POINT('Ctrl Pts',(1.77938085564261,-1.,-1.15639547194689));
#36313=CARTESIAN_POINT('Ctrl Pts',(1.77938085564261,1.,-1.15639547194689));
#36314=CARTESIAN_POINT('Ctrl Pts',(1.78245795880949,-1.,-1.16191881298458));
#36315=CARTESIAN_POINT('Ctrl Pts',(1.78245795880949,1.,-1.16191881298458));
#36316=CARTESIAN_POINT('Ctrl Pts',(1.78550566040349,-1.,-1.16747166312239));
#36317=CARTESIAN_POINT('Ctrl Pts',(1.78550566040349,1.,-1.16747166312239));
#36318=CARTESIAN_POINT('Ctrl Pts',(1.78852398877523,-1.,-1.17305363177265));
#36319=CARTESIAN_POINT('Ctrl Pts',(1.78852398877523,1.,-1.17305363177265));
#36320=CARTESIAN_POINT('Ctrl Pts',(1.79151291552646,-1.,-1.17866429440781));
#36321=CARTESIAN_POINT('Ctrl Pts',(1.79151291552646,1.,-1.17866429440781));
#36322=CARTESIAN_POINT('Ctrl Pts',(1.79447240321572,-1.,-1.18430321697471));
#36323=CARTESIAN_POINT('Ctrl Pts',(1.79447240321572,1.,-1.18430321697471));
#36324=CARTESIAN_POINT('Ctrl Pts',(1.79740245923649,-1.,-1.1899699793456));
#36325=CARTESIAN_POINT('Ctrl Pts',(1.79740245923649,1.,-1.1899699793456));
#36326=CARTESIAN_POINT('Ctrl Pts',(1.80030314370121,-1.,-1.19566418930405));
#36327=CARTESIAN_POINT('Ctrl Pts',(1.80030314370121,1.,-1.19566418930405));
#36328=CARTESIAN_POINT('Ctrl Pts',(1.8031745483882,-1.,-1.2013854893912));
#36329=CARTESIAN_POINT('Ctrl Pts',(1.8031745483882,1.,-1.2013854893912));
#36330=CARTESIAN_POINT('Ctrl Pts',(1.80601678480772,-1.,-1.20713356605519));
#36331=CARTESIAN_POINT('Ctrl Pts',(1.80601678480772,1.,-1.20713356605519));
#36332=CARTESIAN_POINT('Ctrl Pts',(1.80882996916931,-1.,-1.2129081570818));
#36333=CARTESIAN_POINT('Ctrl Pts',(1.80882996916931,1.,-1.2129081570818));
#36334=CARTESIAN_POINT('Ctrl Pts',(1.81161420806172,-1.,-1.2187090610323));
#36335=CARTESIAN_POINT('Ctrl Pts',(1.81161420806172,1.,-1.2187090610323));
#36336=CARTESIAN_POINT('Ctrl Pts',(1.81436959209778,-1.,-1.22453613304507));
#36337=CARTESIAN_POINT('Ctrl Pts',(1.81436959209778,1.,-1.22453613304507));
#36338=CARTESIAN_POINT('Ctrl Pts',(1.81655087183054,-1.,-1.22921864890975));
#36339=CARTESIAN_POINT('Ctrl Pts',(1.81655087183054,1.,-1.22921864890975));
#36340=CARTESIAN_POINT('Ctrl Pts',(1.81817389920914,-1.,-1.23274224526804));
#36341=CARTESIAN_POINT('Ctrl Pts',(1.81817389920914,1.,-1.23274224526804));
#36342=CARTESIAN_POINT('Ctrl Pts',(1.81925017193531,-1.,-1.23509651170384));
#36343=CARTESIAN_POINT('Ctrl Pts',(1.81925017193531,1.,-1.23509651170384));
#36344=CARTESIAN_POINT('Ctrl Pts',(1.81978687191668,-1.,-1.23627494547115));
#36345=CARTESIAN_POINT('Ctrl Pts',(1.81978687191668,1.,-1.23627494547115));
#36346=CARTESIAN_POINT('',(1.5055822144029,1.,-0.892032620296855));
#36347=CARTESIAN_POINT('Ctrl Pts',(1.5055822144029,1.,-0.892032620296855));
#36348=CARTESIAN_POINT('Ctrl Pts',(1.50980486807181,1.,-0.894452006967538));
#36349=CARTESIAN_POINT('Ctrl Pts',(1.51805569591479,1.,-0.89918504749193));
#36350=CARTESIAN_POINT('Ctrl Pts',(1.52984849890434,1.,-0.905967409640499));
#36351=CARTESIAN_POINT('Ctrl Pts',(1.54440491152807,1.,-0.91437591904658));
#36352=CARTESIAN_POINT('Ctrl Pts',(1.56065988582509,1.,-0.923832188966322));
#36353=CARTESIAN_POINT('Ctrl Pts',(1.57499388385561,1.,-0.932246680128849));
#36354=CARTESIAN_POINT('Ctrl Pts',(1.58744937489796,1.,-0.939646377909319));
#36355=CARTESIAN_POINT('Ctrl Pts',(1.59810042045408,1.,-0.946078063325796));
#36356=CARTESIAN_POINT('Ctrl Pts',(1.60706069897794,1.,-0.951613284361248));
#36357=CARTESIAN_POINT('Ctrl Pts',(1.61449324337233,1.,-0.956354422921573));
#36358=CARTESIAN_POINT('Ctrl Pts',(1.62061638139929,1.,-0.960438326099958));
#36359=CARTESIAN_POINT('Ctrl Pts',(1.6257193066974,1.,-0.964046107037821));
#36360=CARTESIAN_POINT('Ctrl Pts',(1.63013849959083,1.,-0.967387853228041));
#36361=CARTESIAN_POINT('Ctrl Pts',(1.63420665729609,1.,-0.970669715996356));
#36362=CARTESIAN_POINT('Ctrl Pts',(1.63820952658157,1.,-0.974066058287501));
#36363=CARTESIAN_POINT('Ctrl Pts',(1.64233990826831,1.,-0.977689794120297));
#36364=CARTESIAN_POINT('Ctrl Pts',(1.64665139190834,1.,-0.981562530940574));
#36365=CARTESIAN_POINT('Ctrl Pts',(1.6511001661277,1.,-0.985642622921626));
#36366=CARTESIAN_POINT('Ctrl Pts',(1.65559044289746,1.,-0.98985562785445));
#36367=CARTESIAN_POINT('Ctrl Pts',(1.66001553809916,1.,-0.994121836661116));
#36368=CARTESIAN_POINT('Ctrl Pts',(1.66430758030304,1.,-0.998389654952317));
#36369=CARTESIAN_POINT('Ctrl Pts',(1.66846059277231,1.,-1.00265091003682));
#36370=CARTESIAN_POINT('Ctrl Pts',(1.67250335383248,1.,-1.00692206696387));
#36371=CARTESIAN_POINT('Ctrl Pts',(1.67648246776457,1.,-1.01123236493507));
#36372=CARTESIAN_POINT('Ctrl Pts',(1.6804428989482,1.,-1.01561026162787));
#36373=CARTESIAN_POINT('Ctrl Pts',(1.68440578021739,1.,-1.02006795074222));
#36374=CARTESIAN_POINT('Ctrl Pts',(1.68836910178475,1.,-1.02460180535272));
#36375=CARTESIAN_POINT('Ctrl Pts',(1.69231840863471,1.,-1.02919977579155));
#36376=CARTESIAN_POINT('Ctrl Pts',(1.69623414782769,1.,-1.03384646003587));
#36377=CARTESIAN_POINT('Ctrl Pts',(1.70010052930951,1.,-1.03852922490782));
#36378=CARTESIAN_POINT('Ctrl Pts',(1.70391338707969,1.,-1.04324363334546));
#36379=CARTESIAN_POINT('Ctrl Pts',(1.70767646263641,1.,-1.0479908540499));
#36380=CARTESIAN_POINT('Ctrl Pts',(1.71139783543986,1.,-1.05277517202854));
#36381=CARTESIAN_POINT('Ctrl Pts',(1.71508654427022,1.,-1.05760163192481));
#36382=CARTESIAN_POINT('Ctrl Pts',(1.71874858456908,1.,-1.0624732468065));
#36383=CARTESIAN_POINT('Ctrl Pts',(1.72238500928456,1.,-1.06738966975463));
#36384=CARTESIAN_POINT('Ctrl Pts',(1.72599406198489,1.,-1.07234866990252));
#36385=CARTESIAN_POINT('Ctrl Pts',(1.72957248977424,1.,-1.0773470373727));
#36386=CARTESIAN_POINT('Ctrl Pts',(1.73311705663407,1.,-1.08238162784749));
#36387=CARTESIAN_POINT('Ctrl Pts',(1.73662628326093,1.,-1.08745056285429));
#36388=CARTESIAN_POINT('Ctrl Pts',(1.74010053962252,1.,-1.09255329056496));
#36389=CARTESIAN_POINT('Ctrl Pts',(1.74354119236212,1.,-1.09768999241229));
#36390=CARTESIAN_POINT('Ctrl Pts',(1.74695004214924,1.,-1.10286118991144));
#36391=CARTESIAN_POINT('Ctrl Pts',(1.75032866075914,1.,-1.10806728183003));
#36392=CARTESIAN_POINT('Ctrl Pts',(1.75367772094617,1.,-1.11330807582542));
#36393=CARTESIAN_POINT('Ctrl Pts',(1.75699720772089,1.,-1.11858293216752));
#36394=CARTESIAN_POINT('Ctrl Pts',(1.76028671825084,1.,-1.12389096855078));
#36395=CARTESIAN_POINT('Ctrl Pts',(1.76354571966171,1.,-1.12923123555076));
#36396=CARTESIAN_POINT('Ctrl Pts',(1.76677384551883,1.,-1.13460291804635));
#36397=CARTESIAN_POINT('Ctrl Pts',(1.76997111386806,1.,-1.14000548337));
#36398=CARTESIAN_POINT('Ctrl Pts',(1.77313777896234,1.,-1.14543858226948));
#36399=CARTESIAN_POINT('Ctrl Pts',(1.77627422557034,1.,-1.15090197841531));
#36400=CARTESIAN_POINT('Ctrl Pts',(1.77938085564261,1.,-1.15639547194689));
#36401=CARTESIAN_POINT('Ctrl Pts',(1.78245795880949,1.,-1.16191881298458));
#36402=CARTESIAN_POINT('Ctrl Pts',(1.78550566040349,1.,-1.16747166312239));
#36403=CARTESIAN_POINT('Ctrl Pts',(1.78852398877523,1.,-1.17305363177265));
#36404=CARTESIAN_POINT('Ctrl Pts',(1.79151291552646,1.,-1.17866429440781));
#36405=CARTESIAN_POINT('Ctrl Pts',(1.79447240321572,1.,-1.18430321697471));
#36406=CARTESIAN_POINT('Ctrl Pts',(1.79740245923649,1.,-1.1899699793456));
#36407=CARTESIAN_POINT('Ctrl Pts',(1.80030314370121,1.,-1.19566418930405));
#36408=CARTESIAN_POINT('Ctrl Pts',(1.8031745483882,1.,-1.2013854893912));
#36409=CARTESIAN_POINT('Ctrl Pts',(1.80601678480772,1.,-1.20713356605519));
#36410=CARTESIAN_POINT('Ctrl Pts',(1.80882996916931,1.,-1.2129081570818));
#36411=CARTESIAN_POINT('Ctrl Pts',(1.81161420806172,1.,-1.2187090610323));
#36412=CARTESIAN_POINT('Ctrl Pts',(1.81436959209778,1.,-1.22453613304507));
#36413=CARTESIAN_POINT('Ctrl Pts',(1.81655087183054,1.,-1.22921864890975));
#36414=CARTESIAN_POINT('Ctrl Pts',(1.81817389920914,1.,-1.23274224526804));
#36415=CARTESIAN_POINT('Ctrl Pts',(1.81925017193531,1.,-1.23509651170384));
#36416=CARTESIAN_POINT('Ctrl Pts',(1.81978687191668,1.,-1.23627494547115));
#36417=CARTESIAN_POINT('',(1.5055822144029,0.,-0.892032620296855));
#36418=CARTESIAN_POINT('Origin',(0.,0.,0.));
#36419=CARTESIAN_POINT('',(1.60662857109684,1.,-0.693717979106306));
#36420=CARTESIAN_POINT('Origin',(0.,1.,0.));
#36421=CARTESIAN_POINT('',(1.60662857109684,0.,-0.693717979106308));
#36422=CARTESIAN_POINT('Ctrl Pts',(2.0698113262342,-1.,-0.745574324794401));
#36423=CARTESIAN_POINT('Ctrl Pts',(2.0698113262342,1.,-0.745574324794401));
#36424=CARTESIAN_POINT('Ctrl Pts',(2.06854248895728,-1.,-0.745832791378367));
#36425=CARTESIAN_POINT('Ctrl Pts',(2.06854248895728,1.,-0.745832791378367));
#36426=CARTESIAN_POINT('Ctrl Pts',(2.06600523016815,-1.,-0.746345871544201));
#36427=CARTESIAN_POINT('Ctrl Pts',(2.06600523016815,1.,-0.746345871544201));
#36428=CARTESIAN_POINT('Ctrl Pts',(2.06220058927826,-1.,-0.74710393278792));
#36429=CARTESIAN_POINT('Ctrl Pts',(2.06220058927826,1.,-0.74710393278792));
#36430=CARTESIAN_POINT('Ctrl Pts',(2.05713023031006,-1.,-0.748091554183803));
#36431=CARTESIAN_POINT('Ctrl Pts',(2.05713023031006,1.,-0.748091554183803));
#36432=CARTESIAN_POINT('Ctrl Pts',(2.05079645592154,-1.,-0.749287468665046));
#36433=CARTESIAN_POINT('Ctrl Pts',(2.05079645592154,1.,-0.749287468665046));
#36434=CARTESIAN_POINT('Ctrl Pts',(2.04446689147979,-1.,-0.750444657875576));
#36435=CARTESIAN_POINT('Ctrl Pts',(2.04446689147979,1.,-0.750444657875576));
#36436=CARTESIAN_POINT('Ctrl Pts',(2.03814160092099,-1.,-0.751562963361115));
#36437=CARTESIAN_POINT('Ctrl Pts',(2.03814160092099,1.,-0.751562963361115));
#36438=CARTESIAN_POINT('Ctrl Pts',(2.03182068456221,-1.,-0.752642180487211));
#36439=CARTESIAN_POINT('Ctrl Pts',(2.03182068456221,1.,-0.752642180487211));
#36440=CARTESIAN_POINT('Ctrl Pts',(2.02550428623313,-1.,-0.753682061112768));
#36441=CARTESIAN_POINT('Ctrl Pts',(2.02550428623313,1.,-0.753682061112768));
#36442=CARTESIAN_POINT('Ctrl Pts',(2.01919259405809,-1.,-0.754682330722816));
#36443=CARTESIAN_POINT('Ctrl Pts',(2.01919259405809,1.,-0.754682330722816));
#36444=CARTESIAN_POINT('Ctrl Pts',(2.01288584328084,-1.,-0.755642704957865));
#36445=CARTESIAN_POINT('Ctrl Pts',(2.01288584328084,1.,-0.755642704957865));
#36446=CARTESIAN_POINT('Ctrl Pts',(2.0065843158773,-1.,-0.756562904646671));
#36447=CARTESIAN_POINT('Ctrl Pts',(2.0065843158773,1.,-0.756562904646671));
#36448=CARTESIAN_POINT('Ctrl Pts',(2.00028834739178,-1.,-0.757442676862724));
#36449=CARTESIAN_POINT('Ctrl Pts',(2.00028834739178,1.,-0.757442676862724));
#36450=CARTESIAN_POINT('Ctrl Pts',(1.99399831098817,-1.,-0.758281796766761));
#36451=CARTESIAN_POINT('Ctrl Pts',(1.99399831098817,1.,-0.758281796766761));
#36452=CARTESIAN_POINT('Ctrl Pts',(1.98771456680874,-1.,-0.759080037802488));
#36453=CARTESIAN_POINT('Ctrl Pts',(1.98771456680874,1.,-0.759080037802488));
#36454=CARTESIAN_POINT('Ctrl Pts',(1.98143741418172,-1.,-0.75983714745219));
#36455=CARTESIAN_POINT('Ctrl Pts',(1.98143741418172,1.,-0.75983714745219));
#36456=CARTESIAN_POINT('Ctrl Pts',(1.97516705321494,-1.,-0.760552825409757));
#36457=CARTESIAN_POINT('Ctrl Pts',(1.97516705321494,1.,-0.760552825409757));
#36458=CARTESIAN_POINT('Ctrl Pts',(1.96890351582499,-1.,-0.761226690483821));
#36459=CARTESIAN_POINT('Ctrl Pts',(1.96890351582499,1.,-0.761226690483821));
#36460=CARTESIAN_POINT('Ctrl Pts',(1.96264672744186,-1.,-0.761858300014424));
#36461=CARTESIAN_POINT('Ctrl Pts',(1.96264672744186,1.,-0.761858300014424));
#36462=CARTESIAN_POINT('Ctrl Pts',(1.95639665309869,-1.,-0.762447203806179));
#36463=CARTESIAN_POINT('Ctrl Pts',(1.95639665309869,1.,-0.762447203806179));
#36464=CARTESIAN_POINT('Ctrl Pts',(1.95015342590024,-1.,-0.762992990878769));
#36465=CARTESIAN_POINT('Ctrl Pts',(1.95015342590024,1.,-0.762992990878769));
#36466=CARTESIAN_POINT('Ctrl Pts',(1.9439174661764,-1.,-0.763495333538629));
#36467=CARTESIAN_POINT('Ctrl Pts',(1.9439174661764,1.,-0.763495333538629));
#36468=CARTESIAN_POINT('Ctrl Pts',(1.93768964875886,-1.,-0.763954049121459));
#36469=CARTESIAN_POINT('Ctrl Pts',(1.93768964875886,1.,-0.763954049121459));
#36470=CARTESIAN_POINT('Ctrl Pts',(1.93147105496382,-1.,-0.764369010673941));
#36471=CARTESIAN_POINT('Ctrl Pts',(1.93147105496382,1.,-0.764369010673941));
#36472=CARTESIAN_POINT('Ctrl Pts',(1.92526263537048,-1.,-0.764740025488212));
#36473=CARTESIAN_POINT('Ctrl Pts',(1.92526263537048,1.,-0.764740025488212));
#36474=CARTESIAN_POINT('Ctrl Pts',(1.91906491634196,-1.,-0.765066729667089));
#36475=CARTESIAN_POINT('Ctrl Pts',(1.91906491634196,1.,-0.765066729667089));
#36476=CARTESIAN_POINT('Ctrl Pts',(1.91287765805169,-1.,-0.765348465884722));
#36477=CARTESIAN_POINT('Ctrl Pts',(1.91287765805169,1.,-0.765348465884722));
#36478=CARTESIAN_POINT('Ctrl Pts',(1.90669961402356,-1.,-0.765584196937919));
#36479=CARTESIAN_POINT('Ctrl Pts',(1.90669961402356,1.,-0.765584196937919));
#36480=CARTESIAN_POINT('Ctrl Pts',(1.90052930393596,-1.,-0.765772772593386));
#36481=CARTESIAN_POINT('Ctrl Pts',(1.90052930393596,1.,-0.765772772593386));
#36482=CARTESIAN_POINT('Ctrl Pts',(1.89436577771388,-1.,-0.765913193856978));
#36483=CARTESIAN_POINT('Ctrl Pts',(1.89436577771388,1.,-0.765913193856978));
#36484=CARTESIAN_POINT('Ctrl Pts',(1.88820926433409,-1.,-0.766004837062091));
#36485=CARTESIAN_POINT('Ctrl Pts',(1.88820926433409,1.,-0.766004837062091));
#36486=CARTESIAN_POINT('Ctrl Pts',(1.88206215302561,-1.,-0.766047794851865));
#36487=CARTESIAN_POINT('Ctrl Pts',(1.88206215302561,1.,-0.766047794851865));
#36488=CARTESIAN_POINT('Ctrl Pts',(1.87592888967883,-1.,-0.766042837036744));
#36489=CARTESIAN_POINT('Ctrl Pts',(1.87592888967883,1.,-0.766042837036744));
#36490=CARTESIAN_POINT('Ctrl Pts',(1.86981398314341,-1.,-0.765990708546091));
#36491=CARTESIAN_POINT('Ctrl Pts',(1.86981398314341,1.,-0.765990708546091));
#36492=CARTESIAN_POINT('Ctrl Pts',(1.86372027063312,-1.,-0.765891519092547));
#36493=CARTESIAN_POINT('Ctrl Pts',(1.86372027063312,1.,-0.765891519092547));
#36494=CARTESIAN_POINT('Ctrl Pts',(1.85764741390394,-1.,-0.765744212909319));
#36495=CARTESIAN_POINT('Ctrl Pts',(1.85764741390394,1.,-0.765744212909319));
#36496=CARTESIAN_POINT('Ctrl Pts',(1.85158945130063,-1.,-0.765545710619063));
#36497=CARTESIAN_POINT('Ctrl Pts',(1.85158945130063,1.,-0.765545710619063));
#36498=CARTESIAN_POINT('Ctrl Pts',(1.84553698875924,-1.,-0.765291664862029));
#36499=CARTESIAN_POINT('Ctrl Pts',(1.84553698875924,1.,-0.765291664862029));
#36500=CARTESIAN_POINT('Ctrl Pts',(1.83948181064835,-1.,-0.764978057881738));
#36501=CARTESIAN_POINT('Ctrl Pts',(1.83948181064835,1.,-0.764978057881738));
#36502=CARTESIAN_POINT('Ctrl Pts',(1.83342077227142,-1.,-0.764602549687853));
#36503=CARTESIAN_POINT('Ctrl Pts',(1.83342077227142,1.,-0.764602549687853));
#36504=CARTESIAN_POINT('Ctrl Pts',(1.82735991200065,-1.,-0.764165902605995));
#36505=CARTESIAN_POINT('Ctrl Pts',(1.82735991200065,1.,-0.764165902605995));
#36506=CARTESIAN_POINT('Ctrl Pts',(1.82131873145266,-1.,-0.763673465462727));
#36507=CARTESIAN_POINT('Ctrl Pts',(1.82131873145266,1.,-0.763673465462727));
#36508=CARTESIAN_POINT('Ctrl Pts',(1.8153211840553,-1.,-0.763132003836634));
#36509=CARTESIAN_POINT('Ctrl Pts',(1.8153211840553,1.,-0.763132003836634));
#36510=CARTESIAN_POINT('Ctrl Pts',(1.80938551463965,-1.,-0.762546129463938));
#36511=CARTESIAN_POINT('Ctrl Pts',(1.80938551463965,1.,-0.762546129463938));
#36512=CARTESIAN_POINT('Ctrl Pts',(1.80351583877342,-1.,-0.761915336443547));
#36513=CARTESIAN_POINT('Ctrl Pts',(1.80351583877342,1.,-0.761915336443547));
#36514=CARTESIAN_POINT('Ctrl Pts',(1.79768986997783,-1.,-0.761229695230558));
#36515=CARTESIAN_POINT('Ctrl Pts',(1.79768986997783,1.,-0.761229695230558));
#36516=CARTESIAN_POINT('Ctrl Pts',(1.7918581561088,-1.,-0.760469555880749));
#36517=CARTESIAN_POINT('Ctrl Pts',(1.7918581561088,1.,-0.760469555880749));
#36518=CARTESIAN_POINT('Ctrl Pts',(1.78596964884604,-1.,-0.75961440111019));
#36519=CARTESIAN_POINT('Ctrl Pts',(1.78596964884604,1.,-0.75961440111019));
#36520=CARTESIAN_POINT('Ctrl Pts',(1.77999411220945,-1.,-0.758650626677519));
#36521=CARTESIAN_POINT('Ctrl Pts',(1.77999411220945,1.,-0.758650626677519));
#36522=CARTESIAN_POINT('Ctrl Pts',(1.77394167108292,-1.,-0.757578264077029));
#36523=CARTESIAN_POINT('Ctrl Pts',(1.77394167108292,1.,-0.757578264077029));
#36524=CARTESIAN_POINT('Ctrl Pts',(1.76789396002998,-1.,-0.75642189602781));
#36525=CARTESIAN_POINT('Ctrl Pts',(1.76789396002998,1.,-0.75642189602781));
#36526=CARTESIAN_POINT('Ctrl Pts',(1.76197817240128,-1.,-0.755220979974462));
#36527=CARTESIAN_POINT('Ctrl Pts',(1.76197817240128,1.,-0.755220979974462));
#36528=CARTESIAN_POINT('Ctrl Pts',(1.75631083600019,-1.,-0.754009254027829));
#36529=CARTESIAN_POINT('Ctrl Pts',(1.75631083600019,1.,-0.754009254027829));
#36530=CARTESIAN_POINT('Ctrl Pts',(1.75095139468794,-1.,-0.752797683531314));
#36531=CARTESIAN_POINT('Ctrl Pts',(1.75095139468794,1.,-0.752797683531314));
#36532=CARTESIAN_POINT('Ctrl Pts',(1.74585086852502,-1.,-0.751555614164483));
#36533=CARTESIAN_POINT('Ctrl Pts',(1.74585086852502,1.,-0.751555614164483));
#36534=CARTESIAN_POINT('Ctrl Pts',(1.74080458267114,-1.,-0.75019343598125));
#36535=CARTESIAN_POINT('Ctrl Pts',(1.74080458267114,1.,-0.75019343598125));
#36536=CARTESIAN_POINT('Ctrl Pts',(1.7355035168033,-1.,-0.74858246295687));
#36537=CARTESIAN_POINT('Ctrl Pts',(1.7355035168033,1.,-0.74858246295687));
#36538=CARTESIAN_POINT('Ctrl Pts',(1.72958533647714,-1.,-0.746574710097752));
#36539=CARTESIAN_POINT('Ctrl Pts',(1.72958533647714,1.,-0.746574710097752));
#36540=CARTESIAN_POINT('Ctrl Pts',(1.72268229916769,-1.,-0.744021445433094));
#36541=CARTESIAN_POINT('Ctrl Pts',(1.72268229916769,1.,-0.744021445433094));
#36542=CARTESIAN_POINT('Ctrl Pts',(1.71447789751001,-1.,-0.74079516202821));
#36543=CARTESIAN_POINT('Ctrl Pts',(1.71447789751001,1.,-0.74079516202821));
#36544=CARTESIAN_POINT('Ctrl Pts',(1.70473309004249,-1.,-0.736799665716932));
#36545=CARTESIAN_POINT('Ctrl Pts',(1.70473309004249,1.,-0.736799665716932));
#36546=CARTESIAN_POINT('Ctrl Pts',(1.69326921972915,-1.,-0.731963238685357));
#36547=CARTESIAN_POINT('Ctrl Pts',(1.69326921972915,1.,-0.731963238685357));
#36548=CARTESIAN_POINT('Ctrl Pts',(1.67996158451922,-1.,-0.726235967982445));
#36549=CARTESIAN_POINT('Ctrl Pts',(1.67996158451922,1.,-0.726235967982445));
#36550=CARTESIAN_POINT('Ctrl Pts',(1.66472880551777,-1.,-0.71958543378795));
#36551=CARTESIAN_POINT('Ctrl Pts',(1.66472880551777,1.,-0.71958543378795));
#36552=CARTESIAN_POINT('Ctrl Pts',(1.64752408828442,-1.,-0.711993139340448));
#36553=CARTESIAN_POINT('Ctrl Pts',(1.64752408828442,1.,-0.711993139340448));
#36554=CARTESIAN_POINT('Ctrl Pts',(1.6321654166204,-1.,-0.705159151977294));
#36555=CARTESIAN_POINT('Ctrl Pts',(1.6321654166204,1.,-0.705159151977294));
#36556=CARTESIAN_POINT('Ctrl Pts',(1.61974673471117,-1.,-0.699605146398837));
#36557=CARTESIAN_POINT('Ctrl Pts',(1.61974673471117,1.,-0.699605146398837));
#36558=CARTESIAN_POINT('Ctrl Pts',(1.61106790957619,-1.,-0.69571209787897));
#36559=CARTESIAN_POINT('Ctrl Pts',(1.61106790957619,1.,-0.69571209787897));
#36560=CARTESIAN_POINT('Ctrl Pts',(1.60662857109684,-1.,-0.693717979106306));
#36561=CARTESIAN_POINT('Ctrl Pts',(1.60662857109684,1.,-0.693717979106306));
#36562=CARTESIAN_POINT('',(2.0698113262342,1.,-0.745574324794401));
#36563=CARTESIAN_POINT('Ctrl Pts',(2.0698113262342,1.,-0.745574324794401));
#36564=CARTESIAN_POINT('Ctrl Pts',(2.06854248895728,1.,-0.745832791378367));
#36565=CARTESIAN_POINT('Ctrl Pts',(2.06600523016815,1.,-0.746345871544201));
#36566=CARTESIAN_POINT('Ctrl Pts',(2.06220058927826,1.,-0.74710393278792));
#36567=CARTESIAN_POINT('Ctrl Pts',(2.05713023031006,1.,-0.748091554183803));
#36568=CARTESIAN_POINT('Ctrl Pts',(2.05079645592154,1.,-0.749287468665046));
#36569=CARTESIAN_POINT('Ctrl Pts',(2.04446689147979,1.,-0.750444657875576));
#36570=CARTESIAN_POINT('Ctrl Pts',(2.03814160092099,1.,-0.751562963361115));
#36571=CARTESIAN_POINT('Ctrl Pts',(2.03182068456221,1.,-0.752642180487211));
#36572=CARTESIAN_POINT('Ctrl Pts',(2.02550428623313,1.,-0.753682061112768));
#36573=CARTESIAN_POINT('Ctrl Pts',(2.01919259405809,1.,-0.754682330722816));
#36574=CARTESIAN_POINT('Ctrl Pts',(2.01288584328084,1.,-0.755642704957865));
#36575=CARTESIAN_POINT('Ctrl Pts',(2.0065843158773,1.,-0.756562904646671));
#36576=CARTESIAN_POINT('Ctrl Pts',(2.00028834739178,1.,-0.757442676862724));
#36577=CARTESIAN_POINT('Ctrl Pts',(1.99399831098817,1.,-0.758281796766761));
#36578=CARTESIAN_POINT('Ctrl Pts',(1.98771456680874,1.,-0.759080037802488));
#36579=CARTESIAN_POINT('Ctrl Pts',(1.98143741418172,1.,-0.75983714745219));
#36580=CARTESIAN_POINT('Ctrl Pts',(1.97516705321494,1.,-0.760552825409757));
#36581=CARTESIAN_POINT('Ctrl Pts',(1.96890351582499,1.,-0.761226690483821));
#36582=CARTESIAN_POINT('Ctrl Pts',(1.96264672744186,1.,-0.761858300014424));
#36583=CARTESIAN_POINT('Ctrl Pts',(1.95639665309869,1.,-0.762447203806179));
#36584=CARTESIAN_POINT('Ctrl Pts',(1.95015342590024,1.,-0.762992990878769));
#36585=CARTESIAN_POINT('Ctrl Pts',(1.9439174661764,1.,-0.763495333538629));
#36586=CARTESIAN_POINT('Ctrl Pts',(1.93768964875886,1.,-0.763954049121459));
#36587=CARTESIAN_POINT('Ctrl Pts',(1.93147105496382,1.,-0.764369010673941));
#36588=CARTESIAN_POINT('Ctrl Pts',(1.92526263537048,1.,-0.764740025488212));
#36589=CARTESIAN_POINT('Ctrl Pts',(1.91906491634196,1.,-0.765066729667089));
#36590=CARTESIAN_POINT('Ctrl Pts',(1.91287765805169,1.,-0.765348465884722));
#36591=CARTESIAN_POINT('Ctrl Pts',(1.90669961402356,1.,-0.765584196937919));
#36592=CARTESIAN_POINT('Ctrl Pts',(1.90052930393596,1.,-0.765772772593386));
#36593=CARTESIAN_POINT('Ctrl Pts',(1.89436577771388,1.,-0.765913193856978));
#36594=CARTESIAN_POINT('Ctrl Pts',(1.88820926433409,1.,-0.766004837062091));
#36595=CARTESIAN_POINT('Ctrl Pts',(1.88206215302561,1.,-0.766047794851865));
#36596=CARTESIAN_POINT('Ctrl Pts',(1.87592888967883,1.,-0.766042837036744));
#36597=CARTESIAN_POINT('Ctrl Pts',(1.86981398314341,1.,-0.765990708546091));
#36598=CARTESIAN_POINT('Ctrl Pts',(1.86372027063312,1.,-0.765891519092547));
#36599=CARTESIAN_POINT('Ctrl Pts',(1.85764741390394,1.,-0.765744212909319));
#36600=CARTESIAN_POINT('Ctrl Pts',(1.85158945130063,1.,-0.765545710619063));
#36601=CARTESIAN_POINT('Ctrl Pts',(1.84553698875924,1.,-0.765291664862029));
#36602=CARTESIAN_POINT('Ctrl Pts',(1.83948181064835,1.,-0.764978057881738));
#36603=CARTESIAN_POINT('Ctrl Pts',(1.83342077227142,1.,-0.764602549687853));
#36604=CARTESIAN_POINT('Ctrl Pts',(1.82735991200065,1.,-0.764165902605995));
#36605=CARTESIAN_POINT('Ctrl Pts',(1.82131873145266,1.,-0.763673465462727));
#36606=CARTESIAN_POINT('Ctrl Pts',(1.8153211840553,1.,-0.763132003836634));
#36607=CARTESIAN_POINT('Ctrl Pts',(1.80938551463965,1.,-0.762546129463938));
#36608=CARTESIAN_POINT('Ctrl Pts',(1.80351583877342,1.,-0.761915336443547));
#36609=CARTESIAN_POINT('Ctrl Pts',(1.79768986997783,1.,-0.761229695230558));
#36610=CARTESIAN_POINT('Ctrl Pts',(1.7918581561088,1.,-0.760469555880749));
#36611=CARTESIAN_POINT('Ctrl Pts',(1.78596964884604,1.,-0.75961440111019));
#36612=CARTESIAN_POINT('Ctrl Pts',(1.77999411220945,1.,-0.758650626677519));
#36613=CARTESIAN_POINT('Ctrl Pts',(1.77394167108292,1.,-0.757578264077029));
#36614=CARTESIAN_POINT('Ctrl Pts',(1.76789396002998,1.,-0.75642189602781));
#36615=CARTESIAN_POINT('Ctrl Pts',(1.76197817240128,1.,-0.755220979974462));
#36616=CARTESIAN_POINT('Ctrl Pts',(1.75631083600019,1.,-0.754009254027829));
#36617=CARTESIAN_POINT('Ctrl Pts',(1.75095139468794,1.,-0.752797683531314));
#36618=CARTESIAN_POINT('Ctrl Pts',(1.74585086852502,1.,-0.751555614164483));
#36619=CARTESIAN_POINT('Ctrl Pts',(1.74080458267114,1.,-0.75019343598125));
#36620=CARTESIAN_POINT('Ctrl Pts',(1.7355035168033,1.,-0.74858246295687));
#36621=CARTESIAN_POINT('Ctrl Pts',(1.72958533647714,1.,-0.746574710097752));
#36622=CARTESIAN_POINT('Ctrl Pts',(1.72268229916769,1.,-0.744021445433094));
#36623=CARTESIAN_POINT('Ctrl Pts',(1.71447789751001,1.,-0.74079516202821));
#36624=CARTESIAN_POINT('Ctrl Pts',(1.70473309004249,1.,-0.736799665716932));
#36625=CARTESIAN_POINT('Ctrl Pts',(1.69326921972915,1.,-0.731963238685357));
#36626=CARTESIAN_POINT('Ctrl Pts',(1.67996158451922,1.,-0.726235967982445));
#36627=CARTESIAN_POINT('Ctrl Pts',(1.66472880551777,1.,-0.71958543378795));
#36628=CARTESIAN_POINT('Ctrl Pts',(1.64752408828442,1.,-0.711993139340448));
#36629=CARTESIAN_POINT('Ctrl Pts',(1.6321654166204,1.,-0.705159151977294));
#36630=CARTESIAN_POINT('Ctrl Pts',(1.61974673471117,1.,-0.699605146398837));
#36631=CARTESIAN_POINT('Ctrl Pts',(1.61106790957619,1.,-0.69571209787897));
#36632=CARTESIAN_POINT('Ctrl Pts',(1.60662857109684,1.,-0.693717979106306));
#36633=CARTESIAN_POINT('',(2.0698113262342,0.,-0.745574324794401));
#36634=CARTESIAN_POINT('Origin',(2.11275013067528,0.,-0.61342227326009));
#36635=CARTESIAN_POINT('',(2.11275013067528,1.,-0.61342227326009));
#36636=CARTESIAN_POINT('',(2.0698113262342,1.,-0.745574324794401));
#36637=CARTESIAN_POINT('',(2.11275013067528,0.,-0.61342227326009));
#36638=CARTESIAN_POINT('Ctrl Pts',(1.7075470150345,-1.,-0.383122945602004));
#36639=CARTESIAN_POINT('Ctrl Pts',(1.7075470150345,1.,-0.383122945602004));
#36640=CARTESIAN_POINT('Ctrl Pts',(1.71231062891958,-1.,-0.384119047315542));
#36641=CARTESIAN_POINT('Ctrl Pts',(1.71231062891958,1.,-0.384119047315542));
#36642=CARTESIAN_POINT('Ctrl Pts',(1.72162022246158,-1.,-0.38607079032701));
#36643=CARTESIAN_POINT('Ctrl Pts',(1.72162022246158,1.,-0.38607079032701));
#36644=CARTESIAN_POINT('Ctrl Pts',(1.7349317097561,-1.,-0.388877023509192));
#36645=CARTESIAN_POINT('Ctrl Pts',(1.7349317097561,1.,-0.388877023509192));
#36646=CARTESIAN_POINT('Ctrl Pts',(1.75137405313962,-1.,-0.392375812294307));
#36647=CARTESIAN_POINT('Ctrl Pts',(1.75137405313962,1.,-0.392375812294307));
#36648=CARTESIAN_POINT('Ctrl Pts',(1.7697556004756,-1.,-0.39634619612042));
#36649=CARTESIAN_POINT('Ctrl Pts',(1.7697556004756,1.,-0.39634619612042));
#36650=CARTESIAN_POINT('Ctrl Pts',(1.78598826347533,-1.,-0.399919403783081));
#36651=CARTESIAN_POINT('Ctrl Pts',(1.78598826347533,1.,-0.399919403783081));
#36652=CARTESIAN_POINT('Ctrl Pts',(1.80012077176221,-1.,-0.403107976170441));
#36653=CARTESIAN_POINT('Ctrl Pts',(1.80012077176221,1.,-0.403107976170441));
#36654=CARTESIAN_POINT('Ctrl Pts',(1.81223801813988,-1.,-0.405933518411838));
#36655=CARTESIAN_POINT('Ctrl Pts',(1.81223801813988,1.,-0.405933518411838));
#36656=CARTESIAN_POINT('Ctrl Pts',(1.8224702267854,-1.,-0.408428948108534));
#36657=CARTESIAN_POINT('Ctrl Pts',(1.8224702267854,1.,-0.408428948108534));
#36658=CARTESIAN_POINT('Ctrl Pts',(1.83100408895216,-1.,-0.410641256301675));
#36659=CARTESIAN_POINT('Ctrl Pts',(1.83100408895216,1.,-0.410641256301675));
#36660=CARTESIAN_POINT('Ctrl Pts',(1.83808953475839,-1.,-0.412633125322162));
#36661=CARTESIAN_POINT('Ctrl Pts',(1.83808953475839,1.,-0.412633125322162));
#36662=CARTESIAN_POINT('Ctrl Pts',(1.8440575707371,-1.,-0.41448743825434));
#36663=CARTESIAN_POINT('Ctrl Pts',(1.8440575707371,1.,-0.41448743825434));
#36664=CARTESIAN_POINT('Ctrl Pts',(1.84929312929882,-1.,-0.416300022038864));
#36665=CARTESIAN_POINT('Ctrl Pts',(1.84929312929882,1.,-0.416300022038864));
#36666=CARTESIAN_POINT('Ctrl Pts',(1.85417632856234,-1.,-0.418164129143534));
#36667=CARTESIAN_POINT('Ctrl Pts',(1.85417632856234,1.,-0.418164129143534));
#36668=CARTESIAN_POINT('Ctrl Pts',(1.85903281096686,-1.,-0.42015728797562));
#36669=CARTESIAN_POINT('Ctrl Pts',(1.85903281096686,1.,-0.42015728797562));
#36670=CARTESIAN_POINT('Ctrl Pts',(1.86408083334028,-1.,-0.422327307418275));
#36671=CARTESIAN_POINT('Ctrl Pts',(1.86408083334028,1.,-0.422327307418275));
#36672=CARTESIAN_POINT('Ctrl Pts',(1.86937803944323,-1.,-0.424678177291359));
#36673=CARTESIAN_POINT('Ctrl Pts',(1.86937803944323,1.,-0.424678177291359));
#36674=CARTESIAN_POINT('Ctrl Pts',(1.87486989291484,-1.,-0.427183828519102));
#36675=CARTESIAN_POINT('Ctrl Pts',(1.87486989291484,1.,-0.427183828519102));
#36676=CARTESIAN_POINT('Ctrl Pts',(1.88044229001832,-1.,-0.429803062482345));
#36677=CARTESIAN_POINT('Ctrl Pts',(1.88044229001832,1.,-0.429803062482345));
#36678=CARTESIAN_POINT('Ctrl Pts',(1.88596913666793,-1.,-0.432493038548748));
#36679=CARTESIAN_POINT('Ctrl Pts',(1.88596913666793,1.,-0.432493038548748));
#36680=CARTESIAN_POINT('Ctrl Pts',(1.89136993975504,-1.,-0.435225660963383));
#36681=CARTESIAN_POINT('Ctrl Pts',(1.89136993975504,1.,-0.435225660963383));
#36682=CARTESIAN_POINT('Ctrl Pts',(1.89663648956466,-1.,-0.437995003948244));
#36683=CARTESIAN_POINT('Ctrl Pts',(1.89663648956466,1.,-0.437995003948244));
#36684=CARTESIAN_POINT('Ctrl Pts',(1.90180124389086,-1.,-0.440807833704038));
#36685=CARTESIAN_POINT('Ctrl Pts',(1.90180124389086,1.,-0.440807833704038));
#36686=CARTESIAN_POINT('Ctrl Pts',(1.90691756144898,-1.,-0.443677556849151));
#36687=CARTESIAN_POINT('Ctrl Pts',(1.90691756144898,1.,-0.443677556849151));
#36688=CARTESIAN_POINT('Ctrl Pts',(1.9120369998112,-1.,-0.446617343485711));
#36689=CARTESIAN_POINT('Ctrl Pts',(1.9120369998112,1.,-0.446617343485711));
#36690=CARTESIAN_POINT('Ctrl Pts',(1.91718342555755,-1.,-0.449632260106662));
#36691=CARTESIAN_POINT('Ctrl Pts',(1.91718342555755,1.,-0.449632260106662));
#36692=CARTESIAN_POINT('Ctrl Pts',(1.92235380648502,-1.,-0.452719478359433));
#36693=CARTESIAN_POINT('Ctrl Pts',(1.92235380648502,1.,-0.452719478359433));
#36694=CARTESIAN_POINT('Ctrl Pts',(1.92753067150476,-1.,-0.455872005174371));
#36695=CARTESIAN_POINT('Ctrl Pts',(1.92753067150476,1.,-0.455872005174371));
#36696=CARTESIAN_POINT('Ctrl Pts',(1.93269066517934,-1.,-0.459081234547926));
#36697=CARTESIAN_POINT('Ctrl Pts',(1.93269066517934,1.,-0.459081234547926));
#36698=CARTESIAN_POINT('Ctrl Pts',(1.93781486640821,-1.,-0.462340031009057));
#36699=CARTESIAN_POINT('Ctrl Pts',(1.93781486640821,1.,-0.462340031009057));
#36700=CARTESIAN_POINT('Ctrl Pts',(1.9428979419619,-1.,-0.46564546202603));
#36701=CARTESIAN_POINT('Ctrl Pts',(1.9428979419619,1.,-0.46564546202603));
#36702=CARTESIAN_POINT('Ctrl Pts',(1.94794381136514,-1.,-0.468997482913135));
#36703=CARTESIAN_POINT('Ctrl Pts',(1.94794381136514,1.,-0.468997482913135));
#36704=CARTESIAN_POINT('Ctrl Pts',(1.95296148278133,-1.,-0.472397672264072));
#36705=CARTESIAN_POINT('Ctrl Pts',(1.95296148278133,1.,-0.472397672264072));
#36706=CARTESIAN_POINT('Ctrl Pts',(1.95796111148177,-1.,-0.475848034683176));
#36707=CARTESIAN_POINT('Ctrl Pts',(1.95796111148177,1.,-0.475848034683176));
#36708=CARTESIAN_POINT('Ctrl Pts',(1.96294933055943,-1.,-0.479349583074855));
#36709=CARTESIAN_POINT('Ctrl Pts',(1.96294933055943,1.,-0.479349583074855));
#36710=CARTESIAN_POINT('Ctrl Pts',(1.96792703422362,-1.,-0.482901662120691));
#36711=CARTESIAN_POINT('Ctrl Pts',(1.96792703422362,1.,-0.482901662120691));
#36712=CARTESIAN_POINT('Ctrl Pts',(1.97289186263272,-1.,-0.486502692907659));
#36713=CARTESIAN_POINT('Ctrl Pts',(1.97289186263272,1.,-0.486502692907659));
#36714=CARTESIAN_POINT('Ctrl Pts',(1.97783973019229,-1.,-0.490150627860953));
#36715=CARTESIAN_POINT('Ctrl Pts',(1.97783973019229,1.,-0.490150627860953));
#36716=CARTESIAN_POINT('Ctrl Pts',(1.98276658761821,-1.,-0.493843476541495));
#36717=CARTESIAN_POINT('Ctrl Pts',(1.98276658761821,1.,-0.493843476541495));
#36718=CARTESIAN_POINT('Ctrl Pts',(1.98767044752932,-1.,-0.497579909545574));
#36719=CARTESIAN_POINT('Ctrl Pts',(1.98767044752932,1.,-0.497579909545574));
#36720=CARTESIAN_POINT('Ctrl Pts',(1.99255149126155,-1.,-0.501359287727146));
#36721=CARTESIAN_POINT('Ctrl Pts',(1.99255149126155,1.,-0.501359287727146));
#36722=CARTESIAN_POINT('Ctrl Pts',(1.99741107463572,-1.,-0.505181361323026));
#36723=CARTESIAN_POINT('Ctrl Pts',(1.99741107463572,1.,-0.505181361323026));
#36724=CARTESIAN_POINT('Ctrl Pts',(2.00225107134734,-1.,-0.509046069886157));
#36725=CARTESIAN_POINT('Ctrl Pts',(2.00225107134734,1.,-0.509046069886157));
#36726=CARTESIAN_POINT('Ctrl Pts',(2.00707309946949,-1.,-0.512953306961793));
#36727=CARTESIAN_POINT('Ctrl Pts',(2.00707309946949,1.,-0.512953306961793));
#36728=CARTESIAN_POINT('Ctrl Pts',(2.01187773939242,-1.,-0.516902681728687));
#36729=CARTESIAN_POINT('Ctrl Pts',(2.01187773939242,1.,-0.516902681728687));
#36730=CARTESIAN_POINT('Ctrl Pts',(2.01666477917286,-1.,-0.520893590399371));
#36731=CARTESIAN_POINT('Ctrl Pts',(2.01666477917286,1.,-0.520893590399371));
#36732=CARTESIAN_POINT('Ctrl Pts',(2.02143356304698,-1.,-0.524925318333476));
#36733=CARTESIAN_POINT('Ctrl Pts',(2.02143356304698,1.,-0.524925318333476));
#36734=CARTESIAN_POINT('Ctrl Pts',(2.0261832908329,-1.,-0.528997127241914));
#36735=CARTESIAN_POINT('Ctrl Pts',(2.0261832908329,1.,-0.528997127241914));
#36736=CARTESIAN_POINT('Ctrl Pts',(2.03091336214426,-1.,-0.533108355132977));
#36737=CARTESIAN_POINT('Ctrl Pts',(2.03091336214426,1.,-0.533108355132977));
#36738=CARTESIAN_POINT('Ctrl Pts',(2.03562362954037,-1.,-0.537258489833262));
#36739=CARTESIAN_POINT('Ctrl Pts',(2.03562362954037,1.,-0.537258489833262));
#36740=CARTESIAN_POINT('Ctrl Pts',(2.04031422690527,-1.,-0.541447120615659));
#36741=CARTESIAN_POINT('Ctrl Pts',(2.04031422690527,1.,-0.541447120615659));
#36742=CARTESIAN_POINT('Ctrl Pts',(2.04498544714588,-1.,-0.54567390381743));
#36743=CARTESIAN_POINT('Ctrl Pts',(2.04498544714588,1.,-0.54567390381743));
#36744=CARTESIAN_POINT('Ctrl Pts',(2.04963761077958,-1.,-0.549938525150295));
#36745=CARTESIAN_POINT('Ctrl Pts',(2.04963761077958,1.,-0.549938525150295));
#36746=CARTESIAN_POINT('Ctrl Pts',(2.05427091604413,-1.,-0.554240657463906));
#36747=CARTESIAN_POINT('Ctrl Pts',(2.05427091604413,1.,-0.554240657463906));
#36748=CARTESIAN_POINT('Ctrl Pts',(2.05888537756462,-1.,-0.558579940185152));
#36749=CARTESIAN_POINT('Ctrl Pts',(2.05888537756462,1.,-0.558579940185152));
#36750=CARTESIAN_POINT('Ctrl Pts',(2.06348090160589,-1.,-0.562955993082262));
#36751=CARTESIAN_POINT('Ctrl Pts',(2.06348090160589,1.,-0.562955993082262));
#36752=CARTESIAN_POINT('Ctrl Pts',(2.06805732997334,-1.,-0.567368421181087));
#36753=CARTESIAN_POINT('Ctrl Pts',(2.06805732997334,1.,-0.567368421181087));
#36754=CARTESIAN_POINT('Ctrl Pts',(2.07261449292824,-1.,-0.571816823242603));
#36755=CARTESIAN_POINT('Ctrl Pts',(2.07261449292824,1.,-0.571816823242603));
#36756=CARTESIAN_POINT('Ctrl Pts',(2.07715226767559,-1.,-0.576300797416845));
#36757=CARTESIAN_POINT('Ctrl Pts',(2.07715226767559,1.,-0.576300797416845));
#36758=CARTESIAN_POINT('Ctrl Pts',(2.08167059018418,-1.,-0.580819952108064));
#36759=CARTESIAN_POINT('Ctrl Pts',(2.08167059018418,1.,-0.580819952108064));
#36760=CARTESIAN_POINT('Ctrl Pts',(2.08616943727951,-1.,-0.585373918991617));
#36761=CARTESIAN_POINT('Ctrl Pts',(2.08616943727951,1.,-0.585373918991617));
#36762=CARTESIAN_POINT('Ctrl Pts',(2.09064881812129,-1.,-0.589962365403406));
#36763=CARTESIAN_POINT('Ctrl Pts',(2.09064881812129,1.,-0.589962365403406));
#36764=CARTESIAN_POINT('Ctrl Pts',(2.0951087622027,-1.,-0.594585006052162));
#36765=CARTESIAN_POINT('Ctrl Pts',(2.0951087622027,1.,-0.594585006052162));
#36766=CARTESIAN_POINT('Ctrl Pts',(2.0995493086477,-1.,-0.599241616420534));
#36767=CARTESIAN_POINT('Ctrl Pts',(2.0995493086477,1.,-0.599241616420534));
#36768=CARTESIAN_POINT('Ctrl Pts',(2.10397049886949,-1.,-0.60393203073603));
#36769=CARTESIAN_POINT('Ctrl Pts',(2.10397049886949,1.,-0.60393203073603));
#36770=CARTESIAN_POINT('Ctrl Pts',(2.1074919961518,-1.,-0.607711315454876));
#36771=CARTESIAN_POINT('Ctrl Pts',(2.1074919961518,1.,-0.607711315454876));
#36772=CARTESIAN_POINT('Ctrl Pts',(2.11012443807238,-1.,-0.610560911689899));
#36773=CARTESIAN_POINT('Ctrl Pts',(2.11012443807238,1.,-0.610560911689899));
#36774=CARTESIAN_POINT('Ctrl Pts',(2.11187554259986,-1.,-0.6124673655618));
#36775=CARTESIAN_POINT('Ctrl Pts',(2.11187554259986,1.,-0.6124673655618));
#36776=CARTESIAN_POINT('Ctrl Pts',(2.11275013067528,-1.,-0.61342227326009));
#36777=CARTESIAN_POINT('Ctrl Pts',(2.11275013067528,1.,-0.61342227326009));
#36778=CARTESIAN_POINT('',(1.7075470150345,1.,-0.383122945602004));
#36779=CARTESIAN_POINT('Ctrl Pts',(1.7075470150345,1.,-0.383122945602004));
#36780=CARTESIAN_POINT('Ctrl Pts',(1.71231062891958,1.,-0.384119047315542));
#36781=CARTESIAN_POINT('Ctrl Pts',(1.72162022246158,1.,-0.38607079032701));
#36782=CARTESIAN_POINT('Ctrl Pts',(1.7349317097561,1.,-0.388877023509192));
#36783=CARTESIAN_POINT('Ctrl Pts',(1.75137405313962,1.,-0.392375812294307));
#36784=CARTESIAN_POINT('Ctrl Pts',(1.7697556004756,1.,-0.39634619612042));
#36785=CARTESIAN_POINT('Ctrl Pts',(1.78598826347533,1.,-0.399919403783081));
#36786=CARTESIAN_POINT('Ctrl Pts',(1.80012077176221,1.,-0.403107976170441));
#36787=CARTESIAN_POINT('Ctrl Pts',(1.81223801813988,1.,-0.405933518411838));
#36788=CARTESIAN_POINT('Ctrl Pts',(1.8224702267854,1.,-0.408428948108534));
#36789=CARTESIAN_POINT('Ctrl Pts',(1.83100408895216,1.,-0.410641256301675));
#36790=CARTESIAN_POINT('Ctrl Pts',(1.83808953475839,1.,-0.412633125322162));
#36791=CARTESIAN_POINT('Ctrl Pts',(1.8440575707371,1.,-0.41448743825434));
#36792=CARTESIAN_POINT('Ctrl Pts',(1.84929312929882,1.,-0.416300022038864));
#36793=CARTESIAN_POINT('Ctrl Pts',(1.85417632856234,1.,-0.418164129143534));
#36794=CARTESIAN_POINT('Ctrl Pts',(1.85903281096686,1.,-0.42015728797562));
#36795=CARTESIAN_POINT('Ctrl Pts',(1.86408083334028,1.,-0.422327307418275));
#36796=CARTESIAN_POINT('Ctrl Pts',(1.86937803944323,1.,-0.424678177291359));
#36797=CARTESIAN_POINT('Ctrl Pts',(1.87486989291484,1.,-0.427183828519102));
#36798=CARTESIAN_POINT('Ctrl Pts',(1.88044229001832,1.,-0.429803062482345));
#36799=CARTESIAN_POINT('Ctrl Pts',(1.88596913666793,1.,-0.432493038548748));
#36800=CARTESIAN_POINT('Ctrl Pts',(1.89136993975504,1.,-0.435225660963383));
#36801=CARTESIAN_POINT('Ctrl Pts',(1.89663648956466,1.,-0.437995003948244));
#36802=CARTESIAN_POINT('Ctrl Pts',(1.90180124389086,1.,-0.440807833704038));
#36803=CARTESIAN_POINT('Ctrl Pts',(1.90691756144898,1.,-0.443677556849151));
#36804=CARTESIAN_POINT('Ctrl Pts',(1.9120369998112,1.,-0.446617343485711));
#36805=CARTESIAN_POINT('Ctrl Pts',(1.91718342555755,1.,-0.449632260106662));
#36806=CARTESIAN_POINT('Ctrl Pts',(1.92235380648502,1.,-0.452719478359433));
#36807=CARTESIAN_POINT('Ctrl Pts',(1.92753067150476,1.,-0.455872005174371));
#36808=CARTESIAN_POINT('Ctrl Pts',(1.93269066517934,1.,-0.459081234547926));
#36809=CARTESIAN_POINT('Ctrl Pts',(1.93781486640821,1.,-0.462340031009057));
#36810=CARTESIAN_POINT('Ctrl Pts',(1.9428979419619,1.,-0.46564546202603));
#36811=CARTESIAN_POINT('Ctrl Pts',(1.94794381136514,1.,-0.468997482913135));
#36812=CARTESIAN_POINT('Ctrl Pts',(1.95296148278133,1.,-0.472397672264072));
#36813=CARTESIAN_POINT('Ctrl Pts',(1.95796111148177,1.,-0.475848034683176));
#36814=CARTESIAN_POINT('Ctrl Pts',(1.96294933055943,1.,-0.479349583074855));
#36815=CARTESIAN_POINT('Ctrl Pts',(1.96792703422362,1.,-0.482901662120691));
#36816=CARTESIAN_POINT('Ctrl Pts',(1.97289186263272,1.,-0.486502692907659));
#36817=CARTESIAN_POINT('Ctrl Pts',(1.97783973019229,1.,-0.490150627860953));
#36818=CARTESIAN_POINT('Ctrl Pts',(1.98276658761821,1.,-0.493843476541495));
#36819=CARTESIAN_POINT('Ctrl Pts',(1.98767044752932,1.,-0.497579909545574));
#36820=CARTESIAN_POINT('Ctrl Pts',(1.99255149126155,1.,-0.501359287727146));
#36821=CARTESIAN_POINT('Ctrl Pts',(1.99741107463572,1.,-0.505181361323026));
#36822=CARTESIAN_POINT('Ctrl Pts',(2.00225107134734,1.,-0.509046069886157));
#36823=CARTESIAN_POINT('Ctrl Pts',(2.00707309946949,1.,-0.512953306961793));
#36824=CARTESIAN_POINT('Ctrl Pts',(2.01187773939242,1.,-0.516902681728687));
#36825=CARTESIAN_POINT('Ctrl Pts',(2.01666477917286,1.,-0.520893590399371));
#36826=CARTESIAN_POINT('Ctrl Pts',(2.02143356304698,1.,-0.524925318333476));
#36827=CARTESIAN_POINT('Ctrl Pts',(2.0261832908329,1.,-0.528997127241914));
#36828=CARTESIAN_POINT('Ctrl Pts',(2.03091336214426,1.,-0.533108355132977));
#36829=CARTESIAN_POINT('Ctrl Pts',(2.03562362954037,1.,-0.537258489833262));
#36830=CARTESIAN_POINT('Ctrl Pts',(2.04031422690527,1.,-0.541447120615659));
#36831=CARTESIAN_POINT('Ctrl Pts',(2.04498544714588,1.,-0.54567390381743));
#36832=CARTESIAN_POINT('Ctrl Pts',(2.04963761077958,1.,-0.549938525150295));
#36833=CARTESIAN_POINT('Ctrl Pts',(2.05427091604413,1.,-0.554240657463906));
#36834=CARTESIAN_POINT('Ctrl Pts',(2.05888537756462,1.,-0.558579940185152));
#36835=CARTESIAN_POINT('Ctrl Pts',(2.06348090160589,1.,-0.562955993082262));
#36836=CARTESIAN_POINT('Ctrl Pts',(2.06805732997334,1.,-0.567368421181087));
#36837=CARTESIAN_POINT('Ctrl Pts',(2.07261449292824,1.,-0.571816823242603));
#36838=CARTESIAN_POINT('Ctrl Pts',(2.07715226767559,1.,-0.576300797416845));
#36839=CARTESIAN_POINT('Ctrl Pts',(2.08167059018418,1.,-0.580819952108064));
#36840=CARTESIAN_POINT('Ctrl Pts',(2.08616943727951,1.,-0.585373918991617));
#36841=CARTESIAN_POINT('Ctrl Pts',(2.09064881812129,1.,-0.589962365403406));
#36842=CARTESIAN_POINT('Ctrl Pts',(2.0951087622027,1.,-0.594585006052162));
#36843=CARTESIAN_POINT('Ctrl Pts',(2.0995493086477,1.,-0.599241616420534));
#36844=CARTESIAN_POINT('Ctrl Pts',(2.10397049886949,1.,-0.60393203073603));
#36845=CARTESIAN_POINT('Ctrl Pts',(2.1074919961518,1.,-0.607711315454876));
#36846=CARTESIAN_POINT('Ctrl Pts',(2.11012443807238,1.,-0.610560911689899));
#36847=CARTESIAN_POINT('Ctrl Pts',(2.11187554259986,1.,-0.6124673655618));
#36848=CARTESIAN_POINT('Ctrl Pts',(2.11275013067528,1.,-0.61342227326009));
#36849=CARTESIAN_POINT('',(1.7075470150345,0.,-0.383122945602001));
#36850=CARTESIAN_POINT('Origin',(0.,0.,0.));
#36851=CARTESIAN_POINT('',(1.74236521665491,1.,-0.163289472382896));
#36852=CARTESIAN_POINT('Origin',(0.,1.,0.));
#36853=CARTESIAN_POINT('',(1.74236521665491,0.,-0.163289472382896));
#36854=CARTESIAN_POINT('Ctrl Pts',(2.19890268624765,-1.,-0.0694764450219582));
#36855=CARTESIAN_POINT('Ctrl Pts',(2.19890268624765,1.,-0.0694764450219582));
#36856=CARTESIAN_POINT('Ctrl Pts',(2.19777582085423,-1.,-0.0701143536325491));
#36857=CARTESIAN_POINT('Ctrl Pts',(2.19777582085423,1.,-0.0701143536325491));
#36858=CARTESIAN_POINT('Ctrl Pts',(2.19552129484002,-1.,-0.0713863779526155));
#36859=CARTESIAN_POINT('Ctrl Pts',(2.19552129484002,1.,-0.0713863779526155));
#36860=CARTESIAN_POINT('Ctrl Pts',(2.19213712013662,-1.,-0.0732830357306726));
#36861=CARTESIAN_POINT('Ctrl Pts',(2.19213712013662,1.,-0.0732830357306726));
#36862=CARTESIAN_POINT('Ctrl Pts',(2.1876201139953,-1.,-0.0757891465836149));
#36863=CARTESIAN_POINT('Ctrl Pts',(2.1876201139953,1.,-0.0757891465836149));
#36864=CARTESIAN_POINT('Ctrl Pts',(2.18196589448887,-1.,-0.0788837727685244));
#36865=CARTESIAN_POINT('Ctrl Pts',(2.18196589448887,1.,-0.0788837727685244));
#36866=CARTESIAN_POINT('Ctrl Pts',(2.176303712113,-1.,-0.0819402680872767));
#36867=CARTESIAN_POINT('Ctrl Pts',(2.176303712113,1.,-0.0819402680872767));
#36868=CARTESIAN_POINT('Ctrl Pts',(2.17063357870952,-1.,-0.0849584620835374));
#36869=CARTESIAN_POINT('Ctrl Pts',(2.17063357870952,1.,-0.0849584620835374));
#36870=CARTESIAN_POINT('Ctrl Pts',(2.16495552645014,-1.,-0.0879381291386924));
#36871=CARTESIAN_POINT('Ctrl Pts',(2.16495552645014,1.,-0.0879381291386924));
#36872=CARTESIAN_POINT('Ctrl Pts',(2.15926961544516,-1.,-0.0908789888107267));
#36873=CARTESIAN_POINT('Ctrl Pts',(2.15926961544516,1.,-0.0908789888107267));
#36874=CARTESIAN_POINT('Ctrl Pts',(2.1535759397817,-1.,-0.0937807218867645));
#36875=CARTESIAN_POINT('Ctrl Pts',(2.1535759397817,1.,-0.0937807218867645));
#36876=CARTESIAN_POINT('Ctrl Pts',(2.14787463531795,-1.,-0.096642985230546));
#36877=CARTESIAN_POINT('Ctrl Pts',(2.14787463531795,1.,-0.096642985230546));
#36878=CARTESIAN_POINT('Ctrl Pts',(2.14216588396025,-1.,-0.0994654261990917));
#36879=CARTESIAN_POINT('Ctrl Pts',(2.14216588396025,1.,-0.0994654261990917));
#36880=CARTESIAN_POINT('Ctrl Pts',(2.13644992667165,-1.,-0.102247700556101));
#36881=CARTESIAN_POINT('Ctrl Pts',(2.13644992667165,1.,-0.102247700556101));
#36882=CARTESIAN_POINT('Ctrl Pts',(2.13072704887293,-1.,-0.10498947915274));
#36883=CARTESIAN_POINT('Ctrl Pts',(2.13072704887293,1.,-0.10498947915274));
#36884=CARTESIAN_POINT('Ctrl Pts',(2.12499752307,-1.,-0.10769043523109));
#36885=CARTESIAN_POINT('Ctrl Pts',(2.12499752307,1.,-0.10769043523109));
#36886=CARTESIAN_POINT('Ctrl Pts',(2.11926155590865,-1.,-0.110350236135025));
#36887=CARTESIAN_POINT('Ctrl Pts',(2.11926155590865,1.,-0.110350236135025));
#36888=CARTESIAN_POINT('Ctrl Pts',(2.11351924490306,-1.,-0.112968534419737));
#36889=CARTESIAN_POINT('Ctrl Pts',(2.11351924490306,1.,-0.112968534419737));
#36890=CARTESIAN_POINT('Ctrl Pts',(2.10777050261309,-1.,-0.115544957687927));
#36891=CARTESIAN_POINT('Ctrl Pts',(2.10777050261309,1.,-0.115544957687927));
#36892=CARTESIAN_POINT('Ctrl Pts',(2.102015121329,-1.,-0.118079107988356));
#36893=CARTESIAN_POINT('Ctrl Pts',(2.102015121329,1.,-0.118079107988356));
#36894=CARTESIAN_POINT('Ctrl Pts',(2.0962529286773,-1.,-0.120570567965122));
#36895=CARTESIAN_POINT('Ctrl Pts',(2.0962529286773,1.,-0.120570567965122));
#36896=CARTESIAN_POINT('Ctrl Pts',(2.09048392424825,-1.,-0.123018905621083));
#36897=CARTESIAN_POINT('Ctrl Pts',(2.09048392424825,1.,-0.123018905621083));
#36898=CARTESIAN_POINT('Ctrl Pts',(2.08470840653643,-1.,-0.125423679412062));
#36899=CARTESIAN_POINT('Ctrl Pts',(2.08470840653643,1.,-0.125423679412062));
#36900=CARTESIAN_POINT('Ctrl Pts',(2.07892715110987,-1.,-0.12778444527612));
#36901=CARTESIAN_POINT('Ctrl Pts',(2.07892715110987,1.,-0.12778444527612));
#36902=CARTESIAN_POINT('Ctrl Pts',(2.07314114713063,-1.,-0.130100748328404));
#36903=CARTESIAN_POINT('Ctrl Pts',(2.07314114713063,1.,-0.130100748328404));
#36904=CARTESIAN_POINT('Ctrl Pts',(2.06735123910326,-1.,-0.132372111547711));
#36905=CARTESIAN_POINT('Ctrl Pts',(2.06735123910326,1.,-0.132372111547711));
#36906=CARTESIAN_POINT('Ctrl Pts',(2.06155781517842,-1.,-0.134598026192106));
#36907=CARTESIAN_POINT('Ctrl Pts',(2.06155781517842,1.,-0.134598026192106));
#36908=CARTESIAN_POINT('Ctrl Pts',(2.05576044414264,-1.,-0.136777941218044));
#36909=CARTESIAN_POINT('Ctrl Pts',(2.05576044414264,1.,-0.136777941218044));
#36910=CARTESIAN_POINT('Ctrl Pts',(2.04995762001328,-1.,-0.138911255368966));
#36911=CARTESIAN_POINT('Ctrl Pts',(2.04995762001328,1.,-0.138911255368966));
#36912=CARTESIAN_POINT('Ctrl Pts',(2.04414757947916,-1.,-0.140997332152546));
#36913=CARTESIAN_POINT('Ctrl Pts',(2.04414757947916,1.,-0.140997332152546));
#36914=CARTESIAN_POINT('Ctrl Pts',(2.03832911025912,-1.,-0.143035515058209));
#36915=CARTESIAN_POINT('Ctrl Pts',(2.03832911025912,1.,-0.143035515058209));
#36916=CARTESIAN_POINT('Ctrl Pts',(2.03250223739942,-1.,-0.145025140186058));
#36917=CARTESIAN_POINT('Ctrl Pts',(2.03250223739942,1.,-0.145025140186058));
#36918=CARTESIAN_POINT('Ctrl Pts',(2.02666926182017,-1.,-0.146965557332583));
#36919=CARTESIAN_POINT('Ctrl Pts',(2.02666926182017,1.,-0.146965557332583));
#36920=CARTESIAN_POINT('Ctrl Pts',(2.02083464969894,-1.,-0.148856124775337));
#36921=CARTESIAN_POINT('Ctrl Pts',(2.02083464969894,1.,-0.148856124775337));
#36922=CARTESIAN_POINT('Ctrl Pts',(2.01500291940238,-1.,-0.150696157673078));
#36923=CARTESIAN_POINT('Ctrl Pts',(2.01500291940238,1.,-0.150696157673078));
#36924=CARTESIAN_POINT('Ctrl Pts',(2.00917680318424,-1.,-0.15248488362145));
#36925=CARTESIAN_POINT('Ctrl Pts',(2.00917680318424,1.,-0.15248488362145));
#36926=CARTESIAN_POINT('Ctrl Pts',(2.00335565310543,-1.,-0.154221403049722));
#36927=CARTESIAN_POINT('Ctrl Pts',(2.00335565310543,1.,-0.154221403049722));
#36928=CARTESIAN_POINT('Ctrl Pts',(1.99753284771497,-1.,-0.155904629548784));
#36929=CARTESIAN_POINT('Ctrl Pts',(1.99753284771497,1.,-0.155904629548784));
#36930=CARTESIAN_POINT('Ctrl Pts',(1.99169810931908,-1.,-0.157533331459227));
#36931=CARTESIAN_POINT('Ctrl Pts',(1.99169810931908,1.,-0.157533331459227));
#36932=CARTESIAN_POINT('Ctrl Pts',(1.98584238283292,-1.,-0.159106226437299));
#36933=CARTESIAN_POINT('Ctrl Pts',(1.98584238283292,1.,-0.159106226437299));
#36934=CARTESIAN_POINT('Ctrl Pts',(1.97996195437559,-1.,-0.160622060784611));
#36935=CARTESIAN_POINT('Ctrl Pts',(1.97996195437559,1.,-0.160622060784611));
#36936=CARTESIAN_POINT('Ctrl Pts',(1.97406280235188,-1.,-0.162079693556289));
#36937=CARTESIAN_POINT('Ctrl Pts',(1.97406280235188,1.,-0.162079693556289));
#36938=CARTESIAN_POINT('Ctrl Pts',(1.96816512677967,-1.,-0.163478185457734));
#36939=CARTESIAN_POINT('Ctrl Pts',(1.96816512677967,1.,-0.163478185457734));
#36940=CARTESIAN_POINT('Ctrl Pts',(1.96229379940136,-1.,-0.164816568920269));
#36941=CARTESIAN_POINT('Ctrl Pts',(1.96229379940136,1.,-0.164816568920269));
#36942=CARTESIAN_POINT('Ctrl Pts',(1.9564675971873,-1.,-0.166093592002813));
#36943=CARTESIAN_POINT('Ctrl Pts',(1.9564675971873,1.,-0.166093592002813));
#36944=CARTESIAN_POINT('Ctrl Pts',(1.95069027794294,-1.,-0.167307501784476));
#36945=CARTESIAN_POINT('Ctrl Pts',(1.95069027794294,1.,-0.167307501784476));
#36946=CARTESIAN_POINT('Ctrl Pts',(1.94493757756931,-1.,-0.168455741607556));
#36947=CARTESIAN_POINT('Ctrl Pts',(1.94493757756931,1.,-0.168455741607556));
#36948=CARTESIAN_POINT('Ctrl Pts',(1.93915639211581,-1.,-0.169534904817491));
#36949=CARTESIAN_POINT('Ctrl Pts',(1.93915639211581,1.,-0.169534904817491));
#36950=CARTESIAN_POINT('Ctrl Pts',(1.93329183155539,-1.,-0.170541253116202));
#36951=CARTESIAN_POINT('Ctrl Pts',(1.93329183155539,1.,-0.170541253116202));
#36952=CARTESIAN_POINT('Ctrl Pts',(1.92731093582036,-1.,-0.171471191532988));
#36953=CARTESIAN_POINT('Ctrl Pts',(1.92731093582036,1.,-0.171471191532988));
#36954=CARTESIAN_POINT('Ctrl Pts',(1.9212233439798,-1.,-0.172321621259514));
#36955=CARTESIAN_POINT('Ctrl Pts',(1.9212233439798,1.,-0.172321621259514));
#36956=CARTESIAN_POINT('Ctrl Pts',(1.91511429159527,-1.,-0.173090695383496));
#36957=CARTESIAN_POINT('Ctrl Pts',(1.91511429159527,1.,-0.173090695383496));
#36958=CARTESIAN_POINT('Ctrl Pts',(1.90911693975267,-1.,-0.173776635257817));
#36959=CARTESIAN_POINT('Ctrl Pts',(1.90911693975267,1.,-0.173776635257817));
#36960=CARTESIAN_POINT('Ctrl Pts',(1.90335253862834,-1.,-0.174375518661085));
#36961=CARTESIAN_POINT('Ctrl Pts',(1.90335253862834,1.,-0.174375518661085));
#36962=CARTESIAN_POINT('Ctrl Pts',(1.89788101117132,-1.,-0.174879405091263));
#36963=CARTESIAN_POINT('Ctrl Pts',(1.89788101117132,1.,-0.174879405091263));
#36964=CARTESIAN_POINT('Ctrl Pts',(1.892646301985,-1.,-0.175274276190844));
#36965=CARTESIAN_POINT('Ctrl Pts',(1.892646301985,1.,-0.175274276190844));
#36966=CARTESIAN_POINT('Ctrl Pts',(1.88742606273259,-1.,-0.175538155840648));
#36967=CARTESIAN_POINT('Ctrl Pts',(1.88742606273259,1.,-0.175538155840648));
#36968=CARTESIAN_POINT('Ctrl Pts',(1.88188663145367,-1.,-0.175644148889699));
#36969=CARTESIAN_POINT('Ctrl Pts',(1.88188663145367,1.,-0.175644148889699));
#36970=CARTESIAN_POINT('Ctrl Pts',(1.87563767773588,-1.,-0.175563480746485));
#36971=CARTESIAN_POINT('Ctrl Pts',(1.87563767773588,1.,-0.175563480746485));
#36972=CARTESIAN_POINT('Ctrl Pts',(1.86828349694799,-1.,-0.175268337590758));
#36973=CARTESIAN_POINT('Ctrl Pts',(1.86828349694799,1.,-0.175268337590758));
#36974=CARTESIAN_POINT('Ctrl Pts',(1.85948367088837,-1.,-0.17473525927603));
#36975=CARTESIAN_POINT('Ctrl Pts',(1.85948367088837,1.,-0.17473525927603));
#36976=CARTESIAN_POINT('Ctrl Pts',(1.8489811319852,-1.,-0.173946627587732));
#36977=CARTESIAN_POINT('Ctrl Pts',(1.8489811319852,1.,-0.173946627587732));
#36978=CARTESIAN_POINT('Ctrl Pts',(1.83658380527692,-1.,-0.1728894428919));
#36979=CARTESIAN_POINT('Ctrl Pts',(1.83658380527692,1.,-0.1728894428919));
#36980=CARTESIAN_POINT('Ctrl Pts',(1.82215766811545,-1.,-0.171554770204119));
#36981=CARTESIAN_POINT('Ctrl Pts',(1.82215766811545,1.,-0.171554770204119));
#36982=CARTESIAN_POINT('Ctrl Pts',(1.80561530629706,-1.,-0.169936923904608));
#36983=CARTESIAN_POINT('Ctrl Pts',(1.80561530629706,1.,-0.169936923904608));
#36984=CARTESIAN_POINT('Ctrl Pts',(1.7869064998507,-1.,-0.168032772805197));
#36985=CARTESIAN_POINT('Ctrl Pts',(1.7869064998507,1.,-0.168032772805197));
#36986=CARTESIAN_POINT('Ctrl Pts',(1.77018771684844,-1.,-0.1662793551464));
#36987=CARTESIAN_POINT('Ctrl Pts',(1.77018771684844,1.,-0.1662793551464));
#36988=CARTESIAN_POINT('Ctrl Pts',(1.75666056638427,-1.,-0.164834765707159));
#36989=CARTESIAN_POINT('Ctrl Pts',(1.75666056638427,1.,-0.164834765707159));
#36990=CARTESIAN_POINT('Ctrl Pts',(1.7472034950333,-1.,-0.163814161002002));
#36991=CARTESIAN_POINT('Ctrl Pts',(1.7472034950333,1.,-0.163814161002002));
#36992=CARTESIAN_POINT('Ctrl Pts',(1.74236521665491,-1.,-0.163289472382896));
#36993=CARTESIAN_POINT('Ctrl Pts',(1.74236521665491,1.,-0.163289472382896));
#36994=CARTESIAN_POINT('',(2.19890268624765,1.,-0.0694764450219582));
#36995=CARTESIAN_POINT('Ctrl Pts',(2.19890268624765,1.,-0.0694764450219582));
#36996=CARTESIAN_POINT('Ctrl Pts',(2.19777582085423,1.,-0.0701143536325491));
#36997=CARTESIAN_POINT('Ctrl Pts',(2.19552129484002,1.,-0.0713863779526155));
#36998=CARTESIAN_POINT('Ctrl Pts',(2.19213712013662,1.,-0.0732830357306726));
#36999=CARTESIAN_POINT('Ctrl Pts',(2.1876201139953,1.,-0.0757891465836149));
#37000=CARTESIAN_POINT('Ctrl Pts',(2.18196589448887,1.,-0.0788837727685244));
#37001=CARTESIAN_POINT('Ctrl Pts',(2.176303712113,1.,-0.0819402680872767));
#37002=CARTESIAN_POINT('Ctrl Pts',(2.17063357870952,1.,-0.0849584620835374));
#37003=CARTESIAN_POINT('Ctrl Pts',(2.16495552645014,1.,-0.0879381291386924));
#37004=CARTESIAN_POINT('Ctrl Pts',(2.15926961544516,1.,-0.0908789888107267));
#37005=CARTESIAN_POINT('Ctrl Pts',(2.1535759397817,1.,-0.0937807218867645));
#37006=CARTESIAN_POINT('Ctrl Pts',(2.14787463531795,1.,-0.096642985230546));
#37007=CARTESIAN_POINT('Ctrl Pts',(2.14216588396025,1.,-0.0994654261990917));
#37008=CARTESIAN_POINT('Ctrl Pts',(2.13644992667165,1.,-0.102247700556101));
#37009=CARTESIAN_POINT('Ctrl Pts',(2.13072704887293,1.,-0.10498947915274));
#37010=CARTESIAN_POINT('Ctrl Pts',(2.12499752307,1.,-0.10769043523109));
#37011=CARTESIAN_POINT('Ctrl Pts',(2.11926155590865,1.,-0.110350236135025));
#37012=CARTESIAN_POINT('Ctrl Pts',(2.11351924490306,1.,-0.112968534419737));
#37013=CARTESIAN_POINT('Ctrl Pts',(2.10777050261309,1.,-0.115544957687927));
#37014=CARTESIAN_POINT('Ctrl Pts',(2.102015121329,1.,-0.118079107988356));
#37015=CARTESIAN_POINT('Ctrl Pts',(2.0962529286773,1.,-0.120570567965122));
#37016=CARTESIAN_POINT('Ctrl Pts',(2.09048392424825,1.,-0.123018905621083));
#37017=CARTESIAN_POINT('Ctrl Pts',(2.08470840653643,1.,-0.125423679412062));
#37018=CARTESIAN_POINT('Ctrl Pts',(2.07892715110987,1.,-0.12778444527612));
#37019=CARTESIAN_POINT('Ctrl Pts',(2.07314114713063,1.,-0.130100748328404));
#37020=CARTESIAN_POINT('Ctrl Pts',(2.06735123910326,1.,-0.132372111547711));
#37021=CARTESIAN_POINT('Ctrl Pts',(2.06155781517842,1.,-0.134598026192106));
#37022=CARTESIAN_POINT('Ctrl Pts',(2.05576044414264,1.,-0.136777941218044));
#37023=CARTESIAN_POINT('Ctrl Pts',(2.04995762001328,1.,-0.138911255368966));
#37024=CARTESIAN_POINT('Ctrl Pts',(2.04414757947916,1.,-0.140997332152546));
#37025=CARTESIAN_POINT('Ctrl Pts',(2.03832911025912,1.,-0.143035515058209));
#37026=CARTESIAN_POINT('Ctrl Pts',(2.03250223739942,1.,-0.145025140186058));
#37027=CARTESIAN_POINT('Ctrl Pts',(2.02666926182017,1.,-0.146965557332583));
#37028=CARTESIAN_POINT('Ctrl Pts',(2.02083464969894,1.,-0.148856124775337));
#37029=CARTESIAN_POINT('Ctrl Pts',(2.01500291940238,1.,-0.150696157673078));
#37030=CARTESIAN_POINT('Ctrl Pts',(2.00917680318424,1.,-0.15248488362145));
#37031=CARTESIAN_POINT('Ctrl Pts',(2.00335565310543,1.,-0.154221403049722));
#37032=CARTESIAN_POINT('Ctrl Pts',(1.99753284771497,1.,-0.155904629548784));
#37033=CARTESIAN_POINT('Ctrl Pts',(1.99169810931908,1.,-0.157533331459227));
#37034=CARTESIAN_POINT('Ctrl Pts',(1.98584238283292,1.,-0.159106226437299));
#37035=CARTESIAN_POINT('Ctrl Pts',(1.97996195437559,1.,-0.160622060784611));
#37036=CARTESIAN_POINT('Ctrl Pts',(1.97406280235188,1.,-0.162079693556289));
#37037=CARTESIAN_POINT('Ctrl Pts',(1.96816512677967,1.,-0.163478185457734));
#37038=CARTESIAN_POINT('Ctrl Pts',(1.96229379940136,1.,-0.164816568920269));
#37039=CARTESIAN_POINT('Ctrl Pts',(1.9564675971873,1.,-0.166093592002813));
#37040=CARTESIAN_POINT('Ctrl Pts',(1.95069027794294,1.,-0.167307501784476));
#37041=CARTESIAN_POINT('Ctrl Pts',(1.94493757756931,1.,-0.168455741607556));
#37042=CARTESIAN_POINT('Ctrl Pts',(1.93915639211581,1.,-0.169534904817491));
#37043=CARTESIAN_POINT('Ctrl Pts',(1.93329183155539,1.,-0.170541253116202));
#37044=CARTESIAN_POINT('Ctrl Pts',(1.92731093582036,1.,-0.171471191532988));
#37045=CARTESIAN_POINT('Ctrl Pts',(1.9212233439798,1.,-0.172321621259514));
#37046=CARTESIAN_POINT('Ctrl Pts',(1.91511429159527,1.,-0.173090695383496));
#37047=CARTESIAN_POINT('Ctrl Pts',(1.90911693975267,1.,-0.173776635257817));
#37048=CARTESIAN_POINT('Ctrl Pts',(1.90335253862834,1.,-0.174375518661085));
#37049=CARTESIAN_POINT('Ctrl Pts',(1.89788101117132,1.,-0.174879405091263));
#37050=CARTESIAN_POINT('Ctrl Pts',(1.892646301985,1.,-0.175274276190844));
#37051=CARTESIAN_POINT('Ctrl Pts',(1.88742606273259,1.,-0.175538155840648));
#37052=CARTESIAN_POINT('Ctrl Pts',(1.88188663145367,1.,-0.175644148889699));
#37053=CARTESIAN_POINT('Ctrl Pts',(1.87563767773588,1.,-0.175563480746485));
#37054=CARTESIAN_POINT('Ctrl Pts',(1.86828349694799,1.,-0.175268337590758));
#37055=CARTESIAN_POINT('Ctrl Pts',(1.85948367088837,1.,-0.17473525927603));
#37056=CARTESIAN_POINT('Ctrl Pts',(1.8489811319852,1.,-0.173946627587732));
#37057=CARTESIAN_POINT('Ctrl Pts',(1.83658380527692,1.,-0.1728894428919));
#37058=CARTESIAN_POINT('Ctrl Pts',(1.82215766811545,1.,-0.171554770204119));
#37059=CARTESIAN_POINT('Ctrl Pts',(1.80561530629706,1.,-0.169936923904608));
#37060=CARTESIAN_POINT('Ctrl Pts',(1.7869064998507,1.,-0.168032772805197));
#37061=CARTESIAN_POINT('Ctrl Pts',(1.77018771684844,1.,-0.1662793551464));
#37062=CARTESIAN_POINT('Ctrl Pts',(1.75666056638427,1.,-0.164834765707159));
#37063=CARTESIAN_POINT('Ctrl Pts',(1.7472034950333,1.,-0.163814161002002));
#37064=CARTESIAN_POINT('Ctrl Pts',(1.74236521665491,1.,-0.163289472382896));
#37065=CARTESIAN_POINT('',(2.19890268624765,0.,-0.0694764450219582));
#37066=CARTESIAN_POINT('Origin',(2.19890268624765,0.,0.0694764450219582));
#37067=CARTESIAN_POINT('',(2.19890268624765,1.,0.0694764450219582));
#37068=CARTESIAN_POINT('',(2.19890268624765,1.,-0.0694764450219582));
#37069=CARTESIAN_POINT('',(2.19890268624765,0.,0.0694764450219582));
#37070=CARTESIAN_POINT('Ctrl Pts',(1.74236521665491,-1.,0.163289472382896));
#37071=CARTESIAN_POINT('Ctrl Pts',(1.74236521665491,1.,0.163289472382896));
#37072=CARTESIAN_POINT('Ctrl Pts',(1.74720349503904,-1.,0.163814161002474));
#37073=CARTESIAN_POINT('Ctrl Pts',(1.74720349503904,1.,0.163814161002474));
#37074=CARTESIAN_POINT('Ctrl Pts',(1.75666056640041,-1.,0.164834765708484));
#37075=CARTESIAN_POINT('Ctrl Pts',(1.75666056640041,1.,0.164834765708484));
#37076=CARTESIAN_POINT('Ctrl Pts',(1.77018771687692,-1.,0.166279355148738));
#37077=CARTESIAN_POINT('Ctrl Pts',(1.77018771687692,1.,0.166279355148738));
#37078=CARTESIAN_POINT('Ctrl Pts',(1.78690649988931,-1.,0.16803277280837));
#37079=CARTESIAN_POINT('Ctrl Pts',(1.78690649988931,1.,0.16803277280837));
#37080=CARTESIAN_POINT('Ctrl Pts',(1.80561530633924,-1.,0.169936923908078));
#37081=CARTESIAN_POINT('Ctrl Pts',(1.80561530633924,1.,0.169936923908078));
#37082=CARTESIAN_POINT('Ctrl Pts',(1.82215766815414,-1.,0.171554770207306));
#37083=CARTESIAN_POINT('Ctrl Pts',(1.82215766815414,1.,0.171554770207306));
#37084=CARTESIAN_POINT('Ctrl Pts',(1.83658380530747,-1.,0.17288944289442));
#37085=CARTESIAN_POINT('Ctrl Pts',(1.83658380530747,1.,0.17288944289442));
#37086=CARTESIAN_POINT('Ctrl Pts',(1.84898113200543,-1.,0.173946627589401));
#37087=CARTESIAN_POINT('Ctrl Pts',(1.84898113200543,1.,0.173946627589401));
#37088=CARTESIAN_POINT('Ctrl Pts',(1.85948367089838,-1.,0.174735259276856));
#37089=CARTESIAN_POINT('Ctrl Pts',(1.85948367089838,1.,0.174735259276856));
#37090=CARTESIAN_POINT('Ctrl Pts',(1.86828349694972,-1.,0.1752683375909));
#37091=CARTESIAN_POINT('Ctrl Pts',(1.86828349694972,1.,0.1752683375909));
#37092=CARTESIAN_POINT('Ctrl Pts',(1.87563767773249,-1.,0.175563480746205));
#37093=CARTESIAN_POINT('Ctrl Pts',(1.87563767773249,1.,0.175563480746205));
#37094=CARTESIAN_POINT('Ctrl Pts',(1.88188663144846,-1.,0.175644148889271));
#37095=CARTESIAN_POINT('Ctrl Pts',(1.88188663144846,1.,0.175644148889271));
#37096=CARTESIAN_POINT('Ctrl Pts',(1.88742606272818,-1.,0.175538155840286));
#37097=CARTESIAN_POINT('Ctrl Pts',(1.88742606272818,1.,0.175538155840286));
#37098=CARTESIAN_POINT('Ctrl Pts',(1.89264630198279,-1.,0.175274276190664));
#37099=CARTESIAN_POINT('Ctrl Pts',(1.89264630198279,1.,0.175274276190664));
#37100=CARTESIAN_POINT('Ctrl Pts',(1.89788101117148,-1.,0.174879405091277));
#37101=CARTESIAN_POINT('Ctrl Pts',(1.89788101117148,1.,0.174879405091277));
#37102=CARTESIAN_POINT('Ctrl Pts',(1.90335253863003,-1.,0.174375518661222));
#37103=CARTESIAN_POINT('Ctrl Pts',(1.90335253863003,1.,0.174375518661222));
#37104=CARTESIAN_POINT('Ctrl Pts',(1.90911693975475,-1.,0.173776635257983));
#37105=CARTESIAN_POINT('Ctrl Pts',(1.90911693975475,1.,0.173776635257983));
#37106=CARTESIAN_POINT('Ctrl Pts',(1.91511429159681,-1.,0.173090695383619));
#37107=CARTESIAN_POINT('Ctrl Pts',(1.91511429159681,1.,0.173090695383619));
#37108=CARTESIAN_POINT('Ctrl Pts',(1.92122334398034,-1.,0.172321621259556));
#37109=CARTESIAN_POINT('Ctrl Pts',(1.92122334398034,1.,0.172321621259556));
#37110=CARTESIAN_POINT('Ctrl Pts',(1.92731093582,-1.,0.17147119153296));
#37111=CARTESIAN_POINT('Ctrl Pts',(1.92731093582,1.,0.17147119153296));
#37112=CARTESIAN_POINT('Ctrl Pts',(1.93329183155455,-1.,0.170541253116136));
#37113=CARTESIAN_POINT('Ctrl Pts',(1.93329183155455,1.,0.170541253116136));
#37114=CARTESIAN_POINT('Ctrl Pts',(1.93915639211497,-1.,0.169534904817425));
#37115=CARTESIAN_POINT('Ctrl Pts',(1.93915639211497,1.,0.169534904817425));
#37116=CARTESIAN_POINT('Ctrl Pts',(1.94493757756879,-1.,0.168455741607515));
#37117=CARTESIAN_POINT('Ctrl Pts',(1.94493757756879,1.,0.168455741607515));
#37118=CARTESIAN_POINT('Ctrl Pts',(1.95069027794286,-1.,0.167307501784469));
#37119=CARTESIAN_POINT('Ctrl Pts',(1.95069027794286,1.,0.167307501784469));
#37120=CARTESIAN_POINT('Ctrl Pts',(1.95646759718755,-1.,0.166093592002832));
#37121=CARTESIAN_POINT('Ctrl Pts',(1.95646759718755,1.,0.166093592002832));
#37122=CARTESIAN_POINT('Ctrl Pts',(1.96229379940174,-1.,0.1648165689203));
#37123=CARTESIAN_POINT('Ctrl Pts',(1.96229379940174,1.,0.1648165689203));
#37124=CARTESIAN_POINT('Ctrl Pts',(1.96816512678,-1.,0.16347818545776));
#37125=CARTESIAN_POINT('Ctrl Pts',(1.96816512678,1.,0.16347818545776));
#37126=CARTESIAN_POINT('Ctrl Pts',(1.97406280235204,-1.,0.162079693556302));
#37127=CARTESIAN_POINT('Ctrl Pts',(1.97406280235204,1.,0.162079693556302));
#37128=CARTESIAN_POINT('Ctrl Pts',(1.97996195437557,-1.,0.16062206078461));
#37129=CARTESIAN_POINT('Ctrl Pts',(1.97996195437557,1.,0.16062206078461));
#37130=CARTESIAN_POINT('Ctrl Pts',(1.98584238283279,-1.,0.159106226437288));
#37131=CARTESIAN_POINT('Ctrl Pts',(1.98584238283279,1.,0.159106226437288));
#37132=CARTESIAN_POINT('Ctrl Pts',(1.99169810931893,-1.,0.157533331459215));
#37133=CARTESIAN_POINT('Ctrl Pts',(1.99169810931893,1.,0.157533331459215));
#37134=CARTESIAN_POINT('Ctrl Pts',(1.99753284771487,-1.,0.155904629548774));
#37135=CARTESIAN_POINT('Ctrl Pts',(1.99753284771487,1.,0.155904629548774));
#37136=CARTESIAN_POINT('Ctrl Pts',(2.00335565310539,-1.,0.154221403049719));
#37137=CARTESIAN_POINT('Ctrl Pts',(2.00335565310539,1.,0.154221403049719));
#37138=CARTESIAN_POINT('Ctrl Pts',(2.00917680318426,-1.,0.152484883621452));
#37139=CARTESIAN_POINT('Ctrl Pts',(2.00917680318426,1.,0.152484883621452));
#37140=CARTESIAN_POINT('Ctrl Pts',(2.01500291940243,-1.,0.150696157673084));
#37141=CARTESIAN_POINT('Ctrl Pts',(2.01500291940243,1.,0.150696157673084));
#37142=CARTESIAN_POINT('Ctrl Pts',(2.02083464969897,-1.,0.148856124775342));
#37143=CARTESIAN_POINT('Ctrl Pts',(2.02083464969897,1.,0.148856124775342));
#37144=CARTESIAN_POINT('Ctrl Pts',(2.02666926182017,-1.,0.146965557332586));
#37145=CARTESIAN_POINT('Ctrl Pts',(2.02666926182017,1.,0.146965557332586));
#37146=CARTESIAN_POINT('Ctrl Pts',(2.03250223739941,-1.,0.145025140186058));
#37147=CARTESIAN_POINT('Ctrl Pts',(2.03250223739941,1.,0.145025140186058));
#37148=CARTESIAN_POINT('Ctrl Pts',(2.03832911025913,-1.,0.143035515058208));
#37149=CARTESIAN_POINT('Ctrl Pts',(2.03832911025913,1.,0.143035515058208));
#37150=CARTESIAN_POINT('Ctrl Pts',(2.04414757947919,-1.,0.140997332152545));
#37151=CARTESIAN_POINT('Ctrl Pts',(2.04414757947919,1.,0.140997332152545));
#37152=CARTESIAN_POINT('Ctrl Pts',(2.04995762001333,-1.,0.138911255368966));
#37153=CARTESIAN_POINT('Ctrl Pts',(2.04995762001333,1.,0.138911255368966));
#37154=CARTESIAN_POINT('Ctrl Pts',(2.0557604441427,-1.,0.136777941218044));
#37155=CARTESIAN_POINT('Ctrl Pts',(2.0557604441427,1.,0.136777941218044));
#37156=CARTESIAN_POINT('Ctrl Pts',(2.06155781517844,-1.,0.134598026192107));
#37157=CARTESIAN_POINT('Ctrl Pts',(2.06155781517844,1.,0.134598026192107));
#37158=CARTESIAN_POINT('Ctrl Pts',(2.06735123910319,-1.,0.132372111547709));
#37159=CARTESIAN_POINT('Ctrl Pts',(2.06735123910319,1.,0.132372111547709));
#37160=CARTESIAN_POINT('Ctrl Pts',(2.07314114713047,-1.,0.1301007483284));
#37161=CARTESIAN_POINT('Ctrl Pts',(2.07314114713047,1.,0.1301007483284));
#37162=CARTESIAN_POINT('Ctrl Pts',(2.07892715110967,-1.,0.127784445276116));
#37163=CARTESIAN_POINT('Ctrl Pts',(2.07892715110967,1.,0.127784445276116));
#37164=CARTESIAN_POINT('Ctrl Pts',(2.08470840653628,-1.,0.125423679412058));
#37165=CARTESIAN_POINT('Ctrl Pts',(2.08470840653628,1.,0.125423679412058));
#37166=CARTESIAN_POINT('Ctrl Pts',(2.09048392424826,-1.,0.123018905621083));
#37167=CARTESIAN_POINT('Ctrl Pts',(2.09048392424826,1.,0.123018905621083));
#37168=CARTESIAN_POINT('Ctrl Pts',(2.09625292867756,-1.,0.120570567965129));
#37169=CARTESIAN_POINT('Ctrl Pts',(2.09625292867756,1.,0.120570567965129));
#37170=CARTESIAN_POINT('Ctrl Pts',(2.10201512132945,-1.,0.118079107988368));
#37171=CARTESIAN_POINT('Ctrl Pts',(2.10201512132945,1.,0.118079107988368));
#37172=CARTESIAN_POINT('Ctrl Pts',(2.10777050261359,-1.,0.11554495768794));
#37173=CARTESIAN_POINT('Ctrl Pts',(2.10777050261359,1.,0.11554495768794));
#37174=CARTESIAN_POINT('Ctrl Pts',(2.11351924490335,-1.,0.112968534419746));
#37175=CARTESIAN_POINT('Ctrl Pts',(2.11351924490335,1.,0.112968534419746));
#37176=CARTESIAN_POINT('Ctrl Pts',(2.11926155590849,-1.,0.11035023613502));
#37177=CARTESIAN_POINT('Ctrl Pts',(2.11926155590849,1.,0.11035023613502));
#37178=CARTESIAN_POINT('Ctrl Pts',(2.12499752306927,-1.,0.107690435231068));
#37179=CARTESIAN_POINT('Ctrl Pts',(2.12499752306927,1.,0.107690435231068));
#37180=CARTESIAN_POINT('Ctrl Pts',(2.1307270488718,-1.,0.104989479152703));
#37181=CARTESIAN_POINT('Ctrl Pts',(2.1307270488718,1.,0.104989479152703));
#37182=CARTESIAN_POINT('Ctrl Pts',(2.13644992667052,-1.,0.102247700556063));
#37183=CARTESIAN_POINT('Ctrl Pts',(2.13644992667052,1.,0.102247700556063));
#37184=CARTESIAN_POINT('Ctrl Pts',(2.14216588395974,-1.,0.0994654261990741));
#37185=CARTESIAN_POINT('Ctrl Pts',(2.14216588395974,1.,0.0994654261990741));
#37186=CARTESIAN_POINT('Ctrl Pts',(2.14787463531864,-1.,0.0966429852305688));
#37187=CARTESIAN_POINT('Ctrl Pts',(2.14787463531864,1.,0.0966429852305688));
#37188=CARTESIAN_POINT('Ctrl Pts',(2.15357593978377,-1.,0.0937807218868344));
#37189=CARTESIAN_POINT('Ctrl Pts',(2.15357593978377,1.,0.0937807218868344));
#37190=CARTESIAN_POINT('Ctrl Pts',(2.15926961544808,-1.,0.0908789888108265));
#37191=CARTESIAN_POINT('Ctrl Pts',(2.15926961544808,1.,0.0908789888108265));
#37192=CARTESIAN_POINT('Ctrl Pts',(2.16495552645275,-1.,0.0879381291387821));
#37193=CARTESIAN_POINT('Ctrl Pts',(2.16495552645275,1.,0.0879381291387821));
#37194=CARTESIAN_POINT('Ctrl Pts',(2.17063357871031,-1.,0.0849584620835642));
#37195=CARTESIAN_POINT('Ctrl Pts',(2.17063357871031,1.,0.0849584620835642));
#37196=CARTESIAN_POINT('Ctrl Pts',(2.1763037121106,-1.,0.0819402680871938));
#37197=CARTESIAN_POINT('Ctrl Pts',(2.1763037121106,1.,0.0819402680871938));
#37198=CARTESIAN_POINT('Ctrl Pts',(2.18196589448304,-1.,0.0788837727683226));
#37199=CARTESIAN_POINT('Ctrl Pts',(2.18196589448304,1.,0.0788837727683226));
#37200=CARTESIAN_POINT('Ctrl Pts',(2.1876201139874,-1.,0.075789146583341));
#37201=CARTESIAN_POINT('Ctrl Pts',(2.1876201139874,1.,0.075789146583341));
#37202=CARTESIAN_POINT('Ctrl Pts',(2.19213712012956,-1.,0.0732830357304275));
#37203=CARTESIAN_POINT('Ctrl Pts',(2.19213712012956,1.,0.0732830357304275));
#37204=CARTESIAN_POINT('Ctrl Pts',(2.19552129483562,-1.,0.0713863779524626));
#37205=CARTESIAN_POINT('Ctrl Pts',(2.19552129483562,1.,0.0713863779524626));
#37206=CARTESIAN_POINT('Ctrl Pts',(2.19777582085261,-1.,0.0701143536324925));
#37207=CARTESIAN_POINT('Ctrl Pts',(2.19777582085261,1.,0.0701143536324925));
#37208=CARTESIAN_POINT('Ctrl Pts',(2.19890268624765,-1.,0.0694764450219582));
#37209=CARTESIAN_POINT('Ctrl Pts',(2.19890268624765,1.,0.0694764450219582));
#37210=CARTESIAN_POINT('',(1.74236521665491,1.,0.163289472382896));
#37211=CARTESIAN_POINT('Ctrl Pts',(1.74236521665491,1.,0.163289472382896));
#37212=CARTESIAN_POINT('Ctrl Pts',(1.74720349503904,1.,0.163814161002474));
#37213=CARTESIAN_POINT('Ctrl Pts',(1.75666056640041,1.,0.164834765708484));
#37214=CARTESIAN_POINT('Ctrl Pts',(1.77018771687692,1.,0.166279355148738));
#37215=CARTESIAN_POINT('Ctrl Pts',(1.78690649988931,1.,0.16803277280837));
#37216=CARTESIAN_POINT('Ctrl Pts',(1.80561530633924,1.,0.169936923908078));
#37217=CARTESIAN_POINT('Ctrl Pts',(1.82215766815414,1.,0.171554770207306));
#37218=CARTESIAN_POINT('Ctrl Pts',(1.83658380530747,1.,0.17288944289442));
#37219=CARTESIAN_POINT('Ctrl Pts',(1.84898113200543,1.,0.173946627589401));
#37220=CARTESIAN_POINT('Ctrl Pts',(1.85948367089838,1.,0.174735259276856));
#37221=CARTESIAN_POINT('Ctrl Pts',(1.86828349694972,1.,0.1752683375909));
#37222=CARTESIAN_POINT('Ctrl Pts',(1.87563767773249,1.,0.175563480746205));
#37223=CARTESIAN_POINT('Ctrl Pts',(1.88188663144846,1.,0.175644148889271));
#37224=CARTESIAN_POINT('Ctrl Pts',(1.88742606272818,1.,0.175538155840286));
#37225=CARTESIAN_POINT('Ctrl Pts',(1.89264630198279,1.,0.175274276190664));
#37226=CARTESIAN_POINT('Ctrl Pts',(1.89788101117148,1.,0.174879405091277));
#37227=CARTESIAN_POINT('Ctrl Pts',(1.90335253863003,1.,0.174375518661222));
#37228=CARTESIAN_POINT('Ctrl Pts',(1.90911693975475,1.,0.173776635257983));
#37229=CARTESIAN_POINT('Ctrl Pts',(1.91511429159681,1.,0.173090695383619));
#37230=CARTESIAN_POINT('Ctrl Pts',(1.92122334398034,1.,0.172321621259556));
#37231=CARTESIAN_POINT('Ctrl Pts',(1.92731093582,1.,0.17147119153296));
#37232=CARTESIAN_POINT('Ctrl Pts',(1.93329183155455,1.,0.170541253116136));
#37233=CARTESIAN_POINT('Ctrl Pts',(1.93915639211497,1.,0.169534904817425));
#37234=CARTESIAN_POINT('Ctrl Pts',(1.94493757756879,1.,0.168455741607515));
#37235=CARTESIAN_POINT('Ctrl Pts',(1.95069027794286,1.,0.167307501784469));
#37236=CARTESIAN_POINT('Ctrl Pts',(1.95646759718755,1.,0.166093592002832));
#37237=CARTESIAN_POINT('Ctrl Pts',(1.96229379940174,1.,0.1648165689203));
#37238=CARTESIAN_POINT('Ctrl Pts',(1.96816512678,1.,0.16347818545776));
#37239=CARTESIAN_POINT('Ctrl Pts',(1.97406280235204,1.,0.162079693556302));
#37240=CARTESIAN_POINT('Ctrl Pts',(1.97996195437557,1.,0.16062206078461));
#37241=CARTESIAN_POINT('Ctrl Pts',(1.98584238283279,1.,0.159106226437288));
#37242=CARTESIAN_POINT('Ctrl Pts',(1.99169810931893,1.,0.157533331459215));
#37243=CARTESIAN_POINT('Ctrl Pts',(1.99753284771487,1.,0.155904629548774));
#37244=CARTESIAN_POINT('Ctrl Pts',(2.00335565310539,1.,0.154221403049719));
#37245=CARTESIAN_POINT('Ctrl Pts',(2.00917680318426,1.,0.152484883621452));
#37246=CARTESIAN_POINT('Ctrl Pts',(2.01500291940243,1.,0.150696157673084));
#37247=CARTESIAN_POINT('Ctrl Pts',(2.02083464969897,1.,0.148856124775342));
#37248=CARTESIAN_POINT('Ctrl Pts',(2.02666926182017,1.,0.146965557332586));
#37249=CARTESIAN_POINT('Ctrl Pts',(2.03250223739941,1.,0.145025140186058));
#37250=CARTESIAN_POINT('Ctrl Pts',(2.03832911025913,1.,0.143035515058208));
#37251=CARTESIAN_POINT('Ctrl Pts',(2.04414757947919,1.,0.140997332152545));
#37252=CARTESIAN_POINT('Ctrl Pts',(2.04995762001333,1.,0.138911255368966));
#37253=CARTESIAN_POINT('Ctrl Pts',(2.0557604441427,1.,0.136777941218044));
#37254=CARTESIAN_POINT('Ctrl Pts',(2.06155781517844,1.,0.134598026192107));
#37255=CARTESIAN_POINT('Ctrl Pts',(2.06735123910319,1.,0.132372111547709));
#37256=CARTESIAN_POINT('Ctrl Pts',(2.07314114713047,1.,0.1301007483284));
#37257=CARTESIAN_POINT('Ctrl Pts',(2.07892715110967,1.,0.127784445276116));
#37258=CARTESIAN_POINT('Ctrl Pts',(2.08470840653628,1.,0.125423679412058));
#37259=CARTESIAN_POINT('Ctrl Pts',(2.09048392424826,1.,0.123018905621083));
#37260=CARTESIAN_POINT('Ctrl Pts',(2.09625292867756,1.,0.120570567965129));
#37261=CARTESIAN_POINT('Ctrl Pts',(2.10201512132945,1.,0.118079107988368));
#37262=CARTESIAN_POINT('Ctrl Pts',(2.10777050261359,1.,0.11554495768794));
#37263=CARTESIAN_POINT('Ctrl Pts',(2.11351924490335,1.,0.112968534419746));
#37264=CARTESIAN_POINT('Ctrl Pts',(2.11926155590849,1.,0.11035023613502));
#37265=CARTESIAN_POINT('Ctrl Pts',(2.12499752306927,1.,0.107690435231068));
#37266=CARTESIAN_POINT('Ctrl Pts',(2.1307270488718,1.,0.104989479152703));
#37267=CARTESIAN_POINT('Ctrl Pts',(2.13644992667052,1.,0.102247700556063));
#37268=CARTESIAN_POINT('Ctrl Pts',(2.14216588395974,1.,0.0994654261990741));
#37269=CARTESIAN_POINT('Ctrl Pts',(2.14787463531864,1.,0.0966429852305688));
#37270=CARTESIAN_POINT('Ctrl Pts',(2.15357593978377,1.,0.0937807218868344));
#37271=CARTESIAN_POINT('Ctrl Pts',(2.15926961544808,1.,0.0908789888108265));
#37272=CARTESIAN_POINT('Ctrl Pts',(2.16495552645275,1.,0.0879381291387821));
#37273=CARTESIAN_POINT('Ctrl Pts',(2.17063357871031,1.,0.0849584620835642));
#37274=CARTESIAN_POINT('Ctrl Pts',(2.1763037121106,1.,0.0819402680871938));
#37275=CARTESIAN_POINT('Ctrl Pts',(2.18196589448304,1.,0.0788837727683226));
#37276=CARTESIAN_POINT('Ctrl Pts',(2.1876201139874,1.,0.075789146583341));
#37277=CARTESIAN_POINT('Ctrl Pts',(2.19213712012956,1.,0.0732830357304275));
#37278=CARTESIAN_POINT('Ctrl Pts',(2.19552129483562,1.,0.0713863779524626));
#37279=CARTESIAN_POINT('Ctrl Pts',(2.19777582085261,1.,0.0701143536324925));
#37280=CARTESIAN_POINT('Ctrl Pts',(2.19890268624765,1.,0.0694764450219582));
#37281=CARTESIAN_POINT('',(1.74236521665491,0.,0.163289472382896));
#37282=CARTESIAN_POINT('Origin',(0.,1.,0.));
#37283=CARTESIAN_POINT('Origin',(0.,1.,0.));
#37284=CARTESIAN_POINT('Origin',(0.,0.,0.));
#73279=UNCERTAINTY_MEASURE_WITH_UNIT(LENGTH_MEASURE(0.001),#73367,
'DISTANCE_ACCURACY_VALUE',
'Maximum model space distance between geometric entities at asserted c
onnectivities');
#73302=UNCERTAINTY_MEASURE_WITH_UNIT(LENGTH_MEASURE(0.001),#73367,
'DISTANCE_ACCURACY_VALUE',
'Maximum model space distance between geometric entities at asserted c
onnectivities');
#73343=(
GEOMETRIC_REPRESENTATION_CONTEXT(3)
GLOBAL_UNCERTAINTY_ASSIGNED_CONTEXT((#73279))
GLOBAL_UNIT_ASSIGNED_CONTEXT((#73367,#73369,#73370))
REPRESENTATION_CONTEXT('','3D')
);
#73366=(
GEOMETRIC_REPRESENTATION_CONTEXT(3)
GLOBAL_UNCERTAINTY_ASSIGNED_CONTEXT((#73302))
GLOBAL_UNIT_ASSIGNED_CONTEXT((#73367,#73369,#73370))
REPRESENTATION_CONTEXT('','3D')
);
#73367=(
LENGTH_UNIT()
NAMED_UNIT(*)
SI_UNIT(.CENTI.,.METRE.)
);
#73369=(
NAMED_UNIT(*)
PLANE_ANGLE_UNIT()
SI_UNIT($,.RADIAN.)
);
#73370=(
NAMED_UNIT(*)
SI_UNIT($,.STERADIAN.)
SOLID_ANGLE_UNIT()
);
#73411=SHAPE_DEFINITION_REPRESENTATION(#73544,#73647);
#73544=PRODUCT_DEFINITION_SHAPE('',$,#73711);
#73647=SHAPE_REPRESENTATION('',(#17844),#73343);
#73670=PRODUCT_DEFINITION_CONTEXT('part definition',#73861,'design');
#73711=PRODUCT_DEFINITION('Spur Gear - Module 2, 20 Teeth, 12 mm Bore',
'Spur Gear - Module 2, 20 Teeth, 12 mm Bore',#73774,#73670);
#73774=PRODUCT_DEFINITION_FORMATION('',$,#73903);
#73861=APPLICATION_CONTEXT(
'Core Data for Automotive Mechanical Design Process');
#73862=PRODUCT_CONTEXT('part definition',#73861,'mechanical');
#73903=PRODUCT('Spur Gear - Module 2, 20 Teeth, 12 mm Bore',
'Spur Gear - Module 2, 20 Teeth, 12 mm Bore',
'Spur Gear - Module 2, 20 Teeth, 12 mm Bore',(#73862));
#73996=COLOUR_RGB('Off White',0.89,0.88,0.83);
#73997=FILL_AREA_STYLE_COLOUR('',#73996);
#73998=FILL_AREA_STYLE('',(#73997));
#73999=SURFACE_STYLE_FILL_AREA(#73998);
#74000=SURFACE_SIDE_STYLE('',(#73999));
#74001=SURFACE_STYLE_USAGE(.BOTH.,#74000);
#74002=PRESENTATION_STYLE_ASSIGNMENT((#74001));
ENDSEC;
END-ISO-10303-21;
